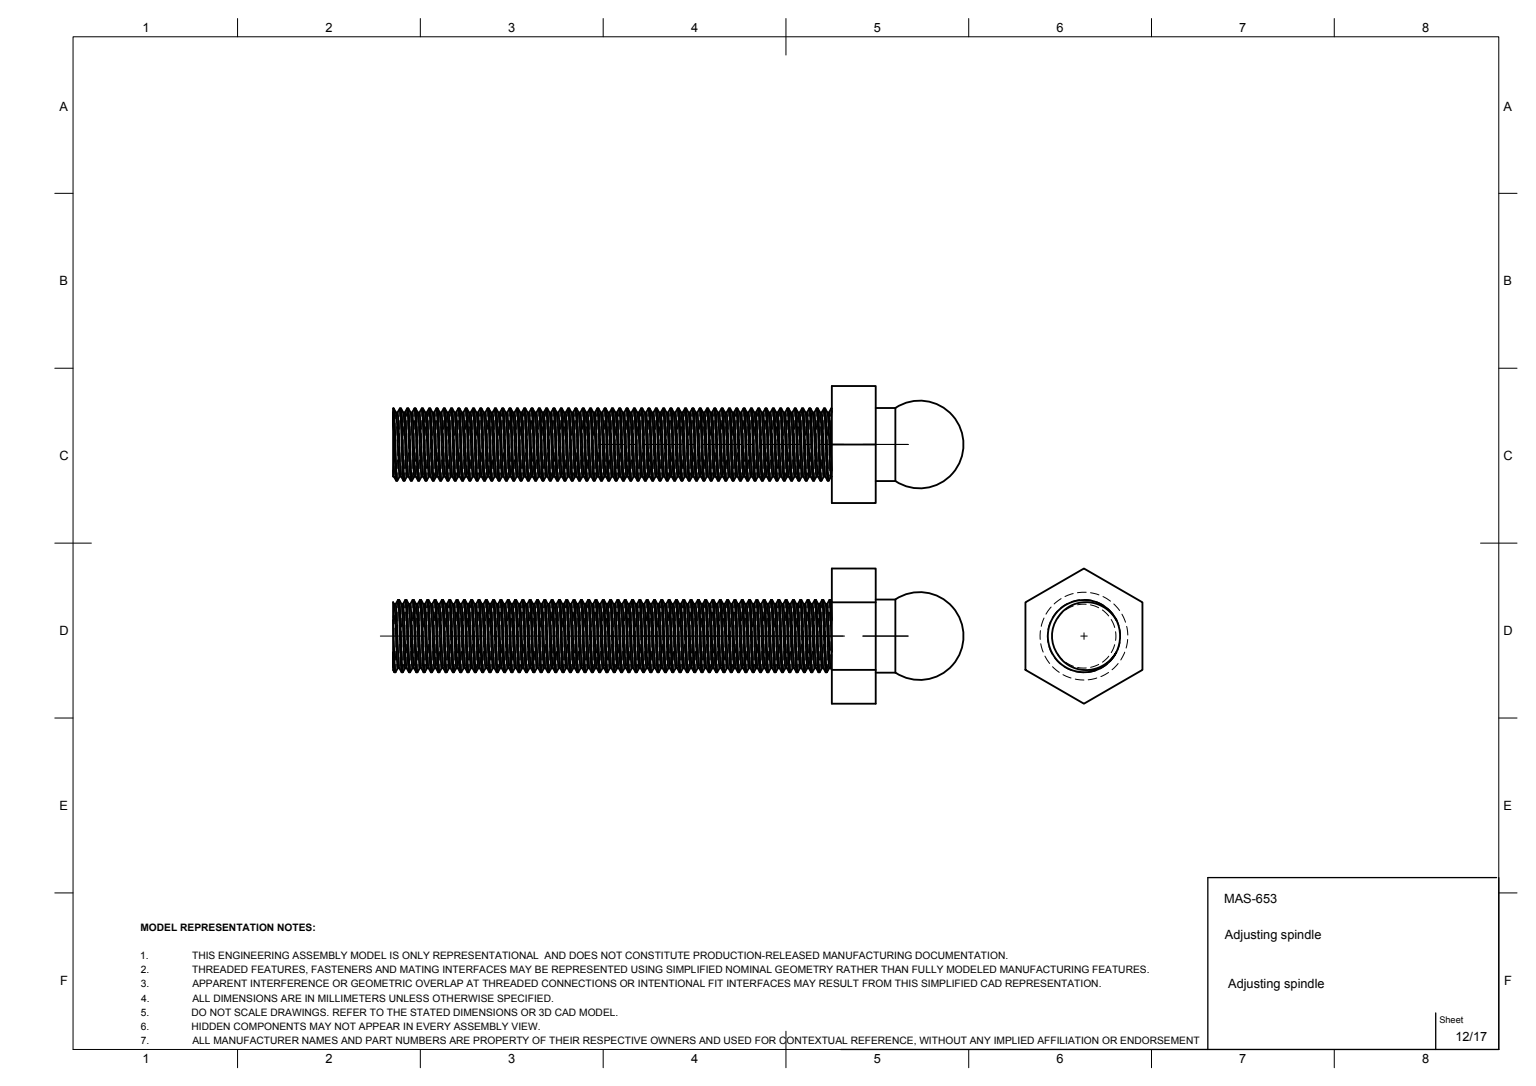
ISO-10303-21;
HEADER;
/* Generated by software containing ST-Developer
 * from STEP Tools, Inc. (www.steptools.com) 
 */

FILE_DESCRIPTION(
/* description */ ('Independent compact industrial fixture table, bolted aluminum worktop
 on connected adjustable support base. Whole-mm nominal dimensions. No
 load rating assigned.'),
/* implementation_level */ '2;1');

FILE_NAME(
/* name */ 'Adjusting spindle.step',
/* time_stamp */ '2026-11-07T17:47:58-08:00',
/* author */ (''),
/* organization */ (''),
/* preprocessor_version */ 'ST-DEVELOPER v20.2',
/* originating_system */ 'Autodesk Translation Framework v15.17.0.0',
/* authorisation */ '');

FILE_SCHEMA (('AUTOMOTIVE_DESIGN { 1 0 10303 214 3 1 1 }'));
ENDSEC;

DATA;
#10=MECHANICAL_DESIGN_GEOMETRIC_PRESENTATION_REPRESENTATION('',(#2261),#97475);
#13=SPHERICAL_SURFACE('',#22948,6.);
#356=B_SPLINE_SURFACE_WITH_KNOTS('',3,3,((#65272,#65273,#65274,#65275,#65276,
#65277,#65278,#65279,#65280,#65281,#65282,#65283,#65284,#65285,#65286,#65287,
#65288,#65289,#65290,#65291,#65292,#65293,#65294,#65295,#65296,#65297,#65298,
#65299,#65300,#65301,#65302,#65303,#65304,#65305,#65306,#65307,#65308,#65309,
#65310,#65311,#65312,#65313,#65314,#65315,#65316,#65317,#65318,#65319,#65320,
#65321,#65322,#65323,#65324,#65325,#65326,#65327,#65328,#65329,#65330,#65331,
#65332,#65333,#65334,#65335,#65336,#65337,#65338,#65339,#65340,#65341,#65342,
#65343,#65344,#65345,#65346,#65347,#65348,#65349,#65350,#65351,#65352,#65353,
#65354,#65355,#65356,#65357,#65358,#65359,#65360,#65361,#65362,#65363,#65364,
#65365,#65366,#65367,#65368,#65369,#65370,#65371,#65372,#65373,#65374,#65375,
#65376,#65377,#65378,#65379,#65380,#65381,#65382,#65383,#65384,#65385,#65386,
#65387,#65388,#65389,#65390,#65391,#65392,#65393,#65394,#65395,#65396,#65397,
#65398,#65399,#65400,#65401,#65402,#65403,#65404,#65405,#65406,#65407,#65408,
#65409,#65410,#65411,#65412,#65413,#65414,#65415,#65416,#65417,#65418,#65419,
#65420,#65421,#65422,#65423,#65424,#65425,#65426,#65427,#65428,#65429,#65430,
#65431,#65432,#65433,#65434,#65435,#65436,#65437,#65438,#65439,#65440,#65441,
#65442,#65443,#65444,#65445,#65446,#65447,#65448,#65449,#65450,#65451,#65452,
#65453,#65454,#65455,#65456,#65457,#65458,#65459,#65460,#65461,#65462,#65463,
#65464,#65465,#65466,#65467,#65468,#65469,#65470,#65471,#65472,#65473,#65474,
#65475,#65476,#65477,#65478,#65479,#65480,#65481,#65482,#65483,#65484,#65485,
#65486,#65487,#65488,#65489,#65490,#65491,#65492,#65493,#65494,#65495,#65496,
#65497,#65498,#65499,#65500,#65501,#65502,#65503,#65504,#65505,#65506,#65507,
#65508,#65509,#65510,#65511,#65512,#65513,#65514,#65515,#65516,#65517,#65518,
#65519,#65520,#65521,#65522,#65523,#65524,#65525,#65526,#65527,#65528,#65529,
#65530,#65531,#65532,#65533,#65534,#65535,#65536,#65537,#65538,#65539,#65540,
#65541,#65542,#65543,#65544,#65545,#65546,#65547,#65548,#65549,#65550,#65551,
#65552,#65553,#65554,#65555,#65556,#65557,#65558,#65559,#65560,#65561,#65562,
#65563,#65564,#65565,#65566,#65567,#65568,#65569,#65570,#65571,#65572,#65573,
#65574,#65575,#65576,#65577,#65578,#65579,#65580,#65581,#65582,#65583,#65584,
#65585,#65586,#65587,#65588,#65589,#65590,#65591,#65592,#65593,#65594,#65595,
#65596,#65597,#65598,#65599,#65600,#65601,#65602,#65603,#65604,#65605,#65606,
#65607,#65608,#65609,#65610,#65611,#65612,#65613,#65614,#65615,#65616,#65617,
#65618,#65619,#65620,#65621,#65622,#65623,#65624,#65625,#65626,#65627,#65628,
#65629,#65630,#65631,#65632,#65633,#65634,#65635,#65636,#65637,#65638,#65639,
#65640,#65641,#65642,#65643,#65644,#65645,#65646,#65647,#65648,#65649,#65650,
#65651,#65652,#65653,#65654,#65655,#65656),(#65657,#65658,#65659,#65660,
#65661,#65662,#65663,#65664,#65665,#65666,#65667,#65668,#65669,#65670,#65671,
#65672,#65673,#65674,#65675,#65676,#65677,#65678,#65679,#65680,#65681,#65682,
#65683,#65684,#65685,#65686,#65687,#65688,#65689,#65690,#65691,#65692,#65693,
#65694,#65695,#65696,#65697,#65698,#65699,#65700,#65701,#65702,#65703,#65704,
#65705,#65706,#65707,#65708,#65709,#65710,#65711,#65712,#65713,#65714,#65715,
#65716,#65717,#65718,#65719,#65720,#65721,#65722,#65723,#65724,#65725,#65726,
#65727,#65728,#65729,#65730,#65731,#65732,#65733,#65734,#65735,#65736,#65737,
#65738,#65739,#65740,#65741,#65742,#65743,#65744,#65745,#65746,#65747,#65748,
#65749,#65750,#65751,#65752,#65753,#65754,#65755,#65756,#65757,#65758,#65759,
#65760,#65761,#65762,#65763,#65764,#65765,#65766,#65767,#65768,#65769,#65770,
#65771,#65772,#65773,#65774,#65775,#65776,#65777,#65778,#65779,#65780,#65781,
#65782,#65783,#65784,#65785,#65786,#65787,#65788,#65789,#65790,#65791,#65792,
#65793,#65794,#65795,#65796,#65797,#65798,#65799,#65800,#65801,#65802,#65803,
#65804,#65805,#65806,#65807,#65808,#65809,#65810,#65811,#65812,#65813,#65814,
#65815,#65816,#65817,#65818,#65819,#65820,#65821,#65822,#65823,#65824,#65825,
#65826,#65827,#65828,#65829,#65830,#65831,#65832,#65833,#65834,#65835,#65836,
#65837,#65838,#65839,#65840,#65841,#65842,#65843,#65844,#65845,#65846,#65847,
#65848,#65849,#65850,#65851,#65852,#65853,#65854,#65855,#65856,#65857,#65858,
#65859,#65860,#65861,#65862,#65863,#65864,#65865,#65866,#65867,#65868,#65869,
#65870,#65871,#65872,#65873,#65874,#65875,#65876,#65877,#65878,#65879,#65880,
#65881,#65882,#65883,#65884,#65885,#65886,#65887,#65888,#65889,#65890,#65891,
#65892,#65893,#65894,#65895,#65896,#65897,#65898,#65899,#65900,#65901,#65902,
#65903,#65904,#65905,#65906,#65907,#65908,#65909,#65910,#65911,#65912,#65913,
#65914,#65915,#65916,#65917,#65918,#65919,#65920,#65921,#65922,#65923,#65924,
#65925,#65926,#65927,#65928,#65929,#65930,#65931,#65932,#65933,#65934,#65935,
#65936,#65937,#65938,#65939,#65940,#65941,#65942,#65943,#65944,#65945,#65946,
#65947,#65948,#65949,#65950,#65951,#65952,#65953,#65954,#65955,#65956,#65957,
#65958,#65959,#65960,#65961,#65962,#65963,#65964,#65965,#65966,#65967,#65968,
#65969,#65970,#65971,#65972,#65973,#65974,#65975,#65976,#65977,#65978,#65979,
#65980,#65981,#65982,#65983,#65984,#65985,#65986,#65987,#65988,#65989,#65990,
#65991,#65992,#65993,#65994,#65995,#65996,#65997,#65998,#65999,#66000,#66001,
#66002,#66003,#66004,#66005,#66006,#66007,#66008,#66009,#66010,#66011,#66012,
#66013,#66014,#66015,#66016,#66017,#66018,#66019,#66020,#66021,#66022,#66023,
#66024,#66025,#66026,#66027,#66028,#66029,#66030,#66031,#66032,#66033,#66034,
#66035,#66036,#66037,#66038,#66039,#66040,#66041),(#66042,#66043,#66044,
#66045,#66046,#66047,#66048,#66049,#66050,#66051,#66052,#66053,#66054,#66055,
#66056,#66057,#66058,#66059,#66060,#66061,#66062,#66063,#66064,#66065,#66066,
#66067,#66068,#66069,#66070,#66071,#66072,#66073,#66074,#66075,#66076,#66077,
#66078,#66079,#66080,#66081,#66082,#66083,#66084,#66085,#66086,#66087,#66088,
#66089,#66090,#66091,#66092,#66093,#66094,#66095,#66096,#66097,#66098,#66099,
#66100,#66101,#66102,#66103,#66104,#66105,#66106,#66107,#66108,#66109,#66110,
#66111,#66112,#66113,#66114,#66115,#66116,#66117,#66118,#66119,#66120,#66121,
#66122,#66123,#66124,#66125,#66126,#66127,#66128,#66129,#66130,#66131,#66132,
#66133,#66134,#66135,#66136,#66137,#66138,#66139,#66140,#66141,#66142,#66143,
#66144,#66145,#66146,#66147,#66148,#66149,#66150,#66151,#66152,#66153,#66154,
#66155,#66156,#66157,#66158,#66159,#66160,#66161,#66162,#66163,#66164,#66165,
#66166,#66167,#66168,#66169,#66170,#66171,#66172,#66173,#66174,#66175,#66176,
#66177,#66178,#66179,#66180,#66181,#66182,#66183,#66184,#66185,#66186,#66187,
#66188,#66189,#66190,#66191,#66192,#66193,#66194,#66195,#66196,#66197,#66198,
#66199,#66200,#66201,#66202,#66203,#66204,#66205,#66206,#66207,#66208,#66209,
#66210,#66211,#66212,#66213,#66214,#66215,#66216,#66217,#66218,#66219,#66220,
#66221,#66222,#66223,#66224,#66225,#66226,#66227,#66228,#66229,#66230,#66231,
#66232,#66233,#66234,#66235,#66236,#66237,#66238,#66239,#66240,#66241,#66242,
#66243,#66244,#66245,#66246,#66247,#66248,#66249,#66250,#66251,#66252,#66253,
#66254,#66255,#66256,#66257,#66258,#66259,#66260,#66261,#66262,#66263,#66264,
#66265,#66266,#66267,#66268,#66269,#66270,#66271,#66272,#66273,#66274,#66275,
#66276,#66277,#66278,#66279,#66280,#66281,#66282,#66283,#66284,#66285,#66286,
#66287,#66288,#66289,#66290,#66291,#66292,#66293,#66294,#66295,#66296,#66297,
#66298,#66299,#66300,#66301,#66302,#66303,#66304,#66305,#66306,#66307,#66308,
#66309,#66310,#66311,#66312,#66313,#66314,#66315,#66316,#66317,#66318,#66319,
#66320,#66321,#66322,#66323,#66324,#66325,#66326,#66327,#66328,#66329,#66330,
#66331,#66332,#66333,#66334,#66335,#66336,#66337,#66338,#66339,#66340,#66341,
#66342,#66343,#66344,#66345,#66346,#66347,#66348,#66349,#66350,#66351,#66352,
#66353,#66354,#66355,#66356,#66357,#66358,#66359,#66360,#66361,#66362,#66363,
#66364,#66365,#66366,#66367,#66368,#66369,#66370,#66371,#66372,#66373,#66374,
#66375,#66376,#66377,#66378,#66379,#66380,#66381,#66382,#66383,#66384,#66385,
#66386,#66387,#66388,#66389,#66390,#66391,#66392,#66393,#66394,#66395,#66396,
#66397,#66398,#66399,#66400,#66401,#66402,#66403,#66404,#66405,#66406,#66407,
#66408,#66409,#66410,#66411,#66412,#66413,#66414,#66415,#66416,#66417,#66418,
#66419,#66420,#66421,#66422,#66423,#66424,#66425,#66426),(#66427,#66428,
#66429,#66430,#66431,#66432,#66433,#66434,#66435,#66436,#66437,#66438,#66439,
#66440,#66441,#66442,#66443,#66444,#66445,#66446,#66447,#66448,#66449,#66450,
#66451,#66452,#66453,#66454,#66455,#66456,#66457,#66458,#66459,#66460,#66461,
#66462,#66463,#66464,#66465,#66466,#66467,#66468,#66469,#66470,#66471,#66472,
#66473,#66474,#66475,#66476,#66477,#66478,#66479,#66480,#66481,#66482,#66483,
#66484,#66485,#66486,#66487,#66488,#66489,#66490,#66491,#66492,#66493,#66494,
#66495,#66496,#66497,#66498,#66499,#66500,#66501,#66502,#66503,#66504,#66505,
#66506,#66507,#66508,#66509,#66510,#66511,#66512,#66513,#66514,#66515,#66516,
#66517,#66518,#66519,#66520,#66521,#66522,#66523,#66524,#66525,#66526,#66527,
#66528,#66529,#66530,#66531,#66532,#66533,#66534,#66535,#66536,#66537,#66538,
#66539,#66540,#66541,#66542,#66543,#66544,#66545,#66546,#66547,#66548,#66549,
#66550,#66551,#66552,#66553,#66554,#66555,#66556,#66557,#66558,#66559,#66560,
#66561,#66562,#66563,#66564,#66565,#66566,#66567,#66568,#66569,#66570,#66571,
#66572,#66573,#66574,#66575,#66576,#66577,#66578,#66579,#66580,#66581,#66582,
#66583,#66584,#66585,#66586,#66587,#66588,#66589,#66590,#66591,#66592,#66593,
#66594,#66595,#66596,#66597,#66598,#66599,#66600,#66601,#66602,#66603,#66604,
#66605,#66606,#66607,#66608,#66609,#66610,#66611,#66612,#66613,#66614,#66615,
#66616,#66617,#66618,#66619,#66620,#66621,#66622,#66623,#66624,#66625,#66626,
#66627,#66628,#66629,#66630,#66631,#66632,#66633,#66634,#66635,#66636,#66637,
#66638,#66639,#66640,#66641,#66642,#66643,#66644,#66645,#66646,#66647,#66648,
#66649,#66650,#66651,#66652,#66653,#66654,#66655,#66656,#66657,#66658,#66659,
#66660,#66661,#66662,#66663,#66664,#66665,#66666,#66667,#66668,#66669,#66670,
#66671,#66672,#66673,#66674,#66675,#66676,#66677,#66678,#66679,#66680,#66681,
#66682,#66683,#66684,#66685,#66686,#66687,#66688,#66689,#66690,#66691,#66692,
#66693,#66694,#66695,#66696,#66697,#66698,#66699,#66700,#66701,#66702,#66703,
#66704,#66705,#66706,#66707,#66708,#66709,#66710,#66711,#66712,#66713,#66714,
#66715,#66716,#66717,#66718,#66719,#66720,#66721,#66722,#66723,#66724,#66725,
#66726,#66727,#66728,#66729,#66730,#66731,#66732,#66733,#66734,#66735,#66736,
#66737,#66738,#66739,#66740,#66741,#66742,#66743,#66744,#66745,#66746,#66747,
#66748,#66749,#66750,#66751,#66752,#66753,#66754,#66755,#66756,#66757,#66758,
#66759,#66760,#66761,#66762,#66763,#66764,#66765,#66766,#66767,#66768,#66769,
#66770,#66771,#66772,#66773,#66774,#66775,#66776,#66777,#66778,#66779,#66780,
#66781,#66782,#66783,#66784,#66785,#66786,#66787,#66788,#66789,#66790,#66791,
#66792,#66793,#66794,#66795,#66796,#66797,#66798,#66799,#66800,#66801,#66802,
#66803,#66804,#66805,#66806,#66807,#66808,#66809,#66810,#66811)),
 .UNSPECIFIED.,.F.,.F.,.F.,(4,4),(4,1,1,1,1,1,1,1,1,1,1,1,1,1,1,1,1,1,1,
1,1,1,1,1,1,1,1,1,1,1,1,1,1,1,1,1,1,1,1,1,1,1,1,1,1,1,1,1,1,1,1,1,1,1,1,
1,1,1,1,1,1,1,1,1,1,1,1,1,1,1,1,1,1,1,1,1,1,1,1,1,1,1,1,1,1,1,1,1,1,1,1,
1,1,1,1,1,1,1,1,1,1,1,1,1,1,1,1,1,1,1,1,1,1,1,1,1,1,1,1,1,1,1,1,1,1,1,1,
1,1,1,1,1,1,1,1,1,1,1,1,1,1,1,1,1,1,1,1,1,1,1,1,1,1,1,1,1,1,1,1,1,1,1,1,
1,1,1,1,1,1,1,1,1,1,1,1,1,1,1,1,1,1,1,1,1,1,1,1,1,1,1,1,1,1,1,1,1,1,1,1,
1,1,1,1,1,1,1,1,1,1,1,1,1,1,1,1,1,1,1,1,1,1,1,1,1,1,1,1,1,1,1,1,1,1,1,1,
1,1,1,1,1,1,1,1,1,1,1,1,1,1,1,1,1,1,1,1,1,1,1,1,1,1,1,1,1,1,1,1,1,1,1,1,
1,1,1,1,1,1,1,1,1,1,1,1,1,1,1,1,1,1,1,1,1,1,1,1,1,1,1,1,1,1,1,1,1,1,1,1,
1,1,1,1,1,1,1,1,1,1,1,1,1,1,1,1,1,1,1,1,1,1,1,1,1,1,1,1,1,1,1,1,1,1,1,1,
1,1,1,1,1,1,1,1,1,1,1,1,1,1,1,1,1,1,1,1,1,1,1,1,1,1,1,1,1,1,1,1,1,1,1,1,
1,1,1,4),(0.,0.0658179306876174),(8.30838445208392,8.80714609643392,9.30590774078392,
10.3034310294839,11.3009543181839,12.2984776068839,13.2960008955839,14.2935241842839,
15.291047472984,16.288570761684,17.286094050384,18.283617339084,19.281140627784,
20.278663916484,21.276187205184,22.273710493884,23.271233782584,24.268757071284,
25.266280359984,26.263803648684,27.261326937384,28.258850226084,29.256373514784,
30.253896803484,31.251420092184,32.2489433808841,33.2464666695841,34.2439899582841,
35.2415132469841,36.2390365356841,37.2365598243841,38.2340831130841,39.2316064017841,
40.2291296904841,41.2266529791841,42.2241762678841,43.2216995565841,44.2192228452841,
45.2167461339841,46.2142694226841,47.2117927113841,48.2093160000841,49.2068392887841,
50.2043625774841,51.2018858661842,52.1994091548842,53.1969324435842,54.1944557322842,
55.1919790209842,56.1895023096842,57.1870255983842,58.1845488870842,59.1820721757842,
60.1795954644842,61.1771187531842,62.1746420418842,63.1721653305842,64.1696886192842,
65.1672119079842,66.1647351966842,67.1622584853842,68.1597817740843,69.1573050627842,
70.1548283514843,71.1523516401843,72.1498749288843,73.1473982175843,74.1449215062843,
75.1424447949843,76.1399680836843,77.1374913723843,78.1350146610843,79.1325379497843,
80.1300612384843,81.1275845271843,82.1251078158843,83.1226311045843,84.1201543932843,
85.1176776819843,86.1152009706843,87.1127242593844,88.1102475480844,89.1077708367844,
90.1052941254844,91.1028174141844,92.1003407028844,93.0978639915844,94.0953872802844,
95.0929105689844,96.0904338576844,97.0879571463844,98.0854804350844,99.0830037237844,
100.080527012484,101.078050301184,102.075573589884,103.073096878584,104.070620167284,
105.068143455984,106.065666744684,107.063190033384,108.060713322084,109.058236610784,
110.055759899484,111.053283188184,112.050806476884,113.048329765584,114.045853054284,
115.043376342985,116.040899631685,117.038422920385,118.035946209085,119.033469497785,
120.030992786485,121.028516075185,122.026039363885,123.023562652585,124.021085941285,
125.018609229985,126.016132518685,127.013655807385,128.011179096085,129.008702384785,
130.006225673485,131.003748962185,132.001272250885,132.998795539585,133.996318828285,
134.993842116985,135.991365405685,136.988888694385,137.986411983085,138.983935271785,
139.981458560485,140.978981849185,141.976505137885,142.974028426585,143.971551715285,
144.969075003985,145.966598292685,146.964121581385,147.961644870085,148.959168158785,
149.956691447485,150.954214736185,151.951738024885,152.949261313585,153.946784602285,
154.944307890985,155.941831179685,156.939354468385,157.936877757085,158.934401045785,
159.931924334485,160.929447623185,161.926970911885,162.924494200585,163.922017489285,
164.919540777985,165.917064066685,166.914587355385,167.912110644085,168.909633932785,
169.907157221485,170.904680510185,171.902203798885,172.899727087585,173.897250376285,
174.894773664985,175.892296953685,176.889820242385,177.887343531085,178.884866819785,
179.882390108485,180.879913397185,181.877436685885,182.874959974585,183.872483263285,
184.870006551985,185.867529840685,186.865053129385,187.862576418085,188.860099706785,
189.857622995485,190.855146284185,191.852669572885,192.850192861585,193.847716150285,
194.845239438985,195.842762727685,196.840286016385,197.837809305085,198.835332593785,
199.832855882485,200.830379171185,201.827902459885,202.825425748585,203.822949037285,
204.820472325985,205.817995614685,206.815518903385,207.813042192085,208.810565480785,
209.808088769485,210.805612058185,211.803135346885,212.800658635585,213.798181924285,
214.795705212985,215.793228501685,216.790751790385,217.788275079085,218.785798367785,
219.783321656485,220.780844945185,221.778368233885,222.775891522585,223.773414811285,
224.770938099985,225.768461388685,226.765984677385,227.763507966085,228.761031254785,
229.758554543485,230.756077832185,231.753601120885,232.751124409585,233.748647698285,
234.746170986985,235.743694275685,236.741217564385,237.738740853085,238.736264141785,
239.733787430485,240.731310719185,241.728834007885,242.726357296585,243.723880585285,
244.721403873985,245.718927162685,246.716450451385,247.713973740085,248.711497028785,
249.709020317485,250.706543606185,251.704066894885,252.701590183585,253.699113472285,
254.696636760985,255.694160049685,256.691683338385,257.689206627085,258.686729915785,
259.684253204485,260.681776493185,261.679299781885,262.676823070585,263.674346359285,
264.671869647985,265.669392936685,266.666916225385,267.664439514085,268.661962802785,
269.659486091485,270.657009380185,271.654532668885,272.652055957585,273.649579246285,
274.647102534985,275.644625823685,276.642149112385,277.639672401085,278.637195689785,
279.634718978485,280.632242267185,281.629765555885,282.627288844585,283.624812133285,
284.622335421985,285.619858710685,286.617381999385,287.614905288085,288.612428576785,
289.609951865485,290.607475154186,291.604998442886,292.602521731586,293.600045020286,
294.597568308986,295.595091597686,296.592614886386,297.590138175086,298.587661463786,
299.585184752486,300.582708041186,301.580231329886,302.577754618586,303.575277907286,
304.572801195986,305.570324484686,306.567847773386,307.565371062086,308.562894350786,
309.560417639486,310.557940928186,311.555464216886,312.552987505586,313.550510794286,
314.548034082986,315.545557371686,316.543080660386,317.540603949086,318.538127237786,
319.535650526486,320.533173815186,321.530697103886,322.528220392586,323.525743681286,
324.523266969986,325.520790258686,326.518313547386,327.515836836086,328.513360124786,
329.510883413486,330.508406702186,331.505929990886,332.503453279586,333.500976568286,
334.498499856986,335.496023145686,336.493546434386,337.491069723086,338.488593011786,
339.486116300486,340.483639589186,341.481162877886,342.478686166586,343.476209455286,
344.473732743986,345.471256032686,346.468779321386,347.466302610086,348.463825898786,
349.461349187486,350.458872476186,351.456395764886,352.453919053586,353.451442342286,
354.448965630986,355.446488919686,356.444012208386,357.441535497086,358.439058785786,
359.436582074486,360.434105363186,361.431628651886,362.429151940586,363.426675229286,
364.424198517986,365.421721806686,366.419245095386,367.416768384086,368.414291672786,
369.411814961486,370.409338250186,371.406861538886,372.404384827586,373.401908116286,
374.399431404986,375.396954693686,376.394477982386,377.392001271086,378.389524559786,
379.387047848486,380.384571137186,381.382094425886,382.379617714586,383.377141003286,
384.374664291986,385.372187580686,386.369710869386,386.868472513736,387.367234158086),
 .UNSPECIFIED.);
#357=B_SPLINE_SURFACE_WITH_KNOTS('',3,3,((#67069,#67070,#67071,#67072,#67073,
#67074,#67075,#67076,#67077,#67078,#67079,#67080,#67081,#67082,#67083,#67084,
#67085,#67086,#67087,#67088,#67089,#67090,#67091,#67092,#67093,#67094,#67095,
#67096,#67097,#67098,#67099,#67100,#67101,#67102,#67103,#67104,#67105,#67106,
#67107,#67108,#67109,#67110,#67111,#67112,#67113,#67114,#67115,#67116,#67117,
#67118,#67119,#67120,#67121,#67122,#67123,#67124,#67125,#67126,#67127,#67128,
#67129,#67130,#67131,#67132,#67133,#67134,#67135,#67136,#67137,#67138,#67139,
#67140,#67141,#67142,#67143,#67144,#67145,#67146,#67147,#67148,#67149,#67150,
#67151,#67152,#67153,#67154,#67155,#67156,#67157,#67158,#67159,#67160,#67161,
#67162,#67163,#67164,#67165,#67166,#67167,#67168,#67169,#67170,#67171,#67172,
#67173,#67174,#67175,#67176,#67177,#67178,#67179,#67180,#67181,#67182,#67183,
#67184,#67185,#67186,#67187,#67188,#67189,#67190,#67191,#67192,#67193,#67194,
#67195,#67196,#67197,#67198,#67199,#67200,#67201,#67202,#67203,#67204,#67205,
#67206,#67207,#67208,#67209,#67210,#67211,#67212,#67213,#67214,#67215,#67216,
#67217,#67218,#67219,#67220,#67221,#67222,#67223,#67224,#67225,#67226,#67227,
#67228,#67229,#67230,#67231,#67232,#67233,#67234,#67235,#67236,#67237,#67238,
#67239,#67240,#67241,#67242,#67243,#67244,#67245,#67246,#67247,#67248,#67249,
#67250,#67251,#67252,#67253,#67254,#67255,#67256,#67257,#67258,#67259,#67260,
#67261,#67262,#67263,#67264,#67265,#67266,#67267,#67268,#67269,#67270,#67271,
#67272,#67273,#67274,#67275,#67276,#67277,#67278,#67279,#67280,#67281,#67282,
#67283,#67284,#67285,#67286,#67287,#67288,#67289,#67290,#67291,#67292,#67293,
#67294,#67295,#67296,#67297,#67298,#67299,#67300,#67301,#67302,#67303,#67304,
#67305,#67306,#67307,#67308,#67309,#67310,#67311,#67312,#67313,#67314,#67315,
#67316,#67317,#67318,#67319,#67320,#67321,#67322,#67323,#67324,#67325,#67326,
#67327,#67328,#67329,#67330,#67331,#67332,#67333,#67334,#67335,#67336,#67337,
#67338,#67339,#67340,#67341,#67342,#67343,#67344,#67345,#67346,#67347,#67348,
#67349,#67350,#67351,#67352,#67353,#67354,#67355,#67356,#67357,#67358,#67359,
#67360,#67361,#67362,#67363,#67364,#67365,#67366,#67367,#67368,#67369,#67370,
#67371,#67372,#67373,#67374,#67375,#67376,#67377,#67378,#67379,#67380,#67381,
#67382,#67383,#67384,#67385,#67386,#67387,#67388,#67389,#67390,#67391,#67392,
#67393,#67394,#67395,#67396,#67397,#67398,#67399,#67400,#67401,#67402,#67403,
#67404,#67405,#67406,#67407,#67408,#67409,#67410,#67411,#67412,#67413,#67414,
#67415,#67416,#67417,#67418,#67419,#67420,#67421,#67422,#67423,#67424,#67425,
#67426,#67427,#67428,#67429,#67430,#67431,#67432,#67433,#67434,#67435,#67436,
#67437,#67438,#67439,#67440,#67441,#67442,#67443,#67444,#67445,#67446,#67447,
#67448,#67449,#67450,#67451,#67452,#67453),(#67454,#67455,#67456,#67457,
#67458,#67459,#67460,#67461,#67462,#67463,#67464,#67465,#67466,#67467,#67468,
#67469,#67470,#67471,#67472,#67473,#67474,#67475,#67476,#67477,#67478,#67479,
#67480,#67481,#67482,#67483,#67484,#67485,#67486,#67487,#67488,#67489,#67490,
#67491,#67492,#67493,#67494,#67495,#67496,#67497,#67498,#67499,#67500,#67501,
#67502,#67503,#67504,#67505,#67506,#67507,#67508,#67509,#67510,#67511,#67512,
#67513,#67514,#67515,#67516,#67517,#67518,#67519,#67520,#67521,#67522,#67523,
#67524,#67525,#67526,#67527,#67528,#67529,#67530,#67531,#67532,#67533,#67534,
#67535,#67536,#67537,#67538,#67539,#67540,#67541,#67542,#67543,#67544,#67545,
#67546,#67547,#67548,#67549,#67550,#67551,#67552,#67553,#67554,#67555,#67556,
#67557,#67558,#67559,#67560,#67561,#67562,#67563,#67564,#67565,#67566,#67567,
#67568,#67569,#67570,#67571,#67572,#67573,#67574,#67575,#67576,#67577,#67578,
#67579,#67580,#67581,#67582,#67583,#67584,#67585,#67586,#67587,#67588,#67589,
#67590,#67591,#67592,#67593,#67594,#67595,#67596,#67597,#67598,#67599,#67600,
#67601,#67602,#67603,#67604,#67605,#67606,#67607,#67608,#67609,#67610,#67611,
#67612,#67613,#67614,#67615,#67616,#67617,#67618,#67619,#67620,#67621,#67622,
#67623,#67624,#67625,#67626,#67627,#67628,#67629,#67630,#67631,#67632,#67633,
#67634,#67635,#67636,#67637,#67638,#67639,#67640,#67641,#67642,#67643,#67644,
#67645,#67646,#67647,#67648,#67649,#67650,#67651,#67652,#67653,#67654,#67655,
#67656,#67657,#67658,#67659,#67660,#67661,#67662,#67663,#67664,#67665,#67666,
#67667,#67668,#67669,#67670,#67671,#67672,#67673,#67674,#67675,#67676,#67677,
#67678,#67679,#67680,#67681,#67682,#67683,#67684,#67685,#67686,#67687,#67688,
#67689,#67690,#67691,#67692,#67693,#67694,#67695,#67696,#67697,#67698,#67699,
#67700,#67701,#67702,#67703,#67704,#67705,#67706,#67707,#67708,#67709,#67710,
#67711,#67712,#67713,#67714,#67715,#67716,#67717,#67718,#67719,#67720,#67721,
#67722,#67723,#67724,#67725,#67726,#67727,#67728,#67729,#67730,#67731,#67732,
#67733,#67734,#67735,#67736,#67737,#67738,#67739,#67740,#67741,#67742,#67743,
#67744,#67745,#67746,#67747,#67748,#67749,#67750,#67751,#67752,#67753,#67754,
#67755,#67756,#67757,#67758,#67759,#67760,#67761,#67762,#67763,#67764,#67765,
#67766,#67767,#67768,#67769,#67770,#67771,#67772,#67773,#67774,#67775,#67776,
#67777,#67778,#67779,#67780,#67781,#67782,#67783,#67784,#67785,#67786,#67787,
#67788,#67789,#67790,#67791,#67792,#67793,#67794,#67795,#67796,#67797,#67798,
#67799,#67800,#67801,#67802,#67803,#67804,#67805,#67806,#67807,#67808,#67809,
#67810,#67811,#67812,#67813,#67814,#67815,#67816,#67817,#67818,#67819,#67820,
#67821,#67822,#67823,#67824,#67825,#67826,#67827,#67828,#67829,#67830,#67831,
#67832,#67833,#67834,#67835,#67836,#67837,#67838),(#67839,#67840,#67841,
#67842,#67843,#67844,#67845,#67846,#67847,#67848,#67849,#67850,#67851,#67852,
#67853,#67854,#67855,#67856,#67857,#67858,#67859,#67860,#67861,#67862,#67863,
#67864,#67865,#67866,#67867,#67868,#67869,#67870,#67871,#67872,#67873,#67874,
#67875,#67876,#67877,#67878,#67879,#67880,#67881,#67882,#67883,#67884,#67885,
#67886,#67887,#67888,#67889,#67890,#67891,#67892,#67893,#67894,#67895,#67896,
#67897,#67898,#67899,#67900,#67901,#67902,#67903,#67904,#67905,#67906,#67907,
#67908,#67909,#67910,#67911,#67912,#67913,#67914,#67915,#67916,#67917,#67918,
#67919,#67920,#67921,#67922,#67923,#67924,#67925,#67926,#67927,#67928,#67929,
#67930,#67931,#67932,#67933,#67934,#67935,#67936,#67937,#67938,#67939,#67940,
#67941,#67942,#67943,#67944,#67945,#67946,#67947,#67948,#67949,#67950,#67951,
#67952,#67953,#67954,#67955,#67956,#67957,#67958,#67959,#67960,#67961,#67962,
#67963,#67964,#67965,#67966,#67967,#67968,#67969,#67970,#67971,#67972,#67973,
#67974,#67975,#67976,#67977,#67978,#67979,#67980,#67981,#67982,#67983,#67984,
#67985,#67986,#67987,#67988,#67989,#67990,#67991,#67992,#67993,#67994,#67995,
#67996,#67997,#67998,#67999,#68000,#68001,#68002,#68003,#68004,#68005,#68006,
#68007,#68008,#68009,#68010,#68011,#68012,#68013,#68014,#68015,#68016,#68017,
#68018,#68019,#68020,#68021,#68022,#68023,#68024,#68025,#68026,#68027,#68028,
#68029,#68030,#68031,#68032,#68033,#68034,#68035,#68036,#68037,#68038,#68039,
#68040,#68041,#68042,#68043,#68044,#68045,#68046,#68047,#68048,#68049,#68050,
#68051,#68052,#68053,#68054,#68055,#68056,#68057,#68058,#68059,#68060,#68061,
#68062,#68063,#68064,#68065,#68066,#68067,#68068,#68069,#68070,#68071,#68072,
#68073,#68074,#68075,#68076,#68077,#68078,#68079,#68080,#68081,#68082,#68083,
#68084,#68085,#68086,#68087,#68088,#68089,#68090,#68091,#68092,#68093,#68094,
#68095,#68096,#68097,#68098,#68099,#68100,#68101,#68102,#68103,#68104,#68105,
#68106,#68107,#68108,#68109,#68110,#68111,#68112,#68113,#68114,#68115,#68116,
#68117,#68118,#68119,#68120,#68121,#68122,#68123,#68124,#68125,#68126,#68127,
#68128,#68129,#68130,#68131,#68132,#68133,#68134,#68135,#68136,#68137,#68138,
#68139,#68140,#68141,#68142,#68143,#68144,#68145,#68146,#68147,#68148,#68149,
#68150,#68151,#68152,#68153,#68154,#68155,#68156,#68157,#68158,#68159,#68160,
#68161,#68162,#68163,#68164,#68165,#68166,#68167,#68168,#68169,#68170,#68171,
#68172,#68173,#68174,#68175,#68176,#68177,#68178,#68179,#68180,#68181,#68182,
#68183,#68184,#68185,#68186,#68187,#68188,#68189,#68190,#68191,#68192,#68193,
#68194,#68195,#68196,#68197,#68198,#68199,#68200,#68201,#68202,#68203,#68204,
#68205,#68206,#68207,#68208,#68209,#68210,#68211,#68212,#68213,#68214,#68215,
#68216,#68217,#68218,#68219,#68220,#68221,#68222,#68223),(#68224,#68225,
#68226,#68227,#68228,#68229,#68230,#68231,#68232,#68233,#68234,#68235,#68236,
#68237,#68238,#68239,#68240,#68241,#68242,#68243,#68244,#68245,#68246,#68247,
#68248,#68249,#68250,#68251,#68252,#68253,#68254,#68255,#68256,#68257,#68258,
#68259,#68260,#68261,#68262,#68263,#68264,#68265,#68266,#68267,#68268,#68269,
#68270,#68271,#68272,#68273,#68274,#68275,#68276,#68277,#68278,#68279,#68280,
#68281,#68282,#68283,#68284,#68285,#68286,#68287,#68288,#68289,#68290,#68291,
#68292,#68293,#68294,#68295,#68296,#68297,#68298,#68299,#68300,#68301,#68302,
#68303,#68304,#68305,#68306,#68307,#68308,#68309,#68310,#68311,#68312,#68313,
#68314,#68315,#68316,#68317,#68318,#68319,#68320,#68321,#68322,#68323,#68324,
#68325,#68326,#68327,#68328,#68329,#68330,#68331,#68332,#68333,#68334,#68335,
#68336,#68337,#68338,#68339,#68340,#68341,#68342,#68343,#68344,#68345,#68346,
#68347,#68348,#68349,#68350,#68351,#68352,#68353,#68354,#68355,#68356,#68357,
#68358,#68359,#68360,#68361,#68362,#68363,#68364,#68365,#68366,#68367,#68368,
#68369,#68370,#68371,#68372,#68373,#68374,#68375,#68376,#68377,#68378,#68379,
#68380,#68381,#68382,#68383,#68384,#68385,#68386,#68387,#68388,#68389,#68390,
#68391,#68392,#68393,#68394,#68395,#68396,#68397,#68398,#68399,#68400,#68401,
#68402,#68403,#68404,#68405,#68406,#68407,#68408,#68409,#68410,#68411,#68412,
#68413,#68414,#68415,#68416,#68417,#68418,#68419,#68420,#68421,#68422,#68423,
#68424,#68425,#68426,#68427,#68428,#68429,#68430,#68431,#68432,#68433,#68434,
#68435,#68436,#68437,#68438,#68439,#68440,#68441,#68442,#68443,#68444,#68445,
#68446,#68447,#68448,#68449,#68450,#68451,#68452,#68453,#68454,#68455,#68456,
#68457,#68458,#68459,#68460,#68461,#68462,#68463,#68464,#68465,#68466,#68467,
#68468,#68469,#68470,#68471,#68472,#68473,#68474,#68475,#68476,#68477,#68478,
#68479,#68480,#68481,#68482,#68483,#68484,#68485,#68486,#68487,#68488,#68489,
#68490,#68491,#68492,#68493,#68494,#68495,#68496,#68497,#68498,#68499,#68500,
#68501,#68502,#68503,#68504,#68505,#68506,#68507,#68508,#68509,#68510,#68511,
#68512,#68513,#68514,#68515,#68516,#68517,#68518,#68519,#68520,#68521,#68522,
#68523,#68524,#68525,#68526,#68527,#68528,#68529,#68530,#68531,#68532,#68533,
#68534,#68535,#68536,#68537,#68538,#68539,#68540,#68541,#68542,#68543,#68544,
#68545,#68546,#68547,#68548,#68549,#68550,#68551,#68552,#68553,#68554,#68555,
#68556,#68557,#68558,#68559,#68560,#68561,#68562,#68563,#68564,#68565,#68566,
#68567,#68568,#68569,#68570,#68571,#68572,#68573,#68574,#68575,#68576,#68577,
#68578,#68579,#68580,#68581,#68582,#68583,#68584,#68585,#68586,#68587,#68588,
#68589,#68590,#68591,#68592,#68593,#68594,#68595,#68596,#68597,#68598,#68599,
#68600,#68601,#68602,#68603,#68604,#68605,#68606,#68607,#68608)),
 .UNSPECIFIED.,.F.,.F.,.F.,(4,4),(4,1,1,1,1,1,1,1,1,1,1,1,1,1,1,1,1,1,1,
1,1,1,1,1,1,1,1,1,1,1,1,1,1,1,1,1,1,1,1,1,1,1,1,1,1,1,1,1,1,1,1,1,1,1,1,
1,1,1,1,1,1,1,1,1,1,1,1,1,1,1,1,1,1,1,1,1,1,1,1,1,1,1,1,1,1,1,1,1,1,1,1,
1,1,1,1,1,1,1,1,1,1,1,1,1,1,1,1,1,1,1,1,1,1,1,1,1,1,1,1,1,1,1,1,1,1,1,1,
1,1,1,1,1,1,1,1,1,1,1,1,1,1,1,1,1,1,1,1,1,1,1,1,1,1,1,1,1,1,1,1,1,1,1,1,
1,1,1,1,1,1,1,1,1,1,1,1,1,1,1,1,1,1,1,1,1,1,1,1,1,1,1,1,1,1,1,1,1,1,1,1,
1,1,1,1,1,1,1,1,1,1,1,1,1,1,1,1,1,1,1,1,1,1,1,1,1,1,1,1,1,1,1,1,1,1,1,1,
1,1,1,1,1,1,1,1,1,1,1,1,1,1,1,1,1,1,1,1,1,1,1,1,1,1,1,1,1,1,1,1,1,1,1,1,
1,1,1,1,1,1,1,1,1,1,1,1,1,1,1,1,1,1,1,1,1,1,1,1,1,1,1,1,1,1,1,1,1,1,1,1,
1,1,1,1,1,1,1,1,1,1,1,1,1,1,1,1,1,1,1,1,1,1,1,1,1,1,1,1,1,1,1,1,1,1,1,1,
1,1,1,1,1,1,1,1,1,1,1,1,1,1,1,1,1,1,1,1,1,1,1,1,1,1,1,1,1,1,1,1,1,1,1,1,
1,1,1,4),(0.,0.0658179306876174),(11.6150328478191,12.1137944921691,12.6125561365191,
13.6100794252191,14.6076027139191,15.6051260026191,16.6026492913191,17.6001725800191,
18.5976958687191,19.5952191574192,20.5927424461192,21.5902657348192,22.5877890235192,
23.5853123122192,24.5828356009192,25.5803588896192,26.5778821783192,27.5754054670192,
28.5729287557192,29.5704520444192,30.5679753331192,31.5654986218192,32.5630219105192,
33.5605451992192,34.5580684879192,35.5555917766192,36.5531150653192,37.5506383540192,
38.5481616427193,39.5456849314193,40.5432082201193,41.5407315088193,42.5382547975193,
43.5357780862193,44.5333013749193,45.5308246636193,46.5283479523193,47.5258712410193,
48.5233945297193,49.5209178184193,50.5184411071193,51.5159643958193,52.5134876845193,
53.5110109732193,54.5085342619193,55.5060575506193,56.5035808393194,57.5011041280194,
58.4986274167194,59.4961507054194,60.4936739941194,61.4911972828194,62.4887205715194,
63.4862438602194,64.4837671489194,65.4812904376194,66.4788137263194,67.4763370150194,
68.4738603037194,69.4713835924194,70.4689068811194,71.4664301698194,72.4639534585194,
73.4614767472195,74.4590000359194,75.4565233246195,76.4540466133195,77.4515699020195,
78.4490931907195,79.4466164794195,80.4441397681195,81.4416630568195,82.4391863455195,
83.4367096342195,84.4342329229195,85.4317562116195,86.4292795003195,87.4268027890195,
88.4243260777195,89.4218493664195,90.4193726551195,91.4168959438195,92.4144192325195,
93.4119425212196,94.4094658099196,95.4069890986196,96.4045123873196,97.4020356760196,
98.3995589647196,99.3970822534196,100.39460554212,101.39212883082,102.38965211952,
103.38717540822,104.38469869692,105.38222198562,106.37974527432,107.37726856302,
108.37479185172,109.37231514042,110.36983842912,111.36736171782,112.36488500652,
113.36240829522,114.35993158392,115.35745487262,116.35497816132,117.35250145002,
118.35002473872,119.34754802742,120.34507131612,121.34259460482,122.34011789352,
123.33764118222,124.33516447092,125.33268775962,126.33021104832,127.32773433702,
128.32525762572,129.32278091442,130.32030420312,131.31782749182,132.31535078052,
133.31287406922,134.31039735792,135.30792064662,136.30544393532,137.30296722402,
138.30049051272,139.29801380142,140.29553709012,141.29306037882,142.29058366752,
143.28810695622,144.28563024492,145.28315353362,146.28067682232,147.27820011102,
148.27572339972,149.27324668842,150.27076997712,151.26829326582,152.26581655452,
153.26333984322,154.26086313192,155.25838642062,156.25590970932,157.25343299802,
158.25095628672,159.24847957542,160.24600286412,161.24352615282,162.24104944152,
163.23857273022,164.23609601892,165.23361930762,166.23114259632,167.22866588502,
168.22618917372,169.22371246242,170.22123575112,171.21875903982,172.21628232852,
173.21380561722,174.21132890592,175.20885219462,176.20637548332,177.20389877202,
178.20142206072,179.19894534942,180.19646863812,181.19399192682,182.19151521552,
183.18903850422,184.18656179292,185.18408508162,186.18160837032,187.17913165902,
188.17665494772,189.17417823642,190.17170152512,191.16922481382,192.16674810252,
193.16427139122,194.16179467992,195.15931796862,196.15684125732,197.15436454602,
198.15188783472,199.14941112342,200.14693441212,201.14445770082,202.14198098952,
203.13950427822,204.13702756692,205.13455085562,206.13207414432,207.12959743302,
208.12712072172,209.12464401042,210.12216729912,211.11969058782,212.11721387652,
213.11473716522,214.11226045392,215.10978374262,216.10730703132,217.10483032002,
218.10235360872,219.09987689742,220.09740018612,221.09492347482,222.09244676352,
223.08997005222,224.08749334092,225.08501662962,226.08253991832,227.08006320702,
228.07758649572,229.07510978442,230.07263307312,231.07015636182,232.06767965052,
233.06520293922,234.06272622792,235.06024951662,236.05777280532,237.05529609402,
238.05281938272,239.05034267142,240.04786596012,241.04538924882,242.04291253752,
243.04043582622,244.03795911492,245.03548240362,246.03300569232,247.03052898102,
248.02805226972,249.02557555842,250.02309884712,251.02062213582,252.01814542452,
253.01566871322,254.01319200192,255.01071529062,256.00823857932,257.00576186802,
258.00328515672,259.00080844542,259.99833173412,260.99585502282,261.99337831152,
262.99090160022,263.98842488892,264.98594817762,265.983471466321,266.980994755021,
267.97851804372,268.97604133242,269.973564621121,270.971087909821,271.968611198521,
272.966134487221,273.963657775921,274.961181064621,275.958704353321,276.956227642021,
277.953750930721,278.951274219421,279.948797508121,280.946320796821,281.943844085521,
282.941367374221,283.938890662921,284.936413951621,285.933937240321,286.931460529021,
287.928983817721,288.926507106421,289.924030395121,290.921553683821,291.919076972521,
292.916600261221,293.914123549921,294.911646838621,295.909170127321,296.906693416021,
297.904216704721,298.901739993421,299.899263282121,300.896786570821,301.894309859521,
302.891833148221,303.889356436921,304.886879725621,305.884403014321,306.881926303021,
307.879449591721,308.876972880421,309.874496169121,310.872019457821,311.869542746521,
312.867066035221,313.864589323921,314.862112612621,315.859635901321,316.857159190021,
317.854682478721,318.852205767421,319.849729056121,320.847252344821,321.844775633521,
322.842298922221,323.839822210921,324.837345499621,325.834868788321,326.832392077021,
327.829915365721,328.827438654421,329.824961943121,330.822485231821,331.820008520521,
332.817531809221,333.815055097921,334.812578386621,335.810101675321,336.807624964021,
337.805148252721,338.802671541421,339.800194830121,340.797718118821,341.795241407521,
342.792764696221,343.790287984921,344.787811273621,345.785334562321,346.782857851021,
347.780381139721,348.777904428421,349.775427717121,350.772951005821,351.770474294521,
352.767997583221,353.765520871921,354.763044160621,355.760567449321,356.758090738021,
357.755614026721,358.753137315421,359.750660604121,360.748183892821,361.745707181521,
362.743230470221,363.740753758921,364.738277047621,365.735800336321,366.733323625021,
367.730846913721,368.728370202421,369.725893491121,370.723416779821,371.720940068521,
372.718463357221,373.715986645921,374.713509934621,375.711033223321,376.708556512021,
377.706079800721,378.703603089421,379.701126378121,380.698649666821,381.696172955521,
382.693696244221,383.691219532921,384.688742821621,385.686266110321,386.683789399021,
387.681312687721,388.678835976421,389.676359265121,390.175120909471,390.673882553821),
 .UNSPECIFIED.);
#1122=B_SPLINE_CURVE_WITH_KNOTS('',3,(#60850,#60851,#60852,#60853,#60854,
#60855,#60856,#60857,#60858,#60859),.UNSPECIFIED.,.F.,.F.,(4,3,3,4),(-4.09293042013064,
-3.99009315480002,-2.99256986610002,-2.06773127522702),.UNSPECIFIED.);
#1123=B_SPLINE_CURVE_WITH_KNOTS('',3,(#60862,#60863,#60864,#60865,#60866,
#60867,#60868,#60869,#60870,#60871),.UNSPECIFIED.,.F.,.F.,(4,3,3,4),(0.,
0.49876164434999,0.997523288699981,1.11639350868703),.UNSPECIFIED.);
#1124=B_SPLINE_CURVE_WITH_KNOTS('',3,(#60876,#60877,#60878,#60879,#60880,
#60881,#60882,#60883,#60884,#60885,#60886,#60887,#60888,#60889,#60890,#60891,
#60892,#60893,#60894,#60895,#60896,#60897),.UNSPECIFIED.,.F.,.F.,(4,3,3,
3,3,3,3,4),(-10.3761157273102,-9.97523288700005,-8.97770959830005,-7.98018630960004,
-6.98266302090004,-5.98513973220003,-4.98761644350003,-4.09293042013064),
 .UNSPECIFIED.);
#1125=B_SPLINE_CURVE_WITH_KNOTS('',3,(#60898,#60899,#60900,#60901,#60902,
#60903,#60904,#60905,#60906,#60907,#60908,#60909,#60910,#60911,#60912,#60913,
#60914,#60915,#60916,#60917,#60918,#60919),.UNSPECIFIED.,.F.,.F.,(4,3,3,
3,3,3,3,4),(1.11639350868703,1.99504657739999,2.9925698661,3.9900931548,
4.98761644350001,5.98513973220002,6.98266302090003,7.39957881586659),
 .UNSPECIFIED.);
#1126=B_SPLINE_CURVE_WITH_KNOTS('',3,(#60924,#60925,#60926,#60927,#60928,
#60929,#60930,#60931,#60932,#60933,#60934,#60935,#60936,#60937,#60938,#60939,
#60940,#60941,#60942,#60943,#60944,#60945),.UNSPECIFIED.,.F.,.F.,(4,3,3,
3,3,3,3,4),(-16.6593010344898,-15.9603726192001,-14.9628493305001,-13.9653260418001,
-12.9678027531001,-11.9702794644001,-10.9727561757001,-10.3761157273102),
 .UNSPECIFIED.);
#1127=B_SPLINE_CURVE_WITH_KNOTS('',3,(#60946,#60947,#60948,#60949,#60950,
#60951,#60952,#60953,#60954,#60955,#60956,#60957,#60958,#60959,#60960,#60961,
#60962,#60963,#60964,#60965,#60966,#60967),.UNSPECIFIED.,.F.,.F.,(4,3,3,
3,3,3,3,4),(7.39957881586659,7.98018630960004,8.97770959830006,9.97523288700007,
10.9727561757001,11.9702794644001,12.9678027531001,13.6827641230462),
 .UNSPECIFIED.);
#1128=B_SPLINE_CURVE_WITH_KNOTS('',3,(#60972,#60973,#60974,#60975,#60976,
#60977,#60978,#60979,#60980,#60981,#60982,#60983,#60984,#60985,#60986,#60987,
#60988,#60989,#60990,#60991,#60992,#60993),.UNSPECIFIED.,.F.,.F.,(4,3,3,
3,3,3,3,4),(-22.9424863416694,-21.9455123514001,-20.9479890627001,-19.9504657740001,
-18.9529424853001,-17.9554191966001,-16.9578959079001,-16.6593010344898),
 .UNSPECIFIED.);
#1129=B_SPLINE_CURVE_WITH_KNOTS('',3,(#60994,#60995,#60996,#60997,#60998,
#60999,#61000,#61001,#61002,#61003,#61004,#61005,#61006,#61007,#61008,#61009,
#61010,#61011,#61012,#61013,#61014,#61015,#61016,#61017,#61018),
 .UNSPECIFIED.,.F.,.F.,(4,3,3,3,3,3,3,3,4),(13.6827641230462,13.9653260418001,
14.9628493305001,15.9603726192001,16.9578959079001,17.9554191966001,18.9529424853001,
19.9504657740001,19.9659494302258),.UNSPECIFIED.);
#1130=B_SPLINE_CURVE_WITH_KNOTS('',3,(#61023,#61024,#61025,#61026,#61027,
#61028,#61029,#61030,#61031,#61032,#61033,#61034,#61035,#61036,#61037,#61038,
#61039,#61040,#61041,#61042,#61043,#61044),.UNSPECIFIED.,.F.,.F.,(4,3,3,
3,3,3,3,4),(-29.225671648849,-28.9281753723002,-27.9306520836002,-26.9331287949001,
-25.9356055062001,-24.9380822175001,-23.9405589288001,-22.9424863416694),
 .UNSPECIFIED.);
#1131=B_SPLINE_CURVE_WITH_KNOTS('',3,(#61045,#61046,#61047,#61048,#61049,
#61050,#61051,#61052,#61053,#61054,#61055,#61056,#61057,#61058,#61059,#61060,
#61061,#61062,#61063,#61064,#61065,#61066),.UNSPECIFIED.,.F.,.F.,(4,3,3,
3,3,3,3,4),(19.9659494302258,20.9479890627001,21.9455123514001,22.9430356401001,
23.9405589288002,24.9380822175002,25.9356055062002,26.2491347374054),
 .UNSPECIFIED.);
#1132=B_SPLINE_CURVE_WITH_KNOTS('',3,(#61071,#61072,#61073,#61074,#61075,
#61076,#61077,#61078,#61079,#61080,#61081,#61082,#61083,#61084,#61085,#61086,
#61087,#61088,#61089,#61090,#61091,#61092),.UNSPECIFIED.,.F.,.F.,(4,3,3,
3,3,3,3,4),(-35.5088569560286,-34.9133151045002,-33.9157918158002,-32.9182685271002,
-31.9207452384002,-30.9232219497002,-29.9256986610002,-29.225671648849),
 .UNSPECIFIED.);
#1133=B_SPLINE_CURVE_WITH_KNOTS('',3,(#61093,#61094,#61095,#61096,#61097,
#61098,#61099,#61100,#61101,#61102,#61103,#61104,#61105,#61106,#61107,#61108,
#61109,#61110,#61111,#61112,#61113,#61114),.UNSPECIFIED.,.F.,.F.,(4,3,3,
3,3,3,3,4),(26.2491347374054,26.9331287949002,27.9306520836002,28.9281753723002,
29.9256986610002,30.9232219497002,31.9207452384002,32.532320044585),
 .UNSPECIFIED.);
#1134=B_SPLINE_CURVE_WITH_KNOTS('',3,(#61119,#61120,#61121,#61122,#61123,
#61124,#61125,#61126,#61127,#61128,#61129,#61130,#61131,#61132,#61133,#61134,
#61135,#61136,#61137,#61138,#61139,#61140),.UNSPECIFIED.,.F.,.F.,(4,3,3,
3,3,3,3,4),(-41.7920422632082,-40.8984548367002,-39.9009315480002,-38.9034082593002,
-37.9058849706002,-36.9083616819002,-35.9108383932002,-35.5088569560286),
 .UNSPECIFIED.);
#1135=B_SPLINE_CURVE_WITH_KNOTS('',3,(#61141,#61142,#61143,#61144,#61145,
#61146,#61147,#61148,#61149,#61150,#61151,#61152,#61153,#61154,#61155,#61156,
#61157,#61158,#61159,#61160,#61161,#61162),.UNSPECIFIED.,.F.,.F.,(4,3,3,
3,3,3,3,4),(32.532320044585,32.9182685271002,33.9157918158002,34.9133151045002,
35.9108383932002,36.9083616819002,37.9058849706002,38.8155053517645),
 .UNSPECIFIED.);
#1136=B_SPLINE_CURVE_WITH_KNOTS('',3,(#61167,#61168,#61169,#61170,#61171,
#61172,#61173,#61174,#61175,#61176,#61177,#61178,#61179,#61180,#61181,#61182,
#61183,#61184,#61185,#61186,#61187,#61188,#61189,#61190,#61191),
 .UNSPECIFIED.,.F.,.F.,(4,3,3,3,3,3,3,3,4),(-48.0752275703878,-47.8811178576003,
-46.8835945689003,-45.8860712802002,-44.8885479915002,-43.8910247028002,
-42.8935014141002,-41.8959781254002,-41.7920422632082),.UNSPECIFIED.);
#1137=B_SPLINE_CURVE_WITH_KNOTS('',3,(#61192,#61193,#61194,#61195,#61196,
#61197,#61198,#61199,#61200,#61201,#61202,#61203,#61204,#61205,#61206,#61207,
#61208,#61209,#61210,#61211,#61212,#61213,#61214,#61215,#61216),
 .UNSPECIFIED.,.F.,.F.,(4,3,3,3,3,3,3,3,4),(38.8155053517645,38.9034082593002,
39.9009315480002,40.8984548367002,41.8959781254002,42.8935014141002,43.8910247028003,
44.8885479915003,45.0986906589441),.UNSPECIFIED.);
#1138=B_SPLINE_CURVE_WITH_KNOTS('',3,(#61221,#61222,#61223,#61224,#61225,
#61226,#61227,#61228,#61229,#61230,#61231,#61232,#61233,#61234,#61235,#61236,
#61237,#61238,#61239,#61240,#61241,#61242),.UNSPECIFIED.,.F.,.F.,(4,3,3,
3,3,3,3,4),(-54.3584128775673,-53.8662575898003,-52.8687343011003,-51.8712110124003,
-50.8736877237003,-49.8761644350003,-48.8786411463003,-48.0752275703878),
 .UNSPECIFIED.);
#1139=B_SPLINE_CURVE_WITH_KNOTS('',3,(#61243,#61244,#61245,#61246,#61247,
#61248,#61249,#61250,#61251,#61252,#61253,#61254,#61255,#61256,#61257,#61258,
#61259,#61260,#61261,#61262,#61263,#61264),.UNSPECIFIED.,.F.,.F.,(4,3,3,
3,3,3,3,4),(45.0986906589441,45.8860712802003,46.8835945689003,47.8811178576003,
48.8786411463002,49.8761644350002,50.8736877237002,51.3818759661237),
 .UNSPECIFIED.);
#1140=B_SPLINE_CURVE_WITH_KNOTS('',3,(#61269,#61270,#61271,#61272,#61273,
#61274,#61275,#61276,#61277,#61278,#61279,#61280,#61281,#61282,#61283,#61284,
#61285,#61286,#61287,#61288,#61289,#61290),.UNSPECIFIED.,.F.,.F.,(4,3,3,
3,3,3,3,4),(-60.6415981847469,-59.8513973220003,-58.8538740333003,-57.8563507446003,
-56.8588274559003,-55.8613041672003,-54.8637808785003,-54.3584128775673),
 .UNSPECIFIED.);
#1141=B_SPLINE_CURVE_WITH_KNOTS('',3,(#61291,#61292,#61293,#61294,#61295,
#61296,#61297,#61298,#61299,#61300,#61301,#61302,#61303,#61304,#61305,#61306,
#61307,#61308,#61309,#61310,#61311,#61312),.UNSPECIFIED.,.F.,.F.,(4,3,3,
3,3,3,3,4),(51.3818759661237,51.8712110124002,52.8687343011003,53.8662575898003,
54.8637808785003,55.8613041672003,56.8588274559003,57.6650612733033),
 .UNSPECIFIED.);
#1142=B_SPLINE_CURVE_WITH_KNOTS('',3,(#61317,#61318,#61319,#61320,#61321,
#61322,#61323,#61324,#61325,#61326,#61327,#61328,#61329,#61330,#61331,#61332,
#61333,#61334,#61335,#61336,#61337,#61338,#61339,#61340,#61341),
 .UNSPECIFIED.,.F.,.F.,(4,3,3,3,3,3,3,3,4),(-66.9247834919265,-66.8340603429004,
-65.8365370542004,-64.8390137655004,-63.8414904768003,-62.8439671881003,
-61.8464438994003,-60.8489206107003,-60.6415981847469),.UNSPECIFIED.);
#1143=B_SPLINE_CURVE_WITH_KNOTS('',3,(#61342,#61343,#61344,#61345,#61346,
#61347,#61348,#61349,#61350,#61351,#61352,#61353,#61354,#61355,#61356,#61357,
#61358,#61359,#61360,#61361,#61362,#61363,#61364,#61365,#61366),
 .UNSPECIFIED.,.F.,.F.,(4,3,3,3,3,3,3,3,4),(57.6650612733033,57.8563507446003,
58.8538740333003,59.8513973220003,60.8489206107003,61.8464438994003,62.8439671881003,
63.8414904768003,63.9482465804829),.UNSPECIFIED.);
#1144=B_SPLINE_CURVE_WITH_KNOTS('',3,(#61371,#61372,#61373,#61374,#61375,
#61376,#61377,#61378,#61379,#61380,#61381,#61382,#61383,#61384,#61385,#61386,
#61387,#61388,#61389,#61390,#61391,#61392),.UNSPECIFIED.,.F.,.F.,(4,3,3,
3,3,3,3,4),(-73.2079687991061,-72.8192000751004,-71.8216767864004,-70.8241534977004,
-69.8266302090004,-68.8291069203004,-67.8315836316004,-66.9247834919265),
 .UNSPECIFIED.);
#1145=B_SPLINE_CURVE_WITH_KNOTS('',3,(#61393,#61394,#61395,#61396,#61397,
#61398,#61399,#61400,#61401,#61402,#61403,#61404,#61405,#61406,#61407,#61408,
#61409,#61410,#61411,#61412,#61413,#61414),.UNSPECIFIED.,.F.,.F.,(4,3,3,
3,3,3,3,4),(63.9482465804829,64.8390137655003,65.8365370542003,66.8340603429004,
67.8315836316004,68.8291069203004,69.8266302090004,70.2314318876625),
 .UNSPECIFIED.);
#1146=B_SPLINE_CURVE_WITH_KNOTS('',3,(#61419,#61420,#61421,#61422,#61423,
#61424,#61425,#61426,#61427,#61428,#61429,#61430,#61431,#61432,#61433,#61434,
#61435,#61436,#61437,#61438,#61439,#61440),.UNSPECIFIED.,.F.,.F.,(4,3,3,
3,3,3,3,4),(-79.4911541062857,-78.8043398073004,-77.8068165186004,-76.8092932299004,
-75.8117699412004,-74.8142466525004,-73.8167233638004,-73.2079687991061),
 .UNSPECIFIED.);
#1147=B_SPLINE_CURVE_WITH_KNOTS('',3,(#61441,#61442,#61443,#61444,#61445,
#61446,#61447,#61448,#61449,#61450,#61451,#61452,#61453,#61454,#61455,#61456,
#61457,#61458,#61459,#61460,#61461,#61462),.UNSPECIFIED.,.F.,.F.,(4,3,3,
3,3,3,3,4),(70.2314318876625,70.8241534977004,71.8216767864004,72.8192000751004,
73.8167233638004,74.8142466525004,75.8117699412004,76.5146171948421),
 .UNSPECIFIED.);
#1148=B_SPLINE_CURVE_WITH_KNOTS('',3,(#61467,#61468,#61469,#61470,#61471,
#61472,#61473,#61474,#61475,#61476,#61477,#61478,#61479,#61480,#61481,#61482,
#61483,#61484,#61485,#61486,#61487,#61488),.UNSPECIFIED.,.F.,.F.,(4,3,3,
3,3,3,3,4),(-85.7743394134653,-84.7894795395005,-83.7919562508005,-82.7944329621005,
-81.7969096734005,-80.7993863847005,-79.8018630960004,-79.4911541062857),
 .UNSPECIFIED.);
#1149=B_SPLINE_CURVE_WITH_KNOTS('',3,(#61489,#61490,#61491,#61492,#61493,
#61494,#61495,#61496,#61497,#61498,#61499,#61500,#61501,#61502,#61503,#61504,
#61505,#61506,#61507,#61508,#61509,#61510,#61511,#61512,#61513),
 .UNSPECIFIED.,.F.,.F.,(4,3,3,3,3,3,3,3,4),(76.5146171948421,76.8092932299004,
77.8068165186004,78.8043398073004,79.8018630960004,80.7993863847004,81.7969096734004,
82.7944329621005,82.7978025020217),.UNSPECIFIED.);
#1150=B_SPLINE_CURVE_WITH_KNOTS('',3,(#61518,#61519,#61520,#61521,#61522,
#61523,#61524,#61525,#61526,#61527,#61528,#61529,#61530,#61531,#61532,#61533,
#61534,#61535,#61536,#61537,#61538,#61539,#61540,#61541,#61542),
 .UNSPECIFIED.,.F.,.F.,(4,3,3,3,3,3,3,3,4),(-92.0575247206449,-91.7721425604005,
-90.7746192717005,-89.7770959830005,-88.7795726943005,-87.7820494056005,
-86.7845261169005,-85.7870028282005,-85.7743394134653),.UNSPECIFIED.);
#1151=B_SPLINE_CURVE_WITH_KNOTS('',3,(#61543,#61544,#61545,#61546,#61547,
#61548,#61549,#61550,#61551,#61552,#61553,#61554,#61555,#61556,#61557,#61558,
#61559,#61560,#61561,#61562,#61563,#61564),.UNSPECIFIED.,.F.,.F.,(4,3,3,
3,3,3,3,4),(82.7978025020217,83.7919562508005,84.7894795395004,85.7870028282005,
86.7845261169005,87.7820494056005,88.7795726943005,89.0809878092013),
 .UNSPECIFIED.);
#1152=B_SPLINE_CURVE_WITH_KNOTS('',3,(#61569,#61570,#61571,#61572,#61573,
#61574,#61575,#61576,#61577,#61578,#61579,#61580,#61581,#61582,#61583,#61584,
#61585,#61586,#61587,#61588,#61589,#61590),.UNSPECIFIED.,.F.,.F.,(4,3,3,
3,3,3,3,4),(-98.3407100278245,-97.7572822926005,-96.7597590039005,-95.7622357152005,
-94.7647124265005,-93.7671891378005,-92.7696658491005,-92.0575247206449),
 .UNSPECIFIED.);
#1153=B_SPLINE_CURVE_WITH_KNOTS('',3,(#61591,#61592,#61593,#61594,#61595,
#61596,#61597,#61598,#61599,#61600,#61601,#61602,#61603,#61604,#61605,#61606,
#61607,#61608,#61609,#61610,#61611,#61612),.UNSPECIFIED.,.F.,.F.,(4,3,3,
3,3,3,3,4),(89.0809878092013,89.7770959830005,90.7746192717005,91.7721425604005,
92.7696658491005,93.7671891378005,94.7647124265005,95.3641731163809),
 .UNSPECIFIED.);
#1154=B_SPLINE_CURVE_WITH_KNOTS('',3,(#61617,#61618,#61619,#61620,#61621,
#61622,#61623,#61624,#61625,#61626,#61627,#61628,#61629,#61630,#61631,#61632,
#61633,#61634,#61635,#61636,#61637,#61638),.UNSPECIFIED.,.F.,.F.,(4,3,3,
3,3,3,3,4),(-104.623895335004,-103.742422024801,-102.744898736101,-101.747375447401,
-100.749852158701,-99.7523288700005,-98.7548055813005,-98.3407100278245),
 .UNSPECIFIED.);
#1155=B_SPLINE_CURVE_WITH_KNOTS('',3,(#61639,#61640,#61641,#61642,#61643,
#61644,#61645,#61646,#61647,#61648,#61649,#61650,#61651,#61652,#61653,#61654,
#61655,#61656,#61657,#61658,#61659,#61660),.UNSPECIFIED.,.F.,.F.,(4,3,3,
3,3,3,3,4),(95.3641731163809,95.7622357152005,96.7597590039006,97.7572822926005,
98.7548055813005,99.7523288700006,100.749852158701,101.647358423561),
 .UNSPECIFIED.);
#1156=B_SPLINE_CURVE_WITH_KNOTS('',3,(#61665,#61666,#61667,#61668,#61669,
#61670,#61671,#61672,#61673,#61674,#61675,#61676,#61677,#61678,#61679,#61680,
#61681,#61682,#61683,#61684,#61685,#61686,#61687,#61688,#61689),
 .UNSPECIFIED.,.F.,.F.,(4,3,3,3,3,3,3,3,4),(-110.907080642184,-110.725085045701,
-109.727561757001,-108.730038468301,-107.732515179601,-106.734991890901,
-105.737468602201,-104.739945313501,-104.623895335004),.UNSPECIFIED.);
#1157=B_SPLINE_CURVE_WITH_KNOTS('',3,(#61690,#61691,#61692,#61693,#61694,
#61695,#61696,#61697,#61698,#61699,#61700,#61701,#61702,#61703,#61704,#61705,
#61706,#61707,#61708,#61709,#61710,#61711,#61712,#61713,#61714),
 .UNSPECIFIED.,.F.,.F.,(4,3,3,3,3,3,3,3,4),(101.647358423561,101.747375447401,
102.744898736101,103.742422024801,104.739945313501,105.737468602201,106.734991890901,
107.732515179601,107.93054373074),.UNSPECIFIED.);
#1158=B_SPLINE_CURVE_WITH_KNOTS('',3,(#61719,#61720,#61721,#61722,#61723,
#61724,#61725,#61726,#61727,#61728,#61729,#61730,#61731,#61732,#61733,#61734,
#61735,#61736,#61737,#61738,#61739,#61740),.UNSPECIFIED.,.F.,.F.,(4,3,3,
3,3,3,3,4),(-117.190265949363,-116.710224777901,-115.712701489201,-114.715178200501,
-113.717654911801,-112.720131623101,-111.722608334401,-110.907080642184),
 .UNSPECIFIED.);
#1159=B_SPLINE_CURVE_WITH_KNOTS('',3,(#61741,#61742,#61743,#61744,#61745,
#61746,#61747,#61748,#61749,#61750,#61751,#61752,#61753,#61754,#61755,#61756,
#61757,#61758,#61759,#61760,#61761,#61762),.UNSPECIFIED.,.F.,.F.,(4,3,3,
3,3,3,3,4),(107.93054373074,108.730038468301,109.727561757001,110.725085045701,
111.722608334401,112.720131623101,113.717654911801,114.21372903792),
 .UNSPECIFIED.);
#1160=B_SPLINE_CURVE_WITH_KNOTS('',3,(#61767,#61768,#61769,#61770,#61771,
#61772,#61773,#61774,#61775,#61776,#61777,#61778,#61779,#61780,#61781,#61782,
#61783,#61784,#61785,#61786,#61787,#61788),.UNSPECIFIED.,.F.,.F.,(4,3,3,
3,3,3,3,4),(-123.473451256543,-122.695364510101,-121.697841221401,-120.700317932701,
-119.702794644001,-118.705271355301,-117.707748066601,-117.190265949363),
 .UNSPECIFIED.);
#1161=B_SPLINE_CURVE_WITH_KNOTS('',3,(#61789,#61790,#61791,#61792,#61793,
#61794,#61795,#61796,#61797,#61798,#61799,#61800,#61801,#61802,#61803,#61804,
#61805,#61806,#61807,#61808,#61809,#61810),.UNSPECIFIED.,.F.,.F.,(4,3,3,
3,3,3,3,4),(114.21372903792,114.715178200501,115.712701489201,116.710224777901,
117.707748066601,118.705271355301,119.702794644001,120.496914345099),
 .UNSPECIFIED.);
#1162=B_SPLINE_CURVE_WITH_KNOTS('',3,(#61815,#61816,#61817,#61818,#61819,
#61820,#61821,#61822,#61823,#61824,#61825,#61826,#61827,#61828,#61829,#61830,
#61831,#61832,#61833,#61834,#61835,#61836,#61837,#61838,#61839),
 .UNSPECIFIED.,.F.,.F.,(4,3,3,3,3,3,3,3,4),(-129.756636563722,-129.678027531001,
-128.680504242301,-127.682980953601,-126.685457664901,-125.687934376201,
-124.690411087501,-123.692887798801,-123.473451256543),.UNSPECIFIED.);
#1163=B_SPLINE_CURVE_WITH_KNOTS('',3,(#61840,#61841,#61842,#61843,#61844,
#61845,#61846,#61847,#61848,#61849,#61850,#61851,#61852,#61853,#61854,#61855,
#61856,#61857,#61858,#61859,#61860,#61861,#61862,#61863,#61864),
 .UNSPECIFIED.,.F.,.F.,(4,3,3,3,3,3,3,3,4),(120.496914345099,120.700317932701,
121.697841221401,122.695364510101,123.692887798801,124.690411087501,125.687934376201,
126.685457664901,126.780099652279),.UNSPECIFIED.);
#1164=B_SPLINE_CURVE_WITH_KNOTS('',3,(#61869,#61870,#61871,#61872,#61873,
#61874,#61875,#61876,#61877,#61878,#61879,#61880,#61881,#61882,#61883,#61884,
#61885,#61886,#61887,#61888,#61889,#61890),.UNSPECIFIED.,.F.,.F.,(4,3,3,
3,3,3,3,4),(-136.039821870902,-135.663167263201,-134.665643974501,-133.668120685801,
-132.670597397101,-131.673074108401,-130.675550819701,-129.756636563722),
 .UNSPECIFIED.);
#1165=B_SPLINE_CURVE_WITH_KNOTS('',3,(#61891,#61892,#61893,#61894,#61895,
#61896,#61897,#61898,#61899,#61900,#61901,#61902,#61903,#61904,#61905,#61906,
#61907,#61908,#61909,#61910,#61911,#61912),.UNSPECIFIED.,.F.,.F.,(4,3,3,
3,3,3,3,4),(126.780099652279,127.682980953601,128.680504242301,129.678027531001,
130.675550819701,131.673074108401,132.670597397101,133.063284959458),
 .UNSPECIFIED.);
#1166=B_SPLINE_CURVE_WITH_KNOTS('',3,(#61917,#61918,#61919,#61920,#61921,
#61922,#61923,#61924,#61925,#61926,#61927,#61928,#61929,#61930,#61931,#61932,
#61933,#61934,#61935,#61936,#61937,#61938),.UNSPECIFIED.,.F.,.F.,(4,3,3,
3,3,3,3,4),(-142.323007178082,-141.648306995401,-140.650783706701,-139.653260418001,
-138.655737129301,-137.658213840601,-136.660690551901,-136.039821870902),
 .UNSPECIFIED.);
#1167=B_SPLINE_CURVE_WITH_KNOTS('',3,(#61939,#61940,#61941,#61942,#61943,
#61944,#61945,#61946,#61947,#61948,#61949,#61950,#61951,#61952,#61953,#61954,
#61955,#61956,#61957,#61958,#61959,#61960),.UNSPECIFIED.,.F.,.F.,(4,3,3,
3,3,3,3,4),(133.063284959458,133.668120685801,134.665643974501,135.663167263201,
136.660690551901,137.658213840601,138.655737129301,139.346470266638),
 .UNSPECIFIED.);
#1168=B_SPLINE_CURVE_WITH_KNOTS('',3,(#61965,#61966,#61967,#61968,#61969,
#61970,#61971,#61972,#61973,#61974,#61975,#61976,#61977,#61978,#61979,#61980,
#61981,#61982,#61983,#61984,#61985,#61986),.UNSPECIFIED.,.F.,.F.,(4,3,3,
3,3,3,3,4),(-148.606192485261,-147.633446727601,-146.635923438901,-145.638400150201,
-144.640876861501,-143.643353572801,-142.645830284101,-142.323007178082),
 .UNSPECIFIED.);
#1169=B_SPLINE_CURVE_WITH_KNOTS('',3,(#61987,#61988,#61989,#61990,#61991,
#61992,#61993,#61994,#61995,#61996,#61997,#61998,#61999,#62000,#62001,#62002,
#62003,#62004,#62005,#62006,#62007,#62008),.UNSPECIFIED.,.F.,.F.,(4,3,3,
3,3,3,3,4),(139.346470266638,139.653260418001,140.650783706701,141.648306995401,
142.645830284101,143.643353572801,144.640876861501,145.629655573818),
 .UNSPECIFIED.);
#1170=B_SPLINE_CURVE_WITH_KNOTS('',3,(#62013,#62014,#62015,#62016,#62017,
#62018,#62019,#62020,#62021,#62022,#62023,#62024,#62025,#62026,#62027,#62028,
#62029,#62030,#62031,#62032,#62033,#62034,#62035,#62036,#62037),
 .UNSPECIFIED.,.F.,.F.,(4,3,3,3,3,3,3,3,4),(-154.889377792441,-154.616109748501,
-153.618586459801,-152.621063171101,-151.623539882401,-150.626016593701,
-149.628493305001,-148.630970016301,-148.606192485261),.UNSPECIFIED.);
#1171=B_SPLINE_CURVE_WITH_KNOTS('',3,(#62038,#62039,#62040,#62041,#62042,
#62043,#62044,#62045,#62046,#62047,#62048,#62049,#62050,#62051,#62052,#62053,
#62054,#62055,#62056,#62057,#62058,#62059,#62060,#62061,#62062),
 .UNSPECIFIED.,.F.,.F.,(4,3,3,3,3,3,3,3,4),(145.629655573818,145.638400150201,
146.635923438901,147.633446727601,148.630970016301,149.628493305001,150.626016593701,
151.623539882401,151.912840880997),.UNSPECIFIED.);
#1172=B_SPLINE_CURVE_WITH_KNOTS('',3,(#62067,#62068,#62069,#62070,#62071,
#62072,#62073,#62074,#62075,#62076,#62077,#62078,#62079,#62080,#62081,#62082,
#62083,#62084,#62085,#62086,#62087,#62088),.UNSPECIFIED.,.F.,.F.,(4,3,3,
3,3,3,3,4),(-161.17256309962,-160.601249480701,-159.603726192001,-158.606202903301,
-157.608679614601,-156.611156325901,-155.613633037201,-154.889377792441),
 .UNSPECIFIED.);
#1173=B_SPLINE_CURVE_WITH_KNOTS('',3,(#62089,#62090,#62091,#62092,#62093,
#62094,#62095,#62096,#62097,#62098,#62099,#62100,#62101,#62102,#62103,#62104,
#62105,#62106,#62107,#62108,#62109,#62110),.UNSPECIFIED.,.F.,.F.,(4,3,3,
3,3,3,3,4),(151.912840880997,152.621063171101,153.618586459801,154.616109748501,
155.613633037201,156.611156325901,157.608679614601,158.196026188177),
 .UNSPECIFIED.);
#1174=B_SPLINE_CURVE_WITH_KNOTS('',3,(#62115,#62116,#62117,#62118,#62119,
#62120,#62121,#62122,#62123,#62124,#62125,#62126,#62127,#62128,#62129,#62130,
#62131,#62132,#62133,#62134,#62135,#62136),.UNSPECIFIED.,.F.,.F.,(4,3,3,
3,3,3,3,4),(-167.4557484068,-166.586389212901,-165.588865924201,-164.591342635501,
-163.593819346801,-162.596296058101,-161.598772769401,-161.17256309962),
 .UNSPECIFIED.);
#1175=B_SPLINE_CURVE_WITH_KNOTS('',3,(#62137,#62138,#62139,#62140,#62141,
#62142,#62143,#62144,#62145,#62146,#62147,#62148,#62149,#62150,#62151,#62152,
#62153,#62154,#62155,#62156,#62157,#62158),.UNSPECIFIED.,.F.,.F.,(4,3,3,
3,3,3,3,4),(158.196026188177,158.606202903301,159.603726192001,160.601249480701,
161.598772769401,162.596296058101,163.593819346801,164.479211495356),
 .UNSPECIFIED.);
#1176=B_SPLINE_CURVE_WITH_KNOTS('',3,(#62163,#62164,#62165,#62166,#62167,
#62168,#62169,#62170,#62171,#62172,#62173,#62174,#62175,#62176,#62177,#62178,
#62179,#62180,#62181,#62182,#62183,#62184,#62185,#62186,#62187),
 .UNSPECIFIED.,.F.,.F.,(4,3,3,3,3,3,3,3,4),(-173.738933713979,-173.569052233801,
-172.571528945101,-171.574005656401,-170.576482367701,-169.578959079001,
-168.581435790301,-167.583912501601,-167.4557484068),.UNSPECIFIED.);
#1177=B_SPLINE_CURVE_WITH_KNOTS('',3,(#62188,#62189,#62190,#62191,#62192,
#62193,#62194,#62195,#62196,#62197,#62198,#62199,#62200,#62201,#62202,#62203,
#62204,#62205,#62206,#62207,#62208,#62209,#62210,#62211,#62212),
 .UNSPECIFIED.,.F.,.F.,(4,3,3,3,3,3,3,3,4),(164.479211495356,164.591342635501,
165.588865924201,166.586389212901,167.583912501601,168.581435790301,169.578959079001,
170.576482367701,170.762396802536),.UNSPECIFIED.);
#1178=B_SPLINE_CURVE_WITH_KNOTS('',3,(#62217,#62218,#62219,#62220,#62221,
#62222,#62223,#62224,#62225,#62226,#62227,#62228,#62229,#62230,#62231,#62232,
#62233,#62234,#62235,#62236,#62237,#62238),.UNSPECIFIED.,.F.,.F.,(4,3,3,
3,3,3,3,4),(-180.022119021159,-179.554191966001,-178.556668677301,-177.559145388601,
-176.561622099901,-175.564098811201,-174.566575522501,-173.738933713979),
 .UNSPECIFIED.);
#1179=B_SPLINE_CURVE_WITH_KNOTS('',3,(#62239,#62240,#62241,#62242,#62243,
#62244,#62245,#62246,#62247,#62248,#62249,#62250,#62251,#62252,#62253,#62254,
#62255,#62256,#62257,#62258,#62259,#62260),.UNSPECIFIED.,.F.,.F.,(4,3,3,
3,3,3,3,4),(170.762396802536,171.574005656401,172.571528945101,173.569052233801,
174.566575522501,175.564098811201,176.561622099901,177.045582109715),
 .UNSPECIFIED.);
#1180=B_SPLINE_CURVE_WITH_KNOTS('',3,(#62265,#62266,#62267,#62268,#62269,
#62270,#62271,#62272,#62273,#62274,#62275,#62276,#62277,#62278,#62279,#62280,
#62281,#62282,#62283,#62284,#62285,#62286),.UNSPECIFIED.,.F.,.F.,(4,3,3,
3,3,3,3,4),(-186.305304328338,-185.539331698201,-184.541808409501,-183.544285120801,
-182.546761832101,-181.549238543401,-180.551715254701,-180.022119021159),
 .UNSPECIFIED.);
#1181=B_SPLINE_CURVE_WITH_KNOTS('',3,(#62287,#62288,#62289,#62290,#62291,
#62292,#62293,#62294,#62295,#62296,#62297,#62298,#62299,#62300,#62301,#62302,
#62303,#62304,#62305,#62306,#62307,#62308),.UNSPECIFIED.,.F.,.F.,(4,3,3,
3,3,3,3,4),(177.045582109715,177.559145388601,178.556668677301,179.554191966001,
180.551715254701,181.549238543401,182.546761832101,183.328767416895),
 .UNSPECIFIED.);
#1182=B_SPLINE_CURVE_WITH_KNOTS('',3,(#62313,#62314,#62315,#62316,#62317,
#62318,#62319,#62320,#62321,#62322,#62323,#62324,#62325,#62326,#62327,#62328,
#62329,#62330,#62331,#62332,#62333,#62334,#62335,#62336,#62337),
 .UNSPECIFIED.,.F.,.F.,(4,3,3,3,3,3,3,3,4),(-192.588489635518,-192.521994719101,
-191.524471430401,-190.526948141701,-189.529424853001,-188.531901564301,
-187.534378275601,-186.536854986901,-186.305304328338),.UNSPECIFIED.);
#1183=B_SPLINE_CURVE_WITH_KNOTS('',3,(#62338,#62339,#62340,#62341,#62342,
#62343,#62344,#62345,#62346,#62347,#62348,#62349,#62350,#62351,#62352,#62353,
#62354,#62355,#62356,#62357,#62358,#62359,#62360,#62361,#62362),
 .UNSPECIFIED.,.F.,.F.,(4,3,3,3,3,3,3,3,4),(183.328767416895,183.544285120801,
184.541808409501,185.539331698201,186.536854986901,187.534378275601,188.531901564301,
189.529424853001,189.611952724075),.UNSPECIFIED.);
#1184=B_SPLINE_CURVE_WITH_KNOTS('',3,(#62367,#62368,#62369,#62370,#62371,
#62372,#62373,#62374,#62375,#62376,#62377,#62378,#62379,#62380,#62381,#62382,
#62383,#62384,#62385,#62386,#62387,#62388),.UNSPECIFIED.,.F.,.F.,(4,3,3,
3,3,3,3,4),(-198.871674942698,-198.507134451301,-197.509611162601,-196.512087873901,
-195.514564585201,-194.517041296501,-193.519518007801,-192.588489635518),
 .UNSPECIFIED.);
#1185=B_SPLINE_CURVE_WITH_KNOTS('',3,(#62389,#62390,#62391,#62392,#62393,
#62394,#62395,#62396,#62397,#62398,#62399,#62400,#62401,#62402,#62403,#62404,
#62405,#62406,#62407,#62408,#62409,#62410),.UNSPECIFIED.,.F.,.F.,(4,3,3,
3,3,3,3,4),(189.611952724075,190.526948141701,191.524471430401,192.521994719101,
193.519518007801,194.517041296501,195.514564585201,195.895138031254),
 .UNSPECIFIED.);
#1186=B_SPLINE_CURVE_WITH_KNOTS('',3,(#62415,#62416,#62417,#62418,#62419,
#62420,#62421,#62422,#62423,#62424,#62425,#62426,#62427,#62428,#62429,#62430,
#62431,#62432,#62433,#62434,#62435,#62436),.UNSPECIFIED.,.F.,.F.,(4,3,3,
3,3,3,3,4),(-205.154860249877,-204.492274183501,-203.494750894801,-202.497227606101,
-201.499704317401,-200.502181028701,-199.504657740001,-198.871674942698),
 .UNSPECIFIED.);
#1187=B_SPLINE_CURVE_WITH_KNOTS('',3,(#62437,#62438,#62439,#62440,#62441,
#62442,#62443,#62444,#62445,#62446,#62447,#62448,#62449,#62450,#62451,#62452,
#62453,#62454,#62455,#62456,#62457,#62458),.UNSPECIFIED.,.F.,.F.,(4,3,3,
3,3,3,3,4),(195.895138031254,196.512087873901,197.509611162601,198.507134451301,
199.504657740001,200.502181028701,201.499704317401,202.178323338434),
 .UNSPECIFIED.);
#1188=B_SPLINE_CURVE_WITH_KNOTS('',3,(#62463,#62464,#62465,#62466,#62467,
#62468,#62469,#62470,#62471,#62472,#62473,#62474,#62475,#62476,#62477,#62478,
#62479,#62480,#62481,#62482,#62483,#62484),.UNSPECIFIED.,.F.,.F.,(4,3,3,
3,3,3,3,4),(-211.438045557057,-210.477413915701,-209.479890627001,-208.482367338301,
-207.484844049601,-206.487320760901,-205.489797472201,-205.154860249877),
 .UNSPECIFIED.);
#1189=B_SPLINE_CURVE_WITH_KNOTS('',3,(#62485,#62486,#62487,#62488,#62489,
#62490,#62491,#62492,#62493,#62494,#62495,#62496,#62497,#62498,#62499,#62500,
#62501,#62502,#62503,#62504,#62505,#62506),.UNSPECIFIED.,.F.,.F.,(4,3,3,
3,3,3,3,4),(202.178323338434,202.497227606101,203.494750894801,204.492274183501,
205.489797472201,206.487320760901,207.484844049601,208.461508645613),
 .UNSPECIFIED.);
#1190=B_SPLINE_CURVE_WITH_KNOTS('',3,(#62511,#62512,#62513,#62514,#62515,
#62516,#62517,#62518,#62519,#62520,#62521,#62522,#62523,#62524,#62525,#62526,
#62527,#62528,#62529,#62530,#62531,#62532,#62533,#62534,#62535),
 .UNSPECIFIED.,.F.,.F.,(4,3,3,3,3,3,3,3,4),(-217.721230864236,-217.460076936601,
-216.462553647901,-215.465030359201,-214.467507070501,-213.469983781801,
-212.472460493101,-211.474937204401,-211.438045557057),.UNSPECIFIED.);
#1191=B_SPLINE_CURVE_WITH_KNOTS('',3,(#62536,#62537,#62538,#62539,#62540,
#62541,#62542,#62543,#62544,#62545,#62546,#62547,#62548,#62549,#62550,#62551,
#62552,#62553,#62554,#62555,#62556,#62557,#62558,#62559,#62560),
 .UNSPECIFIED.,.F.,.F.,(4,3,3,3,3,3,3,3,4),(208.461508645613,208.482367338301,
209.479890627001,210.477413915701,211.474937204401,212.472460493101,213.469983781801,
214.467507070501,214.744693952793),.UNSPECIFIED.);
#1192=B_SPLINE_CURVE_WITH_KNOTS('',3,(#62565,#62566,#62567,#62568,#62569,
#62570,#62571,#62572,#62573,#62574,#62575,#62576,#62577,#62578,#62579,#62580,
#62581,#62582,#62583,#62584,#62585,#62586),.UNSPECIFIED.,.F.,.F.,(4,3,3,
3,3,3,3,4),(-224.004416171416,-223.445216668801,-222.447693380101,-221.450170091401,
-220.452646802701,-219.455123514001,-218.457600225301,-217.721230864236),
 .UNSPECIFIED.);
#1193=B_SPLINE_CURVE_WITH_KNOTS('',3,(#62587,#62588,#62589,#62590,#62591,
#62592,#62593,#62594,#62595,#62596,#62597,#62598,#62599,#62600,#62601,#62602,
#62603,#62604,#62605,#62606,#62607,#62608),.UNSPECIFIED.,.F.,.F.,(4,3,3,
3,3,3,3,4),(214.744693952793,215.465030359201,216.462553647901,217.460076936601,
218.457600225301,219.455123514001,220.452646802701,221.027879259972),
 .UNSPECIFIED.);
#1194=B_SPLINE_CURVE_WITH_KNOTS('',3,(#62613,#62614,#62615,#62616,#62617,
#62618,#62619,#62620,#62621,#62622,#62623,#62624,#62625,#62626,#62627,#62628,
#62629,#62630,#62631,#62632,#62633,#62634),.UNSPECIFIED.,.F.,.F.,(4,3,3,
3,3,3,3,4),(-230.287601478595,-229.430356401001,-228.432833112301,-227.435309823601,
-226.437786534901,-225.440263246201,-224.442739957501,-224.004416171416),
 .UNSPECIFIED.);
#1195=B_SPLINE_CURVE_WITH_KNOTS('',3,(#62635,#62636,#62637,#62638,#62639,
#62640,#62641,#62642,#62643,#62644,#62645,#62646,#62647,#62648,#62649,#62650,
#62651,#62652,#62653,#62654,#62655,#62656),.UNSPECIFIED.,.F.,.F.,(4,3,3,
3,3,3,3,4),(221.027879259972,221.450170091401,222.447693380101,223.445216668801,
224.442739957501,225.440263246201,226.437786534901,227.311064567152),
 .UNSPECIFIED.);
#1196=B_SPLINE_CURVE_WITH_KNOTS('',3,(#62661,#62662,#62663,#62664,#62665,
#62666,#62667,#62668,#62669,#62670,#62671,#62672,#62673,#62674,#62675,#62676,
#62677,#62678,#62679,#62680,#62681,#62682,#62683,#62684,#62685),
 .UNSPECIFIED.,.F.,.F.,(4,3,3,3,3,3,3,3,4),(-236.570786785775,-236.413019421901,
-235.415496133201,-234.417972844501,-233.420449555801,-232.422926267101,
-231.425402978401,-230.427879689701,-230.287601478595),.UNSPECIFIED.);
#1197=B_SPLINE_CURVE_WITH_KNOTS('',3,(#62686,#62687,#62688,#62689,#62690,
#62691,#62692,#62693,#62694,#62695,#62696,#62697,#62698,#62699,#62700,#62701,
#62702,#62703,#62704,#62705,#62706,#62707,#62708,#62709,#62710),
 .UNSPECIFIED.,.F.,.F.,(4,3,3,3,3,3,3,3,4),(227.311064567152,227.435309823601,
228.432833112301,229.430356401001,230.427879689701,231.425402978401,232.422926267101,
233.420449555801,233.594249874331),.UNSPECIFIED.);
#1198=B_SPLINE_CURVE_WITH_KNOTS('',3,(#62715,#62716,#62717,#62718,#62719,
#62720,#62721,#62722,#62723,#62724,#62725,#62726,#62727,#62728,#62729,#62730,
#62731,#62732,#62733,#62734,#62735,#62736),.UNSPECIFIED.,.F.,.F.,(4,3,3,
3,3,3,3,4),(-242.853972092955,-242.398159154101,-241.400635865401,-240.403112576701,
-239.405589288001,-238.408065999301,-237.410542710601,-236.570786785775),
 .UNSPECIFIED.);
#1199=B_SPLINE_CURVE_WITH_KNOTS('',3,(#62737,#62738,#62739,#62740,#62741,
#62742,#62743,#62744,#62745,#62746,#62747,#62748,#62749,#62750,#62751,#62752,
#62753,#62754,#62755,#62756,#62757,#62758),.UNSPECIFIED.,.F.,.F.,(4,3,3,
3,3,3,3,4),(233.594249874331,234.417972844501,235.415496133201,236.413019421901,
237.410542710601,238.408065999301,239.405589288001,239.877435181511),
 .UNSPECIFIED.);
#1200=B_SPLINE_CURVE_WITH_KNOTS('',3,(#62763,#62764,#62765,#62766,#62767,
#62768,#62769,#62770,#62771,#62772,#62773,#62774,#62775,#62776,#62777,#62778,
#62779,#62780,#62781,#62782,#62783,#62784),.UNSPECIFIED.,.F.,.F.,(4,3,3,
3,3,3,3,4),(-249.137157400134,-248.383298886301,-247.385775597601,-246.388252308901,
-245.390729020201,-244.393205731501,-243.395682442801,-242.853972092955),
 .UNSPECIFIED.);
#1201=B_SPLINE_CURVE_WITH_KNOTS('',3,(#62785,#62786,#62787,#62788,#62789,
#62790,#62791,#62792,#62793,#62794,#62795,#62796,#62797,#62798,#62799,#62800,
#62801,#62802,#62803,#62804,#62805,#62806),.UNSPECIFIED.,.F.,.F.,(4,3,3,
3,3,3,3,4),(239.877435181511,240.403112576701,241.400635865401,242.398159154101,
243.395682442801,244.393205731501,245.390729020201,246.160620488691),
 .UNSPECIFIED.);
#1202=B_SPLINE_CURVE_WITH_KNOTS('',3,(#62811,#62812,#62813,#62814,#62815,
#62816,#62817,#62818,#62819,#62820,#62821,#62822,#62823,#62824,#62825,#62826,
#62827,#62828,#62829,#62830,#62831,#62832,#62833,#62834,#62835),
 .UNSPECIFIED.,.F.,.F.,(4,3,3,3,3,3,3,3,4),(-255.420342707314,-255.365961907201,
-254.368438618501,-253.370915329801,-252.373392041101,-251.375868752401,
-250.378345463701,-249.380822175001,-249.137157400134),.UNSPECIFIED.);
#1203=B_SPLINE_CURVE_WITH_KNOTS('',3,(#62836,#62837,#62838,#62839,#62840,
#62841,#62842,#62843,#62844,#62845,#62846,#62847,#62848,#62849,#62850,#62851,
#62852,#62853,#62854,#62855,#62856,#62857,#62858,#62859,#62860),
 .UNSPECIFIED.,.F.,.F.,(4,3,3,3,3,3,3,3,4),(246.160620488691,246.388252308901,
247.385775597601,248.383298886301,249.380822175001,250.378345463701,251.375868752401,
252.373392041101,252.44380579587),.UNSPECIFIED.);
#1204=B_SPLINE_CURVE_WITH_KNOTS('',3,(#62865,#62866,#62867,#62868,#62869,
#62870,#62871,#62872,#62873,#62874,#62875,#62876,#62877,#62878,#62879,#62880,
#62881,#62882,#62883,#62884,#62885,#62886),.UNSPECIFIED.,.F.,.F.,(4,3,3,
3,3,3,3,4),(-261.703528014493,-261.351101639401,-260.353578350701,-259.356055062001,
-258.358531773301,-257.361008484601,-256.363485195901,-255.420342707314),
 .UNSPECIFIED.);
#1205=B_SPLINE_CURVE_WITH_KNOTS('',3,(#62887,#62888,#62889,#62890,#62891,
#62892,#62893,#62894,#62895,#62896,#62897,#62898,#62899,#62900,#62901,#62902,
#62903,#62904,#62905,#62906,#62907,#62908),.UNSPECIFIED.,.F.,.F.,(4,3,3,
3,3,3,3,4),(252.44380579587,253.370915329801,254.368438618501,255.365961907201,
256.363485195901,257.361008484601,258.358531773301,258.72699110305),
 .UNSPECIFIED.);
#1206=B_SPLINE_CURVE_WITH_KNOTS('',3,(#62913,#62914,#62915,#62916,#62917,
#62918,#62919,#62920,#62921,#62922,#62923,#62924,#62925,#62926,#62927,#62928,
#62929,#62930,#62931,#62932,#62933,#62934),.UNSPECIFIED.,.F.,.F.,(4,3,3,
3,3,3,3,4),(-267.986713321673,-267.336241371601,-266.338718082901,-265.341194794201,
-264.343671505501,-263.346148216802,-262.348624928101,-261.703528014493),
 .UNSPECIFIED.);
#1207=B_SPLINE_CURVE_WITH_KNOTS('',3,(#62935,#62936,#62937,#62938,#62939,
#62940,#62941,#62942,#62943,#62944,#62945,#62946,#62947,#62948,#62949,#62950,
#62951,#62952,#62953,#62954,#62955,#62956),.UNSPECIFIED.,.F.,.F.,(4,3,3,
3,3,3,3,4),(258.72699110305,259.356055062001,260.353578350701,261.351101639402,
262.348624928102,263.346148216802,264.343671505502,265.010176410229),
 .UNSPECIFIED.);
#1208=B_SPLINE_CURVE_WITH_KNOTS('',3,(#62961,#62962,#62963,#62964,#62965,
#62966,#62967,#62968,#62969,#62970,#62971,#62972,#62973,#62974,#62975,#62976,
#62977,#62978,#62979,#62980,#62981,#62982),.UNSPECIFIED.,.F.,.F.,(4,3,3,
3,3,3,3,4),(-274.269898628852,-273.321381103802,-272.323857815102,-271.326334526402,
-270.328811237701,-269.331287949001,-268.333764660301,-267.986713321673),
 .UNSPECIFIED.);
#1209=B_SPLINE_CURVE_WITH_KNOTS('',3,(#62983,#62984,#62985,#62986,#62987,
#62988,#62989,#62990,#62991,#62992,#62993,#62994,#62995,#62996,#62997,#62998,
#62999,#63000,#63001,#63002,#63003,#63004),.UNSPECIFIED.,.F.,.F.,(4,3,3,
3,3,3,3,4),(265.010176410229,265.341194794201,266.338718082902,267.336241371602,
268.333764660302,269.331287949002,270.328811237702,271.293361717409),
 .UNSPECIFIED.);
#1210=B_SPLINE_CURVE_WITH_KNOTS('',3,(#63009,#63010,#63011,#63012,#63013,
#63014,#63015,#63016,#63017,#63018,#63019,#63020,#63021,#63022,#63023,#63024,
#63025,#63026,#63027,#63028,#63029,#63030,#63031,#63032,#63033),
 .UNSPECIFIED.,.F.,.F.,(4,3,3,3,3,3,3,3,4),(-280.553083936032,-280.304044124702,
-279.306520836001,-278.308997547301,-277.311474258601,-276.313950969901,
-275.316427681202,-274.318904392502,-274.269898628852),.UNSPECIFIED.);
#1211=B_SPLINE_CURVE_WITH_KNOTS('',3,(#63034,#63035,#63036,#63037,#63038,
#63039,#63040,#63041,#63042,#63043,#63044,#63045,#63046,#63047,#63048,#63049,
#63050,#63051,#63052,#63053,#63054,#63055,#63056,#63057,#63058),
 .UNSPECIFIED.,.F.,.F.,(4,3,3,3,3,3,3,3,4),(271.293361717409,271.326334526402,
272.323857815102,273.321381103802,274.318904392502,275.316427681202,276.313950969902,
277.311474258602,277.576547024588),.UNSPECIFIED.);
#1212=B_SPLINE_CURVE_WITH_KNOTS('',3,(#63063,#63064,#63065,#63066,#63067,
#63068,#63069,#63070,#63071,#63072,#63073,#63074,#63075,#63076,#63077,#63078,
#63079,#63080,#63081,#63082,#63083,#63084),.UNSPECIFIED.,.F.,.F.,(4,3,3,
3,3,3,3,4),(-286.836269243212,-286.289183856902,-285.291660568202,-284.294137279502,
-283.296613990802,-282.299090702102,-281.301567413402,-280.553083936032),
 .UNSPECIFIED.);
#1213=B_SPLINE_CURVE_WITH_KNOTS('',3,(#63085,#63086,#63087,#63088,#63089,
#63090,#63091,#63092,#63093,#63094,#63095,#63096,#63097,#63098,#63099,#63100,
#63101,#63102,#63103,#63104,#63105,#63106),.UNSPECIFIED.,.F.,.F.,(4,3,3,
3,3,3,3,4),(277.576547024588,278.308997547302,279.306520836002,280.304044124702,
281.301567413402,282.299090702102,283.296613990802,283.859732331768),
 .UNSPECIFIED.);
#1214=B_SPLINE_CURVE_WITH_KNOTS('',3,(#63111,#63112,#63113,#63114,#63115,
#63116,#63117,#63118,#63119,#63120,#63121,#63122,#63123,#63124,#63125,#63126,
#63127,#63128,#63129,#63130,#63131,#63132),.UNSPECIFIED.,.F.,.F.,(4,3,3,
3,3,3,3,4),(-293.119454550391,-292.274323589102,-291.276800300402,-290.279277011702,
-289.281753723002,-288.284230434302,-287.286707145602,-286.836269243212),
 .UNSPECIFIED.);
#1215=B_SPLINE_CURVE_WITH_KNOTS('',3,(#63133,#63134,#63135,#63136,#63137,
#63138,#63139,#63140,#63141,#63142,#63143,#63144,#63145,#63146,#63147,#63148,
#63149,#63150,#63151,#63152,#63153,#63154),.UNSPECIFIED.,.F.,.F.,(4,3,3,
3,3,3,3,4),(283.859732331768,284.294137279502,285.291660568202,286.289183856902,
287.286707145602,288.284230434302,289.281753723002,290.142917638947),
 .UNSPECIFIED.);
#1216=B_SPLINE_CURVE_WITH_KNOTS('',3,(#63159,#63160,#63161,#63162,#63163,
#63164,#63165,#63166,#63167,#63168,#63169,#63170,#63171,#63172,#63173,#63174,
#63175,#63176,#63177,#63178,#63179,#63180,#63181,#63182,#63183),
 .UNSPECIFIED.,.F.,.F.,(4,3,3,3,3,3,3,3,4),(-299.402639857571,-299.256986610002,
-298.259463321302,-297.261940032602,-296.264416743902,-295.266893455202,
-294.269370166502,-293.271846877802,-293.119454550391),.UNSPECIFIED.);
#1217=B_SPLINE_CURVE_WITH_KNOTS('',3,(#63184,#63185,#63186,#63187,#63188,
#63189,#63190,#63191,#63192,#63193,#63194,#63195,#63196,#63197,#63198,#63199,
#63200,#63201,#63202,#63203,#63204,#63205,#63206,#63207,#63208),
 .UNSPECIFIED.,.F.,.F.,(4,3,3,3,3,3,3,3,4),(290.142917638947,290.279277011702,
291.276800300402,292.274323589102,293.271846877802,294.269370166502,295.266893455202,
296.264416743902,296.426102946127),.UNSPECIFIED.);
#1218=B_SPLINE_CURVE_WITH_KNOTS('',3,(#63213,#63214,#63215,#63216,#63217,
#63218,#63219,#63220,#63221,#63222,#63223,#63224,#63225,#63226,#63227,#63228,
#63229,#63230,#63231,#63232,#63233,#63234),.UNSPECIFIED.,.F.,.F.,(4,3,3,
3,3,3,3,4),(-305.68582516475,-305.242126342202,-304.244603053502,-303.247079764802,
-302.249556476102,-301.252033187402,-300.254509898702,-299.402639857571),
 .UNSPECIFIED.);
#1219=B_SPLINE_CURVE_WITH_KNOTS('',3,(#63235,#63236,#63237,#63238,#63239,
#63240,#63241,#63242,#63243,#63244,#63245,#63246,#63247,#63248,#63249,#63250,
#63251,#63252,#63253,#63254,#63255,#63256),.UNSPECIFIED.,.F.,.F.,(4,3,3,
3,3,3,3,4),(296.426102946127,297.261940032602,298.259463321302,299.256986610002,
300.254509898702,301.252033187402,302.249556476102,302.709288253307),
 .UNSPECIFIED.);
#1220=B_SPLINE_CURVE_WITH_KNOTS('',3,(#63261,#63262,#63263,#63264,#63265,
#63266,#63267,#63268,#63269,#63270,#63271,#63272,#63273,#63274,#63275,#63276,
#63277,#63278,#63279,#63280,#63281,#63282),.UNSPECIFIED.,.F.,.F.,(4,3,3,
3,3,3,3,4),(-311.96901047193,-311.227266074402,-310.229742785702,-309.232219497002,
-308.234696208302,-307.237172919602,-306.239649630902,-305.68582516475),
 .UNSPECIFIED.);
#1221=B_SPLINE_CURVE_WITH_KNOTS('',3,(#63283,#63284,#63285,#63286,#63287,
#63288,#63289,#63290,#63291,#63292,#63293,#63294,#63295,#63296,#63297,#63298,
#63299,#63300,#63301,#63302,#63303,#63304),.UNSPECIFIED.,.F.,.F.,(4,3,3,
3,3,3,3,4),(302.709288253307,303.247079764802,304.244603053502,305.242126342202,
306.239649630902,307.237172919602,308.234696208302,308.992473560486),
 .UNSPECIFIED.);
#1222=B_SPLINE_CURVE_WITH_KNOTS('',3,(#63309,#63310,#63311,#63312,#63313,
#63314,#63315,#63316,#63317,#63318,#63319,#63320,#63321,#63322,#63323,#63324,
#63325,#63326,#63327,#63328,#63329,#63330,#63331,#63332,#63333),
 .UNSPECIFIED.,.F.,.F.,(4,3,3,3,3,3,3,3,4),(-318.252195779109,-318.209929095302,
-317.212405806602,-316.214882517902,-315.217359229202,-314.219835940502,
-313.222312651802,-312.224789363102,-311.96901047193),.UNSPECIFIED.);
#1223=B_SPLINE_CURVE_WITH_KNOTS('',3,(#63334,#63335,#63336,#63337,#63338,
#63339,#63340,#63341,#63342,#63343,#63344,#63345,#63346,#63347,#63348,#63349,
#63350,#63351,#63352,#63353,#63354,#63355,#63356,#63357,#63358),
 .UNSPECIFIED.,.F.,.F.,(4,3,3,3,3,3,3,3,4),(308.992473560486,309.232219497002,
310.229742785702,311.227266074402,312.224789363102,313.222312651802,314.219835940502,
315.217359229202,315.275658867666),.UNSPECIFIED.);
#1224=B_SPLINE_CURVE_WITH_KNOTS('',3,(#63363,#63364,#63365,#63366,#63367,
#63368,#63369,#63370,#63371,#63372,#63373,#63374,#63375,#63376,#63377,#63378,
#63379,#63380,#63381,#63382,#63383,#63384),.UNSPECIFIED.,.F.,.F.,(4,3,3,
3,3,3,3,4),(-324.535381086289,-324.195068827502,-323.197545538802,-322.200022250102,
-321.202498961402,-320.204975672702,-319.207452384002,-318.252195779109),
 .UNSPECIFIED.);
#1225=B_SPLINE_CURVE_WITH_KNOTS('',3,(#63385,#63386,#63387,#63388,#63389,
#63390,#63391,#63392,#63393,#63394,#63395,#63396,#63397,#63398,#63399,#63400,
#63401,#63402,#63403,#63404,#63405,#63406),.UNSPECIFIED.,.F.,.F.,(4,3,3,
3,3,3,3,4),(315.275658867666,316.214882517902,317.212405806602,318.209929095302,
319.207452384002,320.204975672702,321.202498961402,321.558844174845),
 .UNSPECIFIED.);
#1226=B_SPLINE_CURVE_WITH_KNOTS('',3,(#63411,#63412,#63413,#63414,#63415,
#63416,#63417,#63418,#63419,#63420,#63421,#63422,#63423,#63424,#63425,#63426,
#63427,#63428,#63429,#63430,#63431,#63432),.UNSPECIFIED.,.F.,.F.,(4,3,3,
3,3,3,3,4),(-330.818566393468,-330.180208559702,-329.182685271002,-328.185161982302,
-327.187638693602,-326.190115404902,-325.192592116202,-324.535381086289),
 .UNSPECIFIED.);
#1227=B_SPLINE_CURVE_WITH_KNOTS('',3,(#63433,#63434,#63435,#63436,#63437,
#63438,#63439,#63440,#63441,#63442,#63443,#63444,#63445,#63446,#63447,#63448,
#63449,#63450,#63451,#63452,#63453,#63454),.UNSPECIFIED.,.F.,.F.,(4,3,3,
3,3,3,3,4),(321.558844174845,322.200022250102,323.197545538802,324.195068827502,
325.192592116202,326.190115404902,327.187638693602,327.842029482025),
 .UNSPECIFIED.);
#1228=B_SPLINE_CURVE_WITH_KNOTS('',3,(#63459,#63460,#63461,#63462,#63463,
#63464,#63465,#63466,#63467,#63468,#63469,#63470,#63471,#63472,#63473,#63474,
#63475,#63476,#63477,#63478,#63479,#63480),.UNSPECIFIED.,.F.,.F.,(4,3,3,
3,3,3,3,4),(-337.101751700648,-336.165348291902,-335.167825003202,-334.170301714502,
-333.172778425802,-332.175255137102,-331.177731848402,-330.818566393468),
 .UNSPECIFIED.);
#1229=B_SPLINE_CURVE_WITH_KNOTS('',3,(#63481,#63482,#63483,#63484,#63485,
#63486,#63487,#63488,#63489,#63490,#63491,#63492,#63493,#63494,#63495,#63496,
#63497,#63498,#63499,#63500,#63501,#63502),.UNSPECIFIED.,.F.,.F.,(4,3,3,
3,3,3,3,4),(327.842029482025,328.185161982302,329.182685271002,330.180208559702,
331.177731848402,332.175255137102,333.172778425802,334.125214789205),
 .UNSPECIFIED.);
#1230=B_SPLINE_CURVE_WITH_KNOTS('',3,(#63507,#63508,#63509,#63510,#63511,
#63512,#63513,#63514,#63515,#63516,#63517,#63518,#63519,#63520,#63521,#63522,
#63523,#63524,#63525,#63526,#63527,#63528,#63529,#63530,#63531),
 .UNSPECIFIED.,.F.,.F.,(4,3,3,3,3,3,3,3,4),(-343.384937007828,-343.148011312802,
-342.150488024102,-341.152964735402,-340.155441446702,-339.157918158002,
-338.160394869302,-337.162871580602,-337.101751700648),.UNSPECIFIED.);
#1231=B_SPLINE_CURVE_WITH_KNOTS('',3,(#63532,#63533,#63534,#63535,#63536,
#63537,#63538,#63539,#63540,#63541,#63542,#63543,#63544,#63545,#63546,#63547,
#63548,#63549,#63550,#63551,#63552,#63553,#63554,#63555,#63556),
 .UNSPECIFIED.,.F.,.F.,(4,3,3,3,3,3,3,3,4),(334.125214789205,334.170301714502,
335.167825003202,336.165348291902,337.162871580602,338.160394869302,339.157918158002,
340.155441446702,340.408400096384),.UNSPECIFIED.);
#1232=B_SPLINE_CURVE_WITH_KNOTS('',3,(#63561,#63562,#63563,#63564,#63565,
#63566,#63567,#63568,#63569,#63570,#63571,#63572,#63573,#63574,#63575,#63576,
#63577,#63578,#63579,#63580,#63581,#63582),.UNSPECIFIED.,.F.,.F.,(4,3,3,
3,3,3,3,4),(-349.668122315007,-349.133151045002,-348.135627756302,-347.138104467602,
-346.140581178902,-345.143057890202,-344.145534601502,-343.384937007828),
 .UNSPECIFIED.);
#1233=B_SPLINE_CURVE_WITH_KNOTS('',3,(#63583,#63584,#63585,#63586,#63587,
#63588,#63589,#63590,#63591,#63592,#63593,#63594,#63595,#63596,#63597,#63598,
#63599,#63600,#63601,#63602,#63603,#63604),.UNSPECIFIED.,.F.,.F.,(4,3,3,
3,3,3,3,4),(340.408400096384,341.152964735402,342.150488024102,343.148011312802,
344.145534601502,345.143057890202,346.140581178902,346.691585403564),
 .UNSPECIFIED.);
#1234=B_SPLINE_CURVE_WITH_KNOTS('',3,(#63609,#63610,#63611,#63612,#63613,
#63614,#63615,#63616,#63617,#63618,#63619,#63620,#63621,#63622,#63623,#63624,
#63625,#63626,#63627,#63628,#63629,#63630),.UNSPECIFIED.,.F.,.F.,(4,3,3,
3,3,3,3,4),(-355.951307622187,-355.118290777202,-354.120767488502,-353.123244199802,
-352.125720911102,-351.128197622402,-350.130674333702,-349.668122315007),
 .UNSPECIFIED.);
#1235=B_SPLINE_CURVE_WITH_KNOTS('',3,(#63631,#63632,#63633,#63634,#63635,
#63636,#63637,#63638,#63639,#63640,#63641,#63642,#63643,#63644,#63645,#63646,
#63647,#63648,#63649,#63650,#63651,#63652),.UNSPECIFIED.,.F.,.F.,(4,3,3,
3,3,3,3,4),(346.691585403564,347.138104467602,348.135627756302,349.133151045002,
350.130674333702,351.128197622402,352.125720911102,352.974770710743),
 .UNSPECIFIED.);
#1236=B_SPLINE_CURVE_WITH_KNOTS('',3,(#63657,#63658,#63659,#63660,#63661,
#63662,#63663,#63664,#63665,#63666,#63667,#63668,#63669,#63670,#63671,#63672,
#63673,#63674,#63675,#63676,#63677,#63678,#63679,#63680,#63681),
 .UNSPECIFIED.,.F.,.F.,(4,3,3,3,3,3,3,3,4),(-362.234492929366,-362.100953798102,
-361.103430509402,-360.105907220702,-359.108383932002,-358.110860643302,
-357.113337354602,-356.115814065902,-355.951307622187),.UNSPECIFIED.);
#1237=B_SPLINE_CURVE_WITH_KNOTS('',3,(#63682,#63683,#63684,#63685,#63686,
#63687,#63688,#63689,#63690,#63691,#63692,#63693,#63694,#63695,#63696,#63697,
#63698,#63699,#63700,#63701,#63702,#63703,#63704,#63705,#63706),
 .UNSPECIFIED.,.F.,.F.,(4,3,3,3,3,3,3,3,4),(352.974770710743,353.123244199802,
354.120767488502,355.118290777202,356.115814065902,357.113337354602,358.110860643302,
359.108383932002,359.257956017923),.UNSPECIFIED.);
#1238=B_SPLINE_CURVE_WITH_KNOTS('',3,(#63711,#63712,#63713,#63714,#63715,
#63716,#63717,#63718,#63719,#63720,#63721,#63722,#63723,#63724,#63725,#63726,
#63727,#63728,#63729,#63730,#63731,#63732),.UNSPECIFIED.,.F.,.F.,(4,3,3,
3,3,3,3,4),(-368.517678236546,-368.086093530302,-367.088570241602,-366.091046952902,
-365.093523664202,-364.096000375502,-363.098477086802,-362.234492929366),
 .UNSPECIFIED.);
#1239=B_SPLINE_CURVE_WITH_KNOTS('',3,(#63733,#63734,#63735,#63736,#63737,
#63738,#63739,#63740,#63741,#63742,#63743,#63744,#63745,#63746,#63747,#63748,
#63749,#63750,#63751,#63752,#63753,#63754),.UNSPECIFIED.,.F.,.F.,(4,3,3,
3,3,3,3,4),(359.257956017923,360.105907220702,361.103430509402,362.100953798102,
363.098477086802,364.096000375502,365.093523664202,365.541141325102),
 .UNSPECIFIED.);
#1240=B_SPLINE_CURVE_WITH_KNOTS('',3,(#63759,#63760,#63761,#63762,#63763,
#63764,#63765,#63766,#63767,#63768,#63769,#63770,#63771,#63772,#63773,#63774,
#63775,#63776,#63777,#63778,#63779,#63780),.UNSPECIFIED.,.F.,.F.,(4,3,3,
3,3,3,3,4),(-374.800863543725,-374.071233262502,-373.073709973802,-372.076186685102,
-371.078663396402,-370.081140107702,-369.083616819002,-368.517678236546),
 .UNSPECIFIED.);
#1241=B_SPLINE_CURVE_WITH_KNOTS('',3,(#63781,#63782,#63783,#63784,#63785,
#63786,#63787,#63788,#63789,#63790,#63791,#63792,#63793,#63794,#63795,#63796,
#63797,#63798,#63799,#63800,#63801,#63802),.UNSPECIFIED.,.F.,.F.,(4,3,3,
3,3,3,3,4),(365.541141325102,366.091046952902,367.088570241602,368.086093530302,
369.083616819002,370.081140107702,371.078663396402,371.824326632282),
 .UNSPECIFIED.);
#1242=B_SPLINE_CURVE_WITH_KNOTS('',3,(#63808,#63809,#63810,#63811,#63812,
#63813),.UNSPECIFIED.,.F.,.F.,(4,1,1,4),(386.415896391544,386.683789399021,
387.681312687721,388.606151278594),.UNSPECIFIED.);
#1243=B_SPLINE_CURVE_WITH_KNOTS('',3,(#63816,#63817,#63818,#63819,#63820),
 .UNSPECIFIED.,.F.,.F.,(4,1,4),(386.415896391544,386.868472513736,387.367234158086),
 .UNSPECIFIED.);
#1244=B_SPLINE_CURVE_WITH_KNOTS('',3,(#63825,#63826,#63827,#63828,#63829,
#63830,#63831,#63832,#63833,#63834),.UNSPECIFIED.,.F.,.F.,(4,1,1,1,1,1,
1,4),(380.132711084365,380.698649666821,381.696172955521,382.693696244221,
383.691219532921,384.688742821621,385.686266110321,386.415896391544),
 .UNSPECIFIED.);
#1245=B_SPLINE_CURVE_WITH_KNOTS('',3,(#63835,#63836,#63837,#63838,#63839,
#63840,#63841,#63842,#63843,#63844,#63845),.UNSPECIFIED.,.F.,.F.,(4,1,1,
1,1,1,1,1,4),(380.132711084365,380.384571137186,381.382094425886,382.379617714586,
383.377141003286,384.374664291986,385.372187580686,386.369710869386,386.415896391544),
 .UNSPECIFIED.);
#1246=B_SPLINE_CURVE_WITH_KNOTS('',3,(#63850,#63851,#63852,#63853,#63854,
#63855,#63856,#63857,#63858,#63859),.UNSPECIFIED.,.F.,.F.,(4,1,1,1,1,1,
1,4),(373.849525777185,374.713509934621,375.711033223321,376.708556512021,
377.706079800721,378.703603089421,379.701126378121,380.132711084365),
 .UNSPECIFIED.);
#1247=B_SPLINE_CURVE_WITH_KNOTS('',3,(#63860,#63861,#63862,#63863,#63864,
#63865,#63866,#63867,#63868,#63869),.UNSPECIFIED.,.F.,.F.,(4,1,1,1,1,1,
1,4),(373.849525777185,374.399431404986,375.396954693686,376.394477982386,
377.392001271086,378.389524559786,379.387047848486,380.132711084365),
 .UNSPECIFIED.);
#1248=B_SPLINE_CURVE_WITH_KNOTS('',3,(#63874,#63875,#63876,#63877,#63878,
#63879,#63880,#63881,#63882,#63883,#63884),.UNSPECIFIED.,.F.,.F.,(4,1,1,
1,1,1,1,1,4),(367.566340470006,367.730846913721,368.728370202421,369.725893491121,
370.723416779821,371.720940068521,372.718463357221,373.715986645921,373.849525777185),
 .UNSPECIFIED.);
#1249=B_SPLINE_CURVE_WITH_KNOTS('',3,(#63885,#63886,#63887,#63888,#63889,
#63890,#63891,#63892,#63893,#63894),.UNSPECIFIED.,.F.,.F.,(4,1,1,1,1,1,
1,4),(367.566340470006,368.414291672786,369.411814961486,370.409338250186,
371.406861538886,372.404384827586,373.401908116286,373.849525777185),
 .UNSPECIFIED.);
#1250=B_SPLINE_CURVE_WITH_KNOTS('',3,(#63899,#63900,#63901,#63902,#63903,
#63904,#63905,#63906,#63907,#63908),.UNSPECIFIED.,.F.,.F.,(4,1,1,1,1,1,
1,4),(361.283155162826,361.745707181521,362.743230470221,363.740753758921,
364.738277047621,365.735800336321,366.733323625021,367.566340470006),
 .UNSPECIFIED.);
#1251=B_SPLINE_CURVE_WITH_KNOTS('',3,(#63909,#63910,#63911,#63912,#63913,
#63914,#63915,#63916,#63917,#63918,#63919),.UNSPECIFIED.,.F.,.F.,(4,1,1,
1,1,1,1,1,4),(361.283155162826,361.431628651886,362.429151940586,363.426675229286,
364.424198517986,365.421721806686,366.419245095386,367.416768384086,367.566340470006),
 .UNSPECIFIED.);
#1252=B_SPLINE_CURVE_WITH_KNOTS('',3,(#63924,#63925,#63926,#63927,#63928,
#63929,#63930,#63931,#63932,#63933),.UNSPECIFIED.,.F.,.F.,(4,1,1,1,1,1,
1,4),(354.999969855647,355.760567449321,356.758090738021,357.755614026721,
358.753137315421,359.750660604121,360.748183892821,361.283155162826),
 .UNSPECIFIED.);
#1253=B_SPLINE_CURVE_WITH_KNOTS('',3,(#63934,#63935,#63936,#63937,#63938,
#63939,#63940,#63941,#63942,#63943),.UNSPECIFIED.,.F.,.F.,(4,1,1,1,1,1,
1,4),(354.999969855647,355.446488919686,356.444012208386,357.441535497086,
358.439058785786,359.436582074486,360.434105363186,361.283155162826),
 .UNSPECIFIED.);
#1254=B_SPLINE_CURVE_WITH_KNOTS('',3,(#63948,#63949,#63950,#63951,#63952,
#63953,#63954,#63955,#63956,#63957,#63958),.UNSPECIFIED.,.F.,.F.,(4,1,1,
1,1,1,1,1,4),(348.716784548467,348.777904428421,349.775427717121,350.772951005821,
351.770474294521,352.767997583221,353.765520871921,354.763044160621,354.999969855647),
 .UNSPECIFIED.);
#1255=B_SPLINE_CURVE_WITH_KNOTS('',3,(#63959,#63960,#63961,#63962,#63963,
#63964,#63965,#63966,#63967,#63968),.UNSPECIFIED.,.F.,.F.,(4,1,1,1,1,1,
1,4),(348.716784548467,349.461349187486,350.458872476186,351.456395764886,
352.453919053586,353.451442342286,354.448965630986,354.999969855647),
 .UNSPECIFIED.);
#1256=B_SPLINE_CURVE_WITH_KNOTS('',3,(#63973,#63974,#63975,#63976,#63977,
#63978,#63979,#63980,#63981,#63982),.UNSPECIFIED.,.F.,.F.,(4,1,1,1,1,1,
1,4),(342.433599241287,342.792764696221,343.790287984921,344.787811273621,
345.785334562321,346.782857851021,347.780381139721,348.716784548467),
 .UNSPECIFIED.);
#1257=B_SPLINE_CURVE_WITH_KNOTS('',3,(#63983,#63984,#63985,#63986,#63987,
#63988,#63989,#63990,#63991,#63992,#63993),.UNSPECIFIED.,.F.,.F.,(4,1,1,
1,1,1,1,1,4),(342.433599241287,342.478686166586,343.476209455286,344.473732743986,
345.471256032686,346.468779321386,347.466302610086,348.463825898786,348.716784548467),
 .UNSPECIFIED.);
#1258=B_SPLINE_CURVE_WITH_KNOTS('',3,(#63998,#63999,#64000,#64001,#64002,
#64003,#64004,#64005,#64006,#64007),.UNSPECIFIED.,.F.,.F.,(4,1,1,1,1,1,
1,4),(336.150413934108,336.807624964021,337.805148252721,338.802671541421,
339.800194830121,340.797718118821,341.795241407521,342.433599241287),
 .UNSPECIFIED.);
#1259=B_SPLINE_CURVE_WITH_KNOTS('',3,(#64008,#64009,#64010,#64011,#64012,
#64013,#64014,#64015,#64016,#64017),.UNSPECIFIED.,.F.,.F.,(4,1,1,1,1,1,
1,4),(336.150413934108,336.493546434386,337.491069723086,338.488593011786,
339.486116300486,340.483639589186,341.481162877886,342.433599241287),
 .UNSPECIFIED.);
#1260=B_SPLINE_CURVE_WITH_KNOTS('',3,(#64022,#64023,#64024,#64025,#64026,
#64027,#64028,#64029,#64030,#64031),.UNSPECIFIED.,.F.,.F.,(4,1,1,1,1,1,
1,4),(329.867228626928,330.822485231821,331.820008520521,332.817531809221,
333.815055097921,334.812578386621,335.810101675321,336.150413934108),
 .UNSPECIFIED.);
#1261=B_SPLINE_CURVE_WITH_KNOTS('',3,(#64032,#64033,#64034,#64035,#64036,
#64037,#64038,#64039,#64040,#64041),.UNSPECIFIED.,.F.,.F.,(4,1,1,1,1,1,
1,4),(329.867228626928,330.508406702186,331.505929990886,332.503453279586,
333.500976568286,334.498499856986,335.496023145686,336.150413934108),
 .UNSPECIFIED.);
#1262=B_SPLINE_CURVE_WITH_KNOTS('',3,(#64046,#64047,#64048,#64049,#64050,
#64051,#64052,#64053,#64054,#64055,#64056),.UNSPECIFIED.,.F.,.F.,(4,1,1,
1,1,1,1,1,4),(323.584043319749,323.839822210921,324.837345499621,325.834868788321,
326.832392077021,327.829915365721,328.827438654421,329.824961943121,329.867228626928),
 .UNSPECIFIED.);
#1263=B_SPLINE_CURVE_WITH_KNOTS('',3,(#64057,#64058,#64059,#64060,#64061,
#64062,#64063,#64064,#64065,#64066),.UNSPECIFIED.,.F.,.F.,(4,1,1,1,1,1,
1,4),(323.584043319749,324.523266969986,325.520790258686,326.518313547386,
327.515836836086,328.513360124786,329.510883413486,329.867228626928),
 .UNSPECIFIED.);
#1264=B_SPLINE_CURVE_WITH_KNOTS('',3,(#64071,#64072,#64073,#64074,#64075,
#64076,#64077,#64078,#64079,#64080),.UNSPECIFIED.,.F.,.F.,(4,1,1,1,1,1,
1,4),(317.300858012569,317.854682478721,318.852205767421,319.849729056121,
320.847252344821,321.844775633521,322.842298922221,323.584043319749),
 .UNSPECIFIED.);
#1265=B_SPLINE_CURVE_WITH_KNOTS('',3,(#64081,#64082,#64083,#64084,#64085,
#64086,#64087,#64088,#64089,#64090,#64091),.UNSPECIFIED.,.F.,.F.,(4,1,1,
1,1,1,1,1,4),(317.300858012569,317.540603949086,318.538127237786,319.535650526486,
320.533173815186,321.530697103886,322.528220392586,323.525743681286,323.584043319749),
 .UNSPECIFIED.);
#1266=B_SPLINE_CURVE_WITH_KNOTS('',3,(#64096,#64097,#64098,#64099,#64100,
#64101,#64102,#64103,#64104,#64105),.UNSPECIFIED.,.F.,.F.,(4,1,1,1,1,1,
1,4),(311.01767270539,311.869542746521,312.867066035221,313.864589323921,
314.862112612621,315.859635901321,316.857159190021,317.300858012569),
 .UNSPECIFIED.);
#1267=B_SPLINE_CURVE_WITH_KNOTS('',3,(#64106,#64107,#64108,#64109,#64110,
#64111,#64112,#64113,#64114,#64115),.UNSPECIFIED.,.F.,.F.,(4,1,1,1,1,1,
1,4),(311.01767270539,311.555464216886,312.552987505586,313.550510794286,
314.548034082986,315.545557371686,316.543080660386,317.300858012569),
 .UNSPECIFIED.);
#1268=B_SPLINE_CURVE_WITH_KNOTS('',3,(#64120,#64121,#64122,#64123,#64124,
#64125,#64126,#64127,#64128,#64129,#64130),.UNSPECIFIED.,.F.,.F.,(4,1,1,
1,1,1,1,1,4),(304.73448739821,304.886879725621,305.884403014321,306.881926303021,
307.879449591721,308.876972880421,309.874496169121,310.872019457821,311.01767270539),
 .UNSPECIFIED.);
#1269=B_SPLINE_CURVE_WITH_KNOTS('',3,(#64131,#64132,#64133,#64134,#64135,
#64136,#64137,#64138,#64139,#64140),.UNSPECIFIED.,.F.,.F.,(4,1,1,1,1,1,
1,4),(304.73448739821,305.570324484686,306.567847773386,307.565371062086,
308.562894350786,309.560417639486,310.557940928186,311.01767270539),
 .UNSPECIFIED.);
#1270=B_SPLINE_CURVE_WITH_KNOTS('',3,(#64145,#64146,#64147,#64148,#64149,
#64150,#64151,#64152,#64153,#64154),.UNSPECIFIED.,.F.,.F.,(4,1,1,1,1,1,
1,4),(298.451302091031,298.901739993421,299.899263282121,300.896786570821,
301.894309859521,302.891833148221,303.889356436921,304.73448739821),
 .UNSPECIFIED.);
#1271=B_SPLINE_CURVE_WITH_KNOTS('',3,(#64155,#64156,#64157,#64158,#64159,
#64160,#64161,#64162,#64163,#64164,#64165),.UNSPECIFIED.,.F.,.F.,(4,1,1,
1,1,1,1,1,4),(298.451302091031,298.587661463786,299.585184752486,300.582708041186,
301.580231329886,302.577754618586,303.575277907286,304.572801195986,304.73448739821),
 .UNSPECIFIED.);
#1272=B_SPLINE_CURVE_WITH_KNOTS('',3,(#64170,#64171,#64172,#64173,#64174,
#64175,#64176,#64177,#64178,#64179),.UNSPECIFIED.,.F.,.F.,(4,1,1,1,1,1,
1,4),(292.168116783851,292.916600261221,293.914123549921,294.911646838621,
295.909170127321,296.906693416021,297.904216704721,298.451302091031),
 .UNSPECIFIED.);
#1273=B_SPLINE_CURVE_WITH_KNOTS('',3,(#64180,#64181,#64182,#64183,#64184,
#64185,#64186,#64187,#64188,#64189),.UNSPECIFIED.,.F.,.F.,(4,1,1,1,1,1,
1,4),(292.168116783851,292.602521731586,293.600045020286,294.597568308986,
295.595091597686,296.592614886386,297.590138175086,298.451302091031),
 .UNSPECIFIED.);
#1274=B_SPLINE_CURVE_WITH_KNOTS('',3,(#64194,#64195,#64196,#64197,#64198,
#64199,#64200,#64201,#64202,#64203,#64204),.UNSPECIFIED.,.F.,.F.,(4,1,1,
1,1,1,1,1,4),(285.884931476671,285.933937240321,286.931460529021,287.928983817721,
288.926507106421,289.924030395121,290.921553683821,291.919076972521,292.168116783851),
 .UNSPECIFIED.);
#1275=B_SPLINE_CURVE_WITH_KNOTS('',3,(#64205,#64206,#64207,#64208,#64209,
#64210,#64211,#64212,#64213,#64214),.UNSPECIFIED.,.F.,.F.,(4,1,1,1,1,1,
1,4),(285.884931476671,286.617381999385,287.614905288085,288.612428576785,
289.609951865485,290.607475154186,291.604998442886,292.168116783851),
 .UNSPECIFIED.);
#1276=B_SPLINE_CURVE_WITH_KNOTS('',3,(#64219,#64220,#64221,#64222,#64223,
#64224,#64225,#64226,#64227,#64228),.UNSPECIFIED.,.F.,.F.,(4,1,1,1,1,1,
1,4),(279.601746169492,279.948797508121,280.946320796821,281.943844085521,
282.941367374221,283.938890662921,284.936413951621,285.884931476671),
 .UNSPECIFIED.);
#1277=B_SPLINE_CURVE_WITH_KNOTS('',3,(#64229,#64230,#64231,#64232,#64233,
#64234,#64235,#64236,#64237,#64238,#64239),.UNSPECIFIED.,.F.,.F.,(4,1,1,
1,1,1,1,1,4),(279.601746169492,279.634718978485,280.632242267185,281.629765555885,
282.627288844585,283.624812133285,284.622335421985,285.619858710685,285.884931476671),
 .UNSPECIFIED.);
#1278=B_SPLINE_CURVE_WITH_KNOTS('',3,(#64244,#64245,#64246,#64247,#64248,
#64249,#64250,#64251,#64252,#64253),.UNSPECIFIED.,.F.,.F.,(4,1,1,1,1,1,
1,4),(273.318560862312,273.963657775921,274.961181064621,275.958704353321,
276.956227642021,277.953750930721,278.951274219421,279.601746169492),
 .UNSPECIFIED.);
#1279=B_SPLINE_CURVE_WITH_KNOTS('',3,(#64254,#64255,#64256,#64257,#64258,
#64259,#64260,#64261,#64262,#64263),.UNSPECIFIED.,.F.,.F.,(4,1,1,1,1,1,
1,4),(273.318560862312,273.649579246285,274.647102534985,275.644625823685,
276.642149112385,277.639672401085,278.637195689785,279.601746169492),
 .UNSPECIFIED.);
#1280=B_SPLINE_CURVE_WITH_KNOTS('',3,(#64268,#64269,#64270,#64271,#64272,
#64273,#64274,#64275,#64276,#64277),.UNSPECIFIED.,.F.,.F.,(4,1,1,1,1,1,
1,4),(267.035375555133,267.97851804372,268.97604133242,269.973564621121,
270.971087909821,271.968611198521,272.966134487221,273.318560862312),
 .UNSPECIFIED.);
#1281=B_SPLINE_CURVE_WITH_KNOTS('',3,(#64278,#64279,#64280,#64281,#64282,
#64283,#64284,#64285,#64286,#64287),.UNSPECIFIED.,.F.,.F.,(4,1,1,1,1,1,
1,4),(267.035375555133,267.664439514085,268.661962802785,269.659486091485,
270.657009380185,271.654532668885,272.652055957585,273.318560862312),
 .UNSPECIFIED.);
#1282=B_SPLINE_CURVE_WITH_KNOTS('',3,(#64292,#64293,#64294,#64295,#64296,
#64297,#64298,#64299,#64300,#64301,#64302),.UNSPECIFIED.,.F.,.F.,(4,1,1,
1,1,1,1,1,4),(260.752190247953,260.99585502282,261.99337831152,262.99090160022,
263.98842488892,264.98594817762,265.983471466321,266.980994755021,267.035375555133),
 .UNSPECIFIED.);
#1283=B_SPLINE_CURVE_WITH_KNOTS('',3,(#64303,#64304,#64305,#64306,#64307,
#64308,#64309,#64310,#64311,#64312),.UNSPECIFIED.,.F.,.F.,(4,1,1,1,1,1,
1,4),(260.752190247953,261.679299781885,262.676823070585,263.674346359285,
264.671869647985,265.669392936685,266.666916225385,267.035375555133),
 .UNSPECIFIED.);
#1284=B_SPLINE_CURVE_WITH_KNOTS('',3,(#64317,#64318,#64319,#64320,#64321,
#64322,#64323,#64324,#64325,#64326),.UNSPECIFIED.,.F.,.F.,(4,1,1,1,1,1,
1,4),(254.469004940774,255.01071529062,256.00823857932,257.00576186802,
258.00328515672,259.00080844542,259.99833173412,260.752190247953),
 .UNSPECIFIED.);
#1285=B_SPLINE_CURVE_WITH_KNOTS('',3,(#64327,#64328,#64329,#64330,#64331,
#64332,#64333,#64334,#64335,#64336,#64337),.UNSPECIFIED.,.F.,.F.,(4,1,1,
1,1,1,1,1,4),(254.469004940774,254.696636760985,255.694160049685,256.691683338385,
257.689206627085,258.686729915785,259.684253204485,260.681776493185,260.752190247953),
 .UNSPECIFIED.);
#1286=B_SPLINE_CURVE_WITH_KNOTS('',3,(#64342,#64343,#64344,#64345,#64346,
#64347,#64348,#64349,#64350,#64351),.UNSPECIFIED.,.F.,.F.,(4,1,1,1,1,1,
1,4),(248.185819633594,249.02557555842,250.02309884712,251.02062213582,
252.01814542452,253.01566871322,254.01319200192,254.469004940774),
 .UNSPECIFIED.);
#1287=B_SPLINE_CURVE_WITH_KNOTS('',3,(#64352,#64353,#64354,#64355,#64356,
#64357,#64358,#64359,#64360,#64361),.UNSPECIFIED.,.F.,.F.,(4,1,1,1,1,1,
1,4),(248.185819633594,248.711497028785,249.709020317485,250.706543606185,
251.704066894885,252.701590183585,253.699113472285,254.469004940774),
 .UNSPECIFIED.);
#1288=B_SPLINE_CURVE_WITH_KNOTS('',3,(#64366,#64367,#64368,#64369,#64370,
#64371,#64372,#64373,#64374,#64375,#64376),.UNSPECIFIED.,.F.,.F.,(4,1,1,
1,1,1,1,1,4),(241.902634326414,242.04291253752,243.04043582622,244.03795911492,
245.03548240362,246.03300569232,247.03052898102,248.02805226972,248.185819633594),
 .UNSPECIFIED.);
#1289=B_SPLINE_CURVE_WITH_KNOTS('',3,(#64377,#64378,#64379,#64380,#64381,
#64382,#64383,#64384,#64385,#64386),.UNSPECIFIED.,.F.,.F.,(4,1,1,1,1,1,
1,4),(241.902634326414,242.726357296585,243.723880585285,244.721403873985,
245.718927162685,246.716450451385,247.713973740085,248.185819633594),
 .UNSPECIFIED.);
#1290=B_SPLINE_CURVE_WITH_KNOTS('',3,(#64391,#64392,#64393,#64394,#64395,
#64396,#64397,#64398,#64399,#64400),.UNSPECIFIED.,.F.,.F.,(4,1,1,1,1,1,
1,4),(235.619449019235,236.05777280532,237.05529609402,238.05281938272,
239.05034267142,240.04786596012,241.04538924882,241.902634326414),
 .UNSPECIFIED.);
#1291=B_SPLINE_CURVE_WITH_KNOTS('',3,(#64401,#64402,#64403,#64404,#64405,
#64406,#64407,#64408,#64409,#64410,#64411),.UNSPECIFIED.,.F.,.F.,(4,1,1,
1,1,1,1,1,4),(235.619449019235,235.743694275685,236.741217564385,237.738740853085,
238.736264141785,239.733787430485,240.731310719185,241.728834007885,241.902634326414),
 .UNSPECIFIED.);
#1292=B_SPLINE_CURVE_WITH_KNOTS('',3,(#64416,#64417,#64418,#64419,#64420,
#64421,#64422,#64423,#64424,#64425),.UNSPECIFIED.,.F.,.F.,(4,1,1,1,1,1,
1,4),(229.336263712055,230.07263307312,231.07015636182,232.06767965052,
233.06520293922,234.06272622792,235.06024951662,235.619449019235),
 .UNSPECIFIED.);
#1293=B_SPLINE_CURVE_WITH_KNOTS('',3,(#64426,#64427,#64428,#64429,#64430,
#64431,#64432,#64433,#64434,#64435),.UNSPECIFIED.,.F.,.F.,(4,1,1,1,1,1,
1,4),(229.336263712055,229.758554543485,230.756077832185,231.753601120885,
232.751124409585,233.748647698285,234.746170986985,235.619449019235),
 .UNSPECIFIED.);
#1294=B_SPLINE_CURVE_WITH_KNOTS('',3,(#64440,#64441,#64442,#64443,#64444,
#64445,#64446,#64447,#64448,#64449,#64450),.UNSPECIFIED.,.F.,.F.,(4,1,1,
1,1,1,1,1,4),(223.053078404876,223.08997005222,224.08749334092,225.08501662962,
226.08253991832,227.08006320702,228.07758649572,229.07510978442,229.336263712055),
 .UNSPECIFIED.);
#1295=B_SPLINE_CURVE_WITH_KNOTS('',3,(#64451,#64452,#64453,#64454,#64455,
#64456,#64457,#64458,#64459,#64460),.UNSPECIFIED.,.F.,.F.,(4,1,1,1,1,1,
1,4),(223.053078404876,223.773414811285,224.770938099985,225.768461388685,
226.765984677385,227.763507966085,228.761031254785,229.336263712055),
 .UNSPECIFIED.);
#1296=B_SPLINE_CURVE_WITH_KNOTS('',3,(#64465,#64466,#64467,#64468,#64469,
#64470,#64471,#64472,#64473,#64474),.UNSPECIFIED.,.F.,.F.,(4,1,1,1,1,1,
1,4),(216.769893097696,217.10483032002,218.10235360872,219.09987689742,
220.09740018612,221.09492347482,222.09244676352,223.053078404876),
 .UNSPECIFIED.);
#1297=B_SPLINE_CURVE_WITH_KNOTS('',3,(#64475,#64476,#64477,#64478,#64479,
#64480,#64481,#64482,#64483,#64484,#64485),.UNSPECIFIED.,.F.,.F.,(4,1,1,
1,1,1,1,1,4),(216.769893097696,216.790751790385,217.788275079085,218.785798367785,
219.783321656485,220.780844945185,221.778368233885,222.775891522585,223.053078404876),
 .UNSPECIFIED.);
#1298=B_SPLINE_CURVE_WITH_KNOTS('',3,(#64490,#64491,#64492,#64493,#64494,
#64495,#64496,#64497,#64498,#64499),.UNSPECIFIED.,.F.,.F.,(4,1,1,1,1,1,
1,4),(210.486707790517,211.11969058782,212.11721387652,213.11473716522,
214.11226045392,215.10978374262,216.10730703132,216.769893097696),
 .UNSPECIFIED.);
#1299=B_SPLINE_CURVE_WITH_KNOTS('',3,(#64500,#64501,#64502,#64503,#64504,
#64505,#64506,#64507,#64508,#64509),.UNSPECIFIED.,.F.,.F.,(4,1,1,1,1,1,
1,4),(210.486707790517,210.805612058185,211.803135346885,212.800658635585,
213.798181924285,214.795705212985,215.793228501685,216.769893097696),
 .UNSPECIFIED.);
#1300=B_SPLINE_CURVE_WITH_KNOTS('',3,(#64514,#64515,#64516,#64517,#64518,
#64519,#64520,#64521,#64522,#64523),.UNSPECIFIED.,.F.,.F.,(4,1,1,1,1,1,
1,4),(204.203522483337,205.13455085562,206.13207414432,207.12959743302,
208.12712072172,209.12464401042,210.12216729912,210.486707790517),
 .UNSPECIFIED.);
#1301=B_SPLINE_CURVE_WITH_KNOTS('',3,(#64524,#64525,#64526,#64527,#64528,
#64529,#64530,#64531,#64532,#64533),.UNSPECIFIED.,.F.,.F.,(4,1,1,1,1,1,
1,4),(204.203522483337,204.820472325985,205.817995614685,206.815518903385,
207.813042192085,208.810565480785,209.808088769485,210.486707790517),
 .UNSPECIFIED.);
#1302=B_SPLINE_CURVE_WITH_KNOTS('',3,(#64538,#64539,#64540,#64541,#64542,
#64543,#64544,#64545,#64546,#64547,#64548),.UNSPECIFIED.,.F.,.F.,(4,1,1,
1,1,1,1,1,4),(197.920337176158,198.15188783472,199.14941112342,200.14693441212,
201.14445770082,202.14198098952,203.13950427822,204.13702756692,204.203522483337),
 .UNSPECIFIED.);
#1303=B_SPLINE_CURVE_WITH_KNOTS('',3,(#64549,#64550,#64551,#64552,#64553,
#64554,#64555,#64556,#64557,#64558),.UNSPECIFIED.,.F.,.F.,(4,1,1,1,1,1,
1,4),(197.920337176158,198.835332593785,199.832855882485,200.830379171185,
201.827902459885,202.825425748585,203.822949037285,204.203522483337),
 .UNSPECIFIED.);
#1304=B_SPLINE_CURVE_WITH_KNOTS('',3,(#64563,#64564,#64565,#64566,#64567,
#64568,#64569,#64570,#64571,#64572),.UNSPECIFIED.,.F.,.F.,(4,1,1,1,1,1,
1,4),(191.637151868978,192.16674810252,193.16427139122,194.16179467992,
195.15931796862,196.15684125732,197.15436454602,197.920337176158),
 .UNSPECIFIED.);
#1305=B_SPLINE_CURVE_WITH_KNOTS('',3,(#64573,#64574,#64575,#64576,#64577,
#64578,#64579,#64580,#64581,#64582,#64583),.UNSPECIFIED.,.F.,.F.,(4,1,1,
1,1,1,1,1,4),(191.637151868978,191.852669572885,192.850192861585,193.847716150285,
194.845239438985,195.842762727685,196.840286016385,197.837809305085,197.920337176158),
 .UNSPECIFIED.);
#1306=B_SPLINE_CURVE_WITH_KNOTS('',3,(#64588,#64589,#64590,#64591,#64592,
#64593,#64594,#64595,#64596,#64597),.UNSPECIFIED.,.F.,.F.,(4,1,1,1,1,1,
1,4),(185.353966561798,186.18160837032,187.17913165902,188.17665494772,
189.17417823642,190.17170152512,191.16922481382,191.637151868978),
 .UNSPECIFIED.);
#1307=B_SPLINE_CURVE_WITH_KNOTS('',3,(#64598,#64599,#64600,#64601,#64602,
#64603,#64604,#64605,#64606,#64607),.UNSPECIFIED.,.F.,.F.,(4,1,1,1,1,1,
1,4),(185.353966561798,185.867529840685,186.865053129385,187.862576418085,
188.860099706785,189.857622995485,190.855146284185,191.637151868978),
 .UNSPECIFIED.);
#1308=B_SPLINE_CURVE_WITH_KNOTS('',3,(#64612,#64613,#64614,#64615,#64616,
#64617,#64618,#64619,#64620,#64621,#64622),.UNSPECIFIED.,.F.,.F.,(4,1,1,
1,1,1,1,1,4),(179.070781254619,179.19894534942,180.19646863812,181.19399192682,
182.19151521552,183.18903850422,184.18656179292,185.18408508162,185.353966561798),
 .UNSPECIFIED.);
#1309=B_SPLINE_CURVE_WITH_KNOTS('',3,(#64623,#64624,#64625,#64626,#64627,
#64628,#64629,#64630,#64631,#64632),.UNSPECIFIED.,.F.,.F.,(4,1,1,1,1,1,
1,4),(179.070781254619,179.882390108485,180.879913397185,181.877436685885,
182.874959974585,183.872483263285,184.870006551985,185.353966561798),
 .UNSPECIFIED.);
#1310=B_SPLINE_CURVE_WITH_KNOTS('',3,(#64637,#64638,#64639,#64640,#64641,
#64642,#64643,#64644,#64645,#64646),.UNSPECIFIED.,.F.,.F.,(4,1,1,1,1,1,
1,4),(172.787595947439,173.21380561722,174.21132890592,175.20885219462,
176.20637548332,177.20389877202,178.20142206072,179.070781254619),
 .UNSPECIFIED.);
#1311=B_SPLINE_CURVE_WITH_KNOTS('',3,(#64647,#64648,#64649,#64650,#64651,
#64652,#64653,#64654,#64655,#64656,#64657),.UNSPECIFIED.,.F.,.F.,(4,1,1,
1,1,1,1,1,4),(172.787595947439,172.899727087585,173.897250376285,174.894773664985,
175.892296953685,176.889820242385,177.887343531085,178.884866819785,179.070781254619),
 .UNSPECIFIED.);
#1312=B_SPLINE_CURVE_WITH_KNOTS('',3,(#64662,#64663,#64664,#64665,#64666,
#64667,#64668,#64669,#64670,#64671),.UNSPECIFIED.,.F.,.F.,(4,1,1,1,1,1,
1,4),(166.50441064026,167.22866588502,168.22618917372,169.22371246242,170.22123575112,
171.21875903982,172.21628232852,172.787595947439),.UNSPECIFIED.);
#1313=B_SPLINE_CURVE_WITH_KNOTS('',3,(#64672,#64673,#64674,#64675,#64676,
#64677,#64678,#64679,#64680,#64681),.UNSPECIFIED.,.F.,.F.,(4,1,1,1,1,1,
1,4),(166.50441064026,166.914587355385,167.912110644085,168.909633932785,
169.907157221485,170.904680510185,171.902203798885,172.787595947439),
 .UNSPECIFIED.);
#1314=B_SPLINE_CURVE_WITH_KNOTS('',3,(#64686,#64687,#64688,#64689,#64690,
#64691,#64692,#64693,#64694,#64695,#64696),.UNSPECIFIED.,.F.,.F.,(4,1,1,
1,1,1,1,1,4),(160.22122533308,160.24600286412,161.24352615282,162.24104944152,
163.23857273022,164.23609601892,165.23361930762,166.23114259632,166.50441064026),
 .UNSPECIFIED.);
#1315=B_SPLINE_CURVE_WITH_KNOTS('',3,(#64697,#64698,#64699,#64700,#64701,
#64702,#64703,#64704,#64705,#64706),.UNSPECIFIED.,.F.,.F.,(4,1,1,1,1,1,
1,4),(160.22122533308,160.929447623185,161.926970911885,162.924494200585,
163.922017489285,164.919540777985,165.917064066685,166.50441064026),
 .UNSPECIFIED.);
#1316=B_SPLINE_CURVE_WITH_KNOTS('',3,(#64711,#64712,#64713,#64714,#64715,
#64716,#64717,#64718,#64719,#64720),.UNSPECIFIED.,.F.,.F.,(4,1,1,1,1,1,
1,4),(153.938040025901,154.26086313192,155.25838642062,156.25590970932,
157.25343299802,158.25095628672,159.24847957542,160.22122533308),
 .UNSPECIFIED.);
#1317=B_SPLINE_CURVE_WITH_KNOTS('',3,(#64721,#64722,#64723,#64724,#64725,
#64726,#64727,#64728,#64729,#64730,#64731),.UNSPECIFIED.,.F.,.F.,(4,1,1,
1,1,1,1,1,4),(153.938040025901,153.946784602285,154.944307890985,155.941831179685,
156.939354468385,157.936877757085,158.934401045785,159.931924334485,160.22122533308),
 .UNSPECIFIED.);
#1318=B_SPLINE_CURVE_WITH_KNOTS('',3,(#64736,#64737,#64738,#64739,#64740,
#64741,#64742,#64743,#64744,#64745),.UNSPECIFIED.,.F.,.F.,(4,1,1,1,1,1,
1,4),(147.654854718721,148.27572339972,149.27324668842,150.27076997712,
151.26829326582,152.26581655452,153.26333984322,153.938040025901),
 .UNSPECIFIED.);
#1319=B_SPLINE_CURVE_WITH_KNOTS('',3,(#64746,#64747,#64748,#64749,#64750,
#64751,#64752,#64753,#64754,#64755),.UNSPECIFIED.,.F.,.F.,(4,1,1,1,1,1,
1,4),(147.654854718721,147.961644870085,148.959168158785,149.956691447485,
150.954214736185,151.951738024885,152.949261313585,153.938040025901),
 .UNSPECIFIED.);
#1320=B_SPLINE_CURVE_WITH_KNOTS('',3,(#64760,#64761,#64762,#64763,#64764,
#64765,#64766,#64767,#64768,#64769),.UNSPECIFIED.,.F.,.F.,(4,1,1,1,1,1,
1,4),(141.371669411541,142.29058366752,143.28810695622,144.28563024492,
145.28315353362,146.28067682232,147.27820011102,147.654854718721),
 .UNSPECIFIED.);
#1321=B_SPLINE_CURVE_WITH_KNOTS('',3,(#64770,#64771,#64772,#64773,#64774,
#64775,#64776,#64777,#64778,#64779),.UNSPECIFIED.,.F.,.F.,(4,1,1,1,1,1,
1,4),(141.371669411541,141.976505137885,142.974028426585,143.971551715285,
144.969075003985,145.966598292685,146.964121581385,147.654854718721),
 .UNSPECIFIED.);
#1322=B_SPLINE_CURVE_WITH_KNOTS('',3,(#64784,#64785,#64786,#64787,#64788,
#64789,#64790,#64791,#64792,#64793,#64794),.UNSPECIFIED.,.F.,.F.,(4,1,1,
1,1,1,1,1,4),(135.088484104362,135.30792064662,136.30544393532,137.30296722402,
138.30049051272,139.29801380142,140.29553709012,141.29306037882,141.371669411541),
 .UNSPECIFIED.);
#1323=B_SPLINE_CURVE_WITH_KNOTS('',3,(#64795,#64796,#64797,#64798,#64799,
#64800,#64801,#64802,#64803,#64804),.UNSPECIFIED.,.F.,.F.,(4,1,1,1,1,1,
1,4),(135.088484104362,135.991365405685,136.988888694385,137.986411983085,
138.983935271785,139.981458560485,140.978981849185,141.371669411541),
 .UNSPECIFIED.);
#1324=B_SPLINE_CURVE_WITH_KNOTS('',3,(#64809,#64810,#64811,#64812,#64813,
#64814,#64815,#64816,#64817,#64818),.UNSPECIFIED.,.F.,.F.,(4,1,1,1,1,1,
1,4),(128.805298797182,129.32278091442,130.32030420312,131.31782749182,
132.31535078052,133.31287406922,134.31039735792,135.088484104362),
 .UNSPECIFIED.);
#1325=B_SPLINE_CURVE_WITH_KNOTS('',3,(#64819,#64820,#64821,#64822,#64823,
#64824,#64825,#64826,#64827,#64828,#64829),.UNSPECIFIED.,.F.,.F.,(4,1,1,
1,1,1,1,1,4),(128.805298797182,129.008702384785,130.006225673485,131.003748962185,
132.001272250885,132.998795539585,133.996318828285,134.993842116985,135.088484104362),
 .UNSPECIFIED.);
#1326=B_SPLINE_CURVE_WITH_KNOTS('',3,(#64834,#64835,#64836,#64837,#64838,
#64839,#64840,#64841,#64842,#64843),.UNSPECIFIED.,.F.,.F.,(4,1,1,1,1,1,
1,4),(122.522113490003,123.33764118222,124.33516447092,125.33268775962,
126.33021104832,127.32773433702,128.32525762572,128.805298797182),
 .UNSPECIFIED.);
#1327=B_SPLINE_CURVE_WITH_KNOTS('',3,(#64844,#64845,#64846,#64847,#64848,
#64849,#64850,#64851,#64852,#64853),.UNSPECIFIED.,.F.,.F.,(4,1,1,1,1,1,
1,4),(122.522113490003,123.023562652585,124.021085941285,125.018609229985,
126.016132518685,127.013655807385,128.011179096085,128.805298797182),
 .UNSPECIFIED.);
#1328=B_SPLINE_CURVE_WITH_KNOTS('',3,(#64858,#64859,#64860,#64861,#64862,
#64863,#64864,#64865,#64866,#64867,#64868),.UNSPECIFIED.,.F.,.F.,(4,1,1,
1,1,1,1,1,4),(116.238928182823,116.35497816132,117.35250145002,118.35002473872,
119.34754802742,120.34507131612,121.34259460482,122.34011789352,122.522113490003),
 .UNSPECIFIED.);
#1329=B_SPLINE_CURVE_WITH_KNOTS('',3,(#64869,#64870,#64871,#64872,#64873,
#64874,#64875,#64876,#64877,#64878),.UNSPECIFIED.,.F.,.F.,(4,1,1,1,1,1,
1,4),(116.238928182823,117.038422920385,118.035946209085,119.033469497785,
120.030992786485,121.028516075185,122.026039363885,122.522113490003),
 .UNSPECIFIED.);
#1330=B_SPLINE_CURVE_WITH_KNOTS('',3,(#64883,#64884,#64885,#64886,#64887,
#64888,#64889,#64890,#64891,#64892),.UNSPECIFIED.,.F.,.F.,(4,1,1,1,1,1,
1,4),(109.955742875644,110.36983842912,111.36736171782,112.36488500652,
113.36240829522,114.35993158392,115.35745487262,116.238928182823),
 .UNSPECIFIED.);
#1331=B_SPLINE_CURVE_WITH_KNOTS('',3,(#64893,#64894,#64895,#64896,#64897,
#64898,#64899,#64900,#64901,#64902,#64903),.UNSPECIFIED.,.F.,.F.,(4,1,1,
1,1,1,1,1,4),(109.955742875644,110.055759899484,111.053283188184,112.050806476884,
113.048329765584,114.045853054284,115.043376342985,116.040899631685,116.238928182823),
 .UNSPECIFIED.);
#1332=B_SPLINE_CURVE_WITH_KNOTS('',3,(#64908,#64909,#64910,#64911,#64912,
#64913,#64914,#64915,#64916,#64917),.UNSPECIFIED.,.F.,.F.,(4,1,1,1,1,1,
1,4),(103.672557568464,104.38469869692,105.38222198562,106.37974527432,
107.37726856302,108.37479185172,109.37231514042,109.955742875644),
 .UNSPECIFIED.);
#1333=B_SPLINE_CURVE_WITH_KNOTS('',3,(#64918,#64919,#64920,#64921,#64922,
#64923,#64924,#64925,#64926,#64927),.UNSPECIFIED.,.F.,.F.,(4,1,1,1,1,1,
1,4),(103.672557568464,104.070620167284,105.068143455984,106.065666744684,
107.063190033384,108.060713322084,109.058236610784,109.955742875644),
 .UNSPECIFIED.);
#1334=B_SPLINE_CURVE_WITH_KNOTS('',3,(#64932,#64933,#64934,#64935,#64936,
#64937,#64938,#64939,#64940,#64941,#64942),.UNSPECIFIED.,.F.,.F.,(4,1,1,
1,1,1,1,1,4),(97.3893722612843,97.4020356760196,98.3995589647196,99.3970822534196,
100.39460554212,101.39212883082,102.38965211952,103.38717540822,103.672557568464),
 .UNSPECIFIED.);
#1335=B_SPLINE_CURVE_WITH_KNOTS('',3,(#64943,#64944,#64945,#64946,#64947,
#64948,#64949,#64950,#64951,#64952),.UNSPECIFIED.,.F.,.F.,(4,1,1,1,1,1,
1,4),(97.3893722612844,98.0854804350844,99.0830037237844,100.080527012484,
101.078050301184,102.075573589884,103.073096878584,103.672557568464),
 .UNSPECIFIED.);
#1336=B_SPLINE_CURVE_WITH_KNOTS('',3,(#64957,#64958,#64959,#64960,#64961,
#64962,#64963,#64964,#64965,#64966),.UNSPECIFIED.,.F.,.F.,(4,1,1,1,1,1,
1,4),(91.1061869541047,91.4168959438195,92.4144192325195,93.4119425212196,
94.4094658099196,95.4069890986196,96.4045123873196,97.3893722612843),
 .UNSPECIFIED.);
#1337=B_SPLINE_CURVE_WITH_KNOTS('',3,(#64967,#64968,#64969,#64970,#64971,
#64972,#64973,#64974,#64975,#64976),.UNSPECIFIED.,.F.,.F.,(4,1,1,1,1,1,
1,4),(91.1061869541048,92.1003407028844,93.0978639915844,94.0953872802844,
95.0929105689844,96.0904338576844,97.0879571463844,97.3893722612844),
 .UNSPECIFIED.);
#1338=B_SPLINE_CURVE_WITH_KNOTS('',3,(#64981,#64982,#64983,#64984,#64985,
#64986,#64987,#64988,#64989,#64990),.UNSPECIFIED.,.F.,.F.,(4,1,1,1,1,1,
1,4),(84.8230016469251,85.4317562116195,86.4292795003195,87.4268027890195,
88.4243260777195,89.4218493664195,90.4193726551195,91.1061869541047),
 .UNSPECIFIED.);
#1339=B_SPLINE_CURVE_WITH_KNOTS('',3,(#64991,#64992,#64993,#64994,#64995,
#64996,#64997,#64998,#64999,#65000,#65001),.UNSPECIFIED.,.F.,.F.,(4,1,1,
1,1,1,1,1,4),(84.8230016469252,85.1176776819843,86.1152009706843,87.1127242593844,
88.1102475480844,89.1077708367844,90.1052941254844,91.1028174141844,91.1061869541048),
 .UNSPECIFIED.);
#1340=B_SPLINE_CURVE_WITH_KNOTS('',3,(#65006,#65007,#65008,#65009,#65010,
#65011,#65012,#65013,#65014,#65015),.UNSPECIFIED.,.F.,.F.,(4,1,1,1,1,1,
1,4),(78.5398163397455,79.4466164794195,80.4441397681195,81.4416630568195,
82.4391863455195,83.4367096342195,84.4342329229195,84.8230016469251),
 .UNSPECIFIED.);
#1341=B_SPLINE_CURVE_WITH_KNOTS('',3,(#65016,#65017,#65018,#65019,#65020,
#65021,#65022,#65023,#65024,#65025),.UNSPECIFIED.,.F.,.F.,(4,1,1,1,1,1,
1,4),(78.5398163397456,79.1325379497843,80.1300612384843,81.1275845271843,
82.1251078158843,83.1226311045843,84.1201543932843,84.8230016469252),
 .UNSPECIFIED.);
#1342=B_SPLINE_CURVE_WITH_KNOTS('',3,(#65030,#65031,#65032,#65033,#65034,
#65035,#65036,#65037,#65038,#65039,#65040),.UNSPECIFIED.,.F.,.F.,(4,1,1,
1,1,1,1,1,4),(72.2566310325659,72.4639534585194,73.4614767472195,74.4590000359194,
75.4565233246195,76.4540466133195,77.4515699020195,78.4490931907195,78.5398163397455),
 .UNSPECIFIED.);
#1343=B_SPLINE_CURVE_WITH_KNOTS('',3,(#65041,#65042,#65043,#65044,#65045,
#65046,#65047,#65048,#65049,#65050),.UNSPECIFIED.,.F.,.F.,(4,1,1,1,1,1,
1,4),(72.256631032566,73.1473982175843,74.1449215062843,75.1424447949843,
76.1399680836843,77.1374913723843,78.1350146610843,78.5398163397456),
 .UNSPECIFIED.);
#1344=B_SPLINE_CURVE_WITH_KNOTS('',3,(#65055,#65056,#65057,#65058,#65059,
#65060,#65061,#65062,#65063,#65064),.UNSPECIFIED.,.F.,.F.,(4,1,1,1,1,1,
1,4),(65.9734457253863,66.4788137263194,67.4763370150194,68.4738603037194,
69.4713835924194,70.4689068811194,71.4664301698194,72.2566310325659),
 .UNSPECIFIED.);
#1345=B_SPLINE_CURVE_WITH_KNOTS('',3,(#65065,#65066,#65067,#65068,#65069,
#65070,#65071,#65072,#65073,#65074,#65075),.UNSPECIFIED.,.F.,.F.,(4,1,1,
1,1,1,1,1,4),(65.9734457253864,66.1647351966842,67.1622584853842,68.1597817740843,
69.1573050627842,70.1548283514843,71.1523516401843,72.1498749288843,72.256631032566),
 .UNSPECIFIED.);
#1346=B_SPLINE_CURVE_WITH_KNOTS('',3,(#65080,#65081,#65082,#65083,#65084,
#65085,#65086,#65087,#65088,#65089),.UNSPECIFIED.,.F.,.F.,(4,1,1,1,1,1,
1,4),(59.6902604182067,60.4936739941194,61.4911972828194,62.4887205715194,
63.4862438602194,64.4837671489194,65.4812904376194,65.9734457253863),
 .UNSPECIFIED.);
#1347=B_SPLINE_CURVE_WITH_KNOTS('',3,(#65090,#65091,#65092,#65093,#65094,
#65095,#65096,#65097,#65098,#65099),.UNSPECIFIED.,.F.,.F.,(4,1,1,1,1,1,
1,4),(59.6902604182069,60.1795954644842,61.1771187531842,62.1746420418842,
63.1721653305842,64.1696886192842,65.1672119079842,65.9734457253864),
 .UNSPECIFIED.);
#1348=B_SPLINE_CURVE_WITH_KNOTS('',3,(#65104,#65105,#65106,#65107,#65108,
#65109,#65110,#65111,#65112,#65113,#65114),.UNSPECIFIED.,.F.,.F.,(4,1,1,
1,1,1,1,1,4),(53.4070751110272,53.5110109732193,54.5085342619193,55.5060575506193,
56.5035808393194,57.5011041280194,58.4986274167194,59.4961507054194,59.6902604182067),
 .UNSPECIFIED.);
#1349=B_SPLINE_CURVE_WITH_KNOTS('',3,(#65115,#65116,#65117,#65118,#65119,
#65120,#65121,#65122,#65123,#65124),.UNSPECIFIED.,.F.,.F.,(4,1,1,1,1,1,
1,4),(53.4070751110273,54.1944557322842,55.1919790209842,56.1895023096842,
57.1870255983842,58.1845488870842,59.1820721757842,59.6902604182069),
 .UNSPECIFIED.);
#1350=B_SPLINE_CURVE_WITH_KNOTS('',3,(#65129,#65130,#65131,#65132,#65133,
#65134,#65135,#65136,#65137,#65138),.UNSPECIFIED.,.F.,.F.,(4,1,1,1,1,1,
1,4),(47.1238898038476,47.5258712410193,48.5233945297193,49.5209178184193,
50.5184411071193,51.5159643958193,52.5134876845193,53.4070751110272),
 .UNSPECIFIED.);
#1351=B_SPLINE_CURVE_WITH_KNOTS('',3,(#65139,#65140,#65141,#65142,#65143,
#65144,#65145,#65146,#65147,#65148,#65149),.UNSPECIFIED.,.F.,.F.,(4,1,1,
1,1,1,1,1,4),(47.1238898038477,47.2117927113841,48.2093160000841,49.2068392887841,
50.2043625774841,51.2018858661842,52.1994091548842,53.1969324435842,53.4070751110273),
 .UNSPECIFIED.);
#1352=B_SPLINE_CURVE_WITH_KNOTS('',3,(#65154,#65155,#65156,#65157,#65158,
#65159,#65160,#65161,#65162,#65163),.UNSPECIFIED.,.F.,.F.,(4,1,1,1,1,1,
1,4),(40.840704496668,41.5407315088193,42.5382547975193,43.5357780862193,
44.5333013749193,45.5308246636193,46.5283479523193,47.1238898038476),
 .UNSPECIFIED.);
#1353=B_SPLINE_CURVE_WITH_KNOTS('',3,(#65164,#65165,#65166,#65167,#65168,
#65169,#65170,#65171,#65172,#65173),.UNSPECIFIED.,.F.,.F.,(4,1,1,1,1,1,
1,4),(40.8407044966681,41.2266529791841,42.2241762678841,43.2216995565841,
44.2192228452841,45.2167461339841,46.2142694226841,47.1238898038477),
 .UNSPECIFIED.);
#1354=B_SPLINE_CURVE_WITH_KNOTS('',3,(#65178,#65179,#65180,#65181,#65182,
#65183,#65184,#65185,#65186,#65187,#65188),.UNSPECIFIED.,.F.,.F.,(4,1,1,
1,1,1,1,1,4),(34.5575191894884,34.5580684879192,35.5555917766192,36.5531150653192,
37.5506383540192,38.5481616427193,39.5456849314193,40.5432082201193,40.840704496668),
 .UNSPECIFIED.);
#1355=B_SPLINE_CURVE_WITH_KNOTS('',3,(#65189,#65190,#65191,#65192,#65193,
#65194,#65195,#65196,#65197,#65198),.UNSPECIFIED.,.F.,.F.,(4,1,1,1,1,1,
1,4),(34.5575191894885,35.2415132469841,36.2390365356841,37.2365598243841,
38.2340831130841,39.2316064017841,40.2291296904841,40.8407044966681),
 .UNSPECIFIED.);
#1356=B_SPLINE_CURVE_WITH_KNOTS('',3,(#65203,#65204,#65205,#65206,#65207,
#65208,#65209,#65210,#65211,#65212),.UNSPECIFIED.,.F.,.F.,(4,1,1,1,1,1,
1,4),(28.2743338823088,28.5729287557192,29.5704520444192,30.5679753331192,
31.5654986218192,32.5630219105192,33.5605451992192,34.5575191894884),
 .UNSPECIFIED.);
#1357=B_SPLINE_CURVE_WITH_KNOTS('',3,(#65213,#65214,#65215,#65216,#65217,
#65218,#65219,#65220,#65221,#65222),.UNSPECIFIED.,.F.,.F.,(4,1,1,1,1,1,
1,4),(28.2743338823089,29.256373514784,30.253896803484,31.251420092184,
32.2489433808841,33.2464666695841,34.2439899582841,34.5575191894885),
 .UNSPECIFIED.);
#1358=B_SPLINE_CURVE_WITH_KNOTS('',3,(#65227,#65228,#65229,#65230,#65231,
#65232,#65233,#65234,#65235,#65236),.UNSPECIFIED.,.F.,.F.,(4,1,1,1,1,1,
1,4),(21.9911485751292,22.5877890235192,23.5853123122192,24.5828356009192,
25.5803588896192,26.5778821783192,27.5754054670192,28.2743338823088),
 .UNSPECIFIED.);
#1359=B_SPLINE_CURVE_WITH_KNOTS('',3,(#65237,#65238,#65239,#65240,#65241,
#65242,#65243,#65244,#65245,#65246,#65247),.UNSPECIFIED.,.F.,.F.,(4,1,1,
1,1,1,1,1,4),(21.9911485751293,22.273710493884,23.271233782584,24.268757071284,
25.266280359984,26.263803648684,27.261326937384,28.258850226084,28.2743338823089),
 .UNSPECIFIED.);
#1360=B_SPLINE_CURVE_WITH_KNOTS('',3,(#65252,#65253,#65254,#65255,#65256,
#65257,#65258,#65259,#65260,#65261),.UNSPECIFIED.,.F.,.F.,(4,1,1,1,1,1,
1,4),(15.7079632679496,16.6026492913191,17.6001725800191,18.5976958687191,
19.5952191574192,20.5927424461192,21.5902657348192,21.9911485751292),
 .UNSPECIFIED.);
#1361=B_SPLINE_CURVE_WITH_KNOTS('',3,(#65262,#65263,#65264,#65265,#65266,
#65267,#65268,#65269,#65270,#65271),.UNSPECIFIED.,.F.,.F.,(4,1,1,1,1,1,
1,4),(15.7079632679497,16.288570761684,17.286094050384,18.283617339084,
19.281140627784,20.278663916484,21.276187205184,21.9911485751293),
 .UNSPECIFIED.);
#1362=B_SPLINE_CURVE_WITH_KNOTS('',3,(#66813,#66814,#66815,#66816,#66817,
#66818,#66819,#66820,#66821,#66822,#66823,#66824,#66825,#66826,#66827,#66828,
#66829,#66830,#66831,#66832,#66833,#66834,#66835,#66836,#66837,#66838,#66839,
#66840,#66841,#66842,#66843,#66844,#66845,#66846,#66847,#66848,#66849,#66850,
#66851,#66852,#66853,#66854,#66855,#66856,#66857,#66858,#66859,#66860,#66861,
#66862,#66863,#66864,#66865,#66866,#66867,#66868,#66869,#66870,#66871,#66872,
#66873,#66874,#66875,#66876,#66877,#66878,#66879,#66880,#66881,#66882,#66883,
#66884,#66885,#66886,#66887,#66888,#66889,#66890,#66891,#66892,#66893,#66894,
#66895,#66896,#66897,#66898,#66899,#66900,#66901,#66902,#66903,#66904,#66905,
#66906,#66907,#66908,#66909,#66910,#66911,#66912,#66913,#66914,#66915,#66916,
#66917,#66918,#66919,#66920,#66921),.UNSPECIFIED.,.F.,.F.,(4,3,3,3,3,3,
3,3,3,3,3,3,3,3,3,3,3,3,3,3,3,3,3,3,3,3,3,3,3,3,3,3,3,3,3,3,4),(0.,0.0359628151845056,
0.0790640675124802,0.122944974172411,0.167078080679047,0.180430545026742,
0.19037773183983,0.196180338284082,0.239492682886256,0.282925566791464,
0.325969530232972,0.368238370501489,0.375078460706215,0.381042467863404,
0.42346125387141,0.465393907031249,0.506323913773678,0.51599109870151,0.544714566753401,
0.554178082246963,0.559723896450525,0.565364051500323,0.606359797650403,
0.648015429264718,0.689524423166306,0.717651633141474,0.732581126571207,
0.739096451862393,0.745778843116641,0.786822056096576,0.827804944486442,
0.845389038445888,0.853674880949773,0.860823772315063,0.901249933519242,
0.94103892518765,0.96847769616201),.UNSPECIFIED.);
#1363=B_SPLINE_CURVE_WITH_KNOTS('',3,(#66922,#66923,#66924,#66925,#66926,
#66927,#66928,#66929,#66930,#66931,#66932,#66933,#66934,#66935,#66936,#66937,
#66938,#66939,#66940),.UNSPECIFIED.,.F.,.F.,(4,3,3,3,3,3,4),(371.824326632282,
372.076186685102,373.073709973802,374.071233262502,375.068756551202,376.066279839902,
376.991118430775),.UNSPECIFIED.);
#1364=B_SPLINE_CURVE_WITH_KNOTS('',3,(#66942,#66943,#66944,#66945,#66946,
#66947,#66948,#66949,#66950,#66951,#66952,#66953,#66954,#66955,#66956,#66957,
#66958,#66959,#66960,#66961,#66962,#66963,#66964,#66965,#66966,#66967,#66968,
#66969,#66970,#66971,#66972,#66973,#66974,#66975,#66976,#66977,#66978,#66979,
#66980,#66981,#66982,#66983,#66984,#66985,#66986,#66987,#66988,#66989,#66990,
#66991,#66992,#66993,#66994,#66995,#66996,#66997,#66998,#66999,#67000,#67001,
#67002,#67003,#67004,#67005,#67006,#67007,#67008,#67009,#67010,#67011,#67012,
#67013,#67014,#67015,#67016,#67017,#67018,#67019,#67020,#67021,#67022,#67023,
#67024,#67025,#67026,#67027,#67028,#67029,#67030,#67031,#67032,#67033,#67034,
#67035,#67036,#67037,#67038,#67039,#67040,#67041,#67042,#67043,#67044,#67045,
#67046,#67047),.UNSPECIFIED.,.F.,.F.,(4,3,3,3,3,3,3,3,3,3,3,3,3,3,3,3,3,
3,3,3,3,3,3,3,3,3,3,3,3,3,3,3,3,3,3,4),(-0.968477696161913,-0.936462781732006,
-0.897034237282827,-0.871088158002514,-0.855755616551603,-0.849836345176422,
-0.809673382933614,-0.76870133116664,-0.750776058518589,-0.741856737530979,
-0.7341371378361,-0.692655598295136,-0.650704137993651,-0.608502345694694,
-0.576851001470477,-0.56347054188062,-0.556078670388381,-0.513475355214464,
-0.481896968797825,-0.440388916382611,-0.398291621794682,-0.386095361159993,
-0.379050278062876,-0.373539380612515,-0.331389873213074,-0.287819274607371,
-0.244248676001668,-0.213717591501459,-0.200360242032618,-0.19269654176718,
-0.1869673316623,-0.143586522253231,-0.0997397595963603,-0.0560111116848197,
-0.0129407155146067,0.),.UNSPECIFIED.);
#1365=B_SPLINE_CURVE_WITH_KNOTS('',3,(#67048,#67049,#67050,#67051,#67052,
#67053,#67054,#67055,#67056),.UNSPECIFIED.,.F.,.F.,(4,1,1,1,1,1,4),(10.3761157273111,
11.3009543181839,12.2984776068839,13.2960008955839,14.2935241842839,15.291047472984,
15.7079632679497),.UNSPECIFIED.);
#1366=B_SPLINE_CURVE_WITH_KNOTS('',3,(#67060,#67061,#67062,#67063,#67064,
#67065,#67066,#67067,#67068),.UNSPECIFIED.,.F.,.F.,(4,1,1,1,1,1,4),(11.6150328478191,
12.1137944921691,12.6125561365191,13.6100794252191,14.6076027139191,15.6051260026191,
15.7079632679496),.UNSPECIFIED.);
#1367=B_SPLINE_CURVE_WITH_KNOTS('',3,(#68610,#68611,#68612,#68613,#68614,
#68615,#68616,#68617,#68618,#68619,#68620,#68621,#68622,#68623,#68624,#68625,
#68626,#68627,#68628,#68629,#68630,#68631,#68632,#68633,#68634,#68635,#68636,
#68637,#68638,#68639,#68640,#68641,#68642,#68643,#68644,#68645,#68646,#68647,
#68648,#68649,#68650,#68651,#68652,#68653,#68654,#68655,#68656,#68657,#68658,
#68659,#68660,#68661,#68662,#68663,#68664,#68665,#68666,#68667,#68668,#68669,
#68670,#68671,#68672,#68673,#68674,#68675,#68676,#68677,#68678,#68679,#68680,
#68681,#68682,#68683,#68684,#68685,#68686,#68687,#68688,#68689,#68690,#68691,
#68692,#68693,#68694,#68695,#68696,#68697,#68698,#68699,#68700,#68701,#68702,
#68703,#68704,#68705,#68706,#68707,#68708,#68709,#68710,#68711,#68712,#68713,
#68714,#68715,#68716,#68717,#68718),.UNSPECIFIED.,.F.,.F.,(4,3,3,3,3,3,
3,3,3,3,3,3,3,3,3,3,3,3,3,3,3,3,3,3,3,3,3,3,3,3,3,3,3,3,3,3,4),(0.,0.0319610084124964,
0.0709970802367925,0.110918019903594,0.151489267836741,0.166268550959158,
0.172136820332691,0.17773227169752,0.218621519728627,0.260105203172031,
0.301749535598996,0.343042584632714,0.348577800050639,0.354310610465885,
0.396643769367683,0.438881645932778,0.480394489143215,0.485838103022159,
0.515447494563868,0.527322668925359,0.533096841618444,0.574119197999633,
0.616402831080215,0.659075854182062,0.69089454476895,0.706803890062393,
0.714443723340302,0.720575125052056,0.722713235355837,0.765747942600601,
0.80908641486819,0.828699390062085,0.838036583520388,0.844245630783005,
0.888067982944121,0.931632292905962,0.965990216419354),.UNSPECIFIED.);
#1368=B_SPLINE_CURVE_WITH_KNOTS('',3,(#68719,#68720,#68721,#68722,#68723,
#68724,#68725,#68726,#68727,#68728,#68729,#68730,#68731,#68732,#68733,#68734,
#68735,#68736,#68737,#68738,#68739,#68740,#68741,#68742,#68743,#68744,#68745,
#68746,#68747,#68748,#68749,#68750,#68751,#68752,#68753,#68754,#68755,#68756,
#68757,#68758,#68759,#68760,#68761,#68762,#68763,#68764,#68765,#68766,#68767,
#68768,#68769,#68770,#68771,#68772,#68773,#68774,#68775,#68776,#68777,#68778,
#68779,#68780,#68781,#68782,#68783,#68784,#68785,#68786,#68787,#68788,#68789,
#68790,#68791,#68792,#68793,#68794,#68795,#68796,#68797,#68798,#68799,#68800,
#68801,#68802,#68803,#68804,#68805,#68806,#68807,#68808,#68809,#68810,#68811,
#68812,#68813,#68814,#68815,#68816,#68817,#68818,#68819,#68820,#68821),
 .UNSPECIFIED.,.F.,.F.,(4,3,3,3,3,3,3,3,3,3,3,3,3,3,3,3,3,3,3,3,3,3,3,3,
3,3,3,3,3,3,3,3,3,3,4),(-0.965990216419533,-0.930132396483882,-0.886600314752691,
-0.859427241407658,-0.844575649172136,-0.83450269382505,-0.791217440053876,
-0.748794152701163,-0.730233964484351,-0.71490535117285,-0.708744621568391,
-0.665691199232105,-0.622727628938354,-0.580003507011809,-0.5479604155669,
-0.535021607402038,-0.529041072836267,-0.487381790675506,-0.451831141232172,
-0.409951411560376,-0.367982065107459,-0.353448430125576,-0.345247061313217,
-0.304116472475951,-0.262917042414806,-0.222498465588061,-0.194686157389553,
-0.181409937644946,-0.17316340151046,-0.167260443835079,-0.125445332876309,
-0.0850027204681986,-0.0449509623998064,-0.00571310113625183,0.),
 .UNSPECIFIED.);
#1369=B_SPLINE_CURVE_WITH_KNOTS('',3,(#68822,#68823,#68824,#68825,#68826,
#68827,#68828,#68829,#68830,#68831,#68832,#68833,#68834,#68835,#68836,#68837,
#68838,#68839,#68840),.UNSPECIFIED.,.F.,.F.,(4,3,3,3,3,3,4),(-379.058849706002,
-378.560088061652,-378.061326417302,-377.063803128602,-376.066279839902,
-375.068756551202,-374.800863543725),.UNSPECIFIED.);
#2223=SHAPE_REPRESENTATION_RELATIONSHIP('SRR','None',#97617,#2242);
#2242=ADVANCED_BREP_SHAPE_REPRESENTATION('',(#2280),#97467);
#2261=STYLED_ITEM('',(#97723),#2280);
#2280=MANIFOLD_SOLID_BREP('Body1',#21822);
#2353=FACE_BOUND('',#4430,.T.);
#2354=FACE_BOUND('',#4432,.T.);
#2488=PLANE('',#22936);
#2489=PLANE('',#22937);
#2490=PLANE('',#22939);
#2491=PLANE('',#22940);
#2492=PLANE('',#22941);
#2493=PLANE('',#22942);
#2494=PLANE('',#22943);
#2495=PLANE('',#22944);
#2496=PLANE('',#22947);
#3086=FACE_OUTER_BOUND('',#4305,.T.);
#3087=FACE_OUTER_BOUND('',#4306,.T.);
#3088=FACE_OUTER_BOUND('',#4307,.T.);
#3089=FACE_OUTER_BOUND('',#4308,.T.);
#3090=FACE_OUTER_BOUND('',#4309,.T.);
#3091=FACE_OUTER_BOUND('',#4310,.T.);
#3092=FACE_OUTER_BOUND('',#4311,.T.);
#3093=FACE_OUTER_BOUND('',#4312,.T.);
#3094=FACE_OUTER_BOUND('',#4313,.T.);
#3095=FACE_OUTER_BOUND('',#4314,.T.);
#3096=FACE_OUTER_BOUND('',#4315,.T.);
#3097=FACE_OUTER_BOUND('',#4316,.T.);
#3098=FACE_OUTER_BOUND('',#4317,.T.);
#3099=FACE_OUTER_BOUND('',#4318,.T.);
#3100=FACE_OUTER_BOUND('',#4319,.T.);
#3101=FACE_OUTER_BOUND('',#4320,.T.);
#3102=FACE_OUTER_BOUND('',#4321,.T.);
#3103=FACE_OUTER_BOUND('',#4322,.T.);
#3104=FACE_OUTER_BOUND('',#4323,.T.);
#3105=FACE_OUTER_BOUND('',#4324,.T.);
#3106=FACE_OUTER_BOUND('',#4325,.T.);
#3107=FACE_OUTER_BOUND('',#4326,.T.);
#3108=FACE_OUTER_BOUND('',#4327,.T.);
#3109=FACE_OUTER_BOUND('',#4328,.T.);
#3110=FACE_OUTER_BOUND('',#4329,.T.);
#3111=FACE_OUTER_BOUND('',#4330,.T.);
#3112=FACE_OUTER_BOUND('',#4331,.T.);
#3113=FACE_OUTER_BOUND('',#4332,.T.);
#3114=FACE_OUTER_BOUND('',#4333,.T.);
#3115=FACE_OUTER_BOUND('',#4334,.T.);
#3116=FACE_OUTER_BOUND('',#4335,.T.);
#3117=FACE_OUTER_BOUND('',#4336,.T.);
#3118=FACE_OUTER_BOUND('',#4337,.T.);
#3119=FACE_OUTER_BOUND('',#4338,.T.);
#3120=FACE_OUTER_BOUND('',#4339,.T.);
#3121=FACE_OUTER_BOUND('',#4340,.T.);
#3122=FACE_OUTER_BOUND('',#4341,.T.);
#3123=FACE_OUTER_BOUND('',#4342,.T.);
#3124=FACE_OUTER_BOUND('',#4343,.T.);
#3125=FACE_OUTER_BOUND('',#4344,.T.);
#3126=FACE_OUTER_BOUND('',#4345,.T.);
#3127=FACE_OUTER_BOUND('',#4346,.T.);
#3128=FACE_OUTER_BOUND('',#4347,.T.);
#3129=FACE_OUTER_BOUND('',#4348,.T.);
#3130=FACE_OUTER_BOUND('',#4349,.T.);
#3131=FACE_OUTER_BOUND('',#4350,.T.);
#3132=FACE_OUTER_BOUND('',#4351,.T.);
#3133=FACE_OUTER_BOUND('',#4352,.T.);
#3134=FACE_OUTER_BOUND('',#4353,.T.);
#3135=FACE_OUTER_BOUND('',#4354,.T.);
#3136=FACE_OUTER_BOUND('',#4355,.T.);
#3137=FACE_OUTER_BOUND('',#4356,.T.);
#3138=FACE_OUTER_BOUND('',#4357,.T.);
#3139=FACE_OUTER_BOUND('',#4358,.T.);
#3140=FACE_OUTER_BOUND('',#4359,.T.);
#3141=FACE_OUTER_BOUND('',#4360,.T.);
#3142=FACE_OUTER_BOUND('',#4361,.T.);
#3143=FACE_OUTER_BOUND('',#4362,.T.);
#3144=FACE_OUTER_BOUND('',#4363,.T.);
#3145=FACE_OUTER_BOUND('',#4364,.T.);
#3146=FACE_OUTER_BOUND('',#4365,.T.);
#3147=FACE_OUTER_BOUND('',#4366,.T.);
#3148=FACE_OUTER_BOUND('',#4367,.T.);
#3149=FACE_OUTER_BOUND('',#4368,.T.);
#3150=FACE_OUTER_BOUND('',#4369,.T.);
#3151=FACE_OUTER_BOUND('',#4370,.T.);
#3152=FACE_OUTER_BOUND('',#4371,.T.);
#3153=FACE_OUTER_BOUND('',#4372,.T.);
#3154=FACE_OUTER_BOUND('',#4373,.T.);
#3155=FACE_OUTER_BOUND('',#4374,.T.);
#3156=FACE_OUTER_BOUND('',#4375,.T.);
#3157=FACE_OUTER_BOUND('',#4376,.T.);
#3158=FACE_OUTER_BOUND('',#4377,.T.);
#3159=FACE_OUTER_BOUND('',#4378,.T.);
#3160=FACE_OUTER_BOUND('',#4379,.T.);
#3161=FACE_OUTER_BOUND('',#4380,.T.);
#3162=FACE_OUTER_BOUND('',#4381,.T.);
#3163=FACE_OUTER_BOUND('',#4382,.T.);
#3164=FACE_OUTER_BOUND('',#4383,.T.);
#3165=FACE_OUTER_BOUND('',#4384,.T.);
#3166=FACE_OUTER_BOUND('',#4385,.T.);
#3167=FACE_OUTER_BOUND('',#4386,.T.);
#3168=FACE_OUTER_BOUND('',#4387,.T.);
#3169=FACE_OUTER_BOUND('',#4388,.T.);
#3170=FACE_OUTER_BOUND('',#4389,.T.);
#3171=FACE_OUTER_BOUND('',#4390,.T.);
#3172=FACE_OUTER_BOUND('',#4391,.T.);
#3173=FACE_OUTER_BOUND('',#4392,.T.);
#3174=FACE_OUTER_BOUND('',#4393,.T.);
#3175=FACE_OUTER_BOUND('',#4394,.T.);
#3176=FACE_OUTER_BOUND('',#4395,.T.);
#3177=FACE_OUTER_BOUND('',#4396,.T.);
#3178=FACE_OUTER_BOUND('',#4397,.T.);
#3179=FACE_OUTER_BOUND('',#4398,.T.);
#3180=FACE_OUTER_BOUND('',#4399,.T.);
#3181=FACE_OUTER_BOUND('',#4400,.T.);
#3182=FACE_OUTER_BOUND('',#4401,.T.);
#3183=FACE_OUTER_BOUND('',#4402,.T.);
#3184=FACE_OUTER_BOUND('',#4403,.T.);
#3185=FACE_OUTER_BOUND('',#4404,.T.);
#3186=FACE_OUTER_BOUND('',#4405,.T.);
#3187=FACE_OUTER_BOUND('',#4406,.T.);
#3188=FACE_OUTER_BOUND('',#4407,.T.);
#3189=FACE_OUTER_BOUND('',#4408,.T.);
#3190=FACE_OUTER_BOUND('',#4409,.T.);
#3191=FACE_OUTER_BOUND('',#4410,.T.);
#3192=FACE_OUTER_BOUND('',#4411,.T.);
#3193=FACE_OUTER_BOUND('',#4412,.T.);
#3194=FACE_OUTER_BOUND('',#4413,.T.);
#3195=FACE_OUTER_BOUND('',#4414,.T.);
#3196=FACE_OUTER_BOUND('',#4415,.T.);
#3197=FACE_OUTER_BOUND('',#4416,.T.);
#3198=FACE_OUTER_BOUND('',#4417,.T.);
#3199=FACE_OUTER_BOUND('',#4418,.T.);
#3200=FACE_OUTER_BOUND('',#4419,.T.);
#3201=FACE_OUTER_BOUND('',#4420,.T.);
#3202=FACE_OUTER_BOUND('',#4421,.T.);
#3203=FACE_OUTER_BOUND('',#4422,.T.);
#3204=FACE_OUTER_BOUND('',#4423,.T.);
#3205=FACE_OUTER_BOUND('',#4424,.T.);
#3206=FACE_OUTER_BOUND('',#4425,.T.);
#3207=FACE_OUTER_BOUND('',#4426,.T.);
#3208=FACE_OUTER_BOUND('',#4427,.T.);
#3209=FACE_OUTER_BOUND('',#4428,.T.);
#3210=FACE_OUTER_BOUND('',#4429,.T.);
#3211=FACE_OUTER_BOUND('',#4431,.T.);
#3212=FACE_OUTER_BOUND('',#4433,.T.);
#3213=FACE_OUTER_BOUND('',#4434,.T.);
#3214=FACE_OUTER_BOUND('',#4435,.T.);
#3215=FACE_OUTER_BOUND('',#4436,.T.);
#3216=FACE_OUTER_BOUND('',#4437,.T.);
#3217=FACE_OUTER_BOUND('',#4438,.T.);
#3218=FACE_OUTER_BOUND('',#4439,.T.);
#3219=FACE_OUTER_BOUND('',#4440,.T.);
#3220=FACE_OUTER_BOUND('',#4441,.T.);
#4305=EDGE_LOOP('',(#16210,#16211,#16212,#16213));
#4306=EDGE_LOOP('',(#16214,#16215,#16216,#16217));
#4307=EDGE_LOOP('',(#16218,#16219,#16220,#16221));
#4308=EDGE_LOOP('',(#16222,#16223,#16224,#16225));
#4309=EDGE_LOOP('',(#16226,#16227,#16228,#16229));
#4310=EDGE_LOOP('',(#16230,#16231,#16232,#16233));
#4311=EDGE_LOOP('',(#16234,#16235,#16236,#16237));
#4312=EDGE_LOOP('',(#16238,#16239,#16240,#16241));
#4313=EDGE_LOOP('',(#16242,#16243,#16244,#16245));
#4314=EDGE_LOOP('',(#16246,#16247,#16248,#16249));
#4315=EDGE_LOOP('',(#16250,#16251,#16252,#16253));
#4316=EDGE_LOOP('',(#16254,#16255,#16256,#16257));
#4317=EDGE_LOOP('',(#16258,#16259,#16260,#16261));
#4318=EDGE_LOOP('',(#16262,#16263,#16264,#16265));
#4319=EDGE_LOOP('',(#16266,#16267,#16268,#16269));
#4320=EDGE_LOOP('',(#16270,#16271,#16272,#16273));
#4321=EDGE_LOOP('',(#16274,#16275,#16276,#16277));
#4322=EDGE_LOOP('',(#16278,#16279,#16280,#16281));
#4323=EDGE_LOOP('',(#16282,#16283,#16284,#16285));
#4324=EDGE_LOOP('',(#16286,#16287,#16288,#16289));
#4325=EDGE_LOOP('',(#16290,#16291,#16292,#16293));
#4326=EDGE_LOOP('',(#16294,#16295,#16296,#16297));
#4327=EDGE_LOOP('',(#16298,#16299,#16300,#16301));
#4328=EDGE_LOOP('',(#16302,#16303,#16304,#16305));
#4329=EDGE_LOOP('',(#16306,#16307,#16308,#16309));
#4330=EDGE_LOOP('',(#16310,#16311,#16312,#16313));
#4331=EDGE_LOOP('',(#16314,#16315,#16316,#16317));
#4332=EDGE_LOOP('',(#16318,#16319,#16320,#16321));
#4333=EDGE_LOOP('',(#16322,#16323,#16324,#16325));
#4334=EDGE_LOOP('',(#16326,#16327,#16328,#16329));
#4335=EDGE_LOOP('',(#16330,#16331,#16332,#16333));
#4336=EDGE_LOOP('',(#16334,#16335,#16336,#16337));
#4337=EDGE_LOOP('',(#16338,#16339,#16340,#16341));
#4338=EDGE_LOOP('',(#16342,#16343,#16344,#16345));
#4339=EDGE_LOOP('',(#16346,#16347,#16348,#16349));
#4340=EDGE_LOOP('',(#16350,#16351,#16352,#16353));
#4341=EDGE_LOOP('',(#16354,#16355,#16356,#16357));
#4342=EDGE_LOOP('',(#16358,#16359,#16360,#16361));
#4343=EDGE_LOOP('',(#16362,#16363,#16364,#16365));
#4344=EDGE_LOOP('',(#16366,#16367,#16368,#16369));
#4345=EDGE_LOOP('',(#16370,#16371,#16372,#16373));
#4346=EDGE_LOOP('',(#16374,#16375,#16376,#16377));
#4347=EDGE_LOOP('',(#16378,#16379,#16380,#16381));
#4348=EDGE_LOOP('',(#16382,#16383,#16384,#16385));
#4349=EDGE_LOOP('',(#16386,#16387,#16388,#16389));
#4350=EDGE_LOOP('',(#16390,#16391,#16392,#16393));
#4351=EDGE_LOOP('',(#16394,#16395,#16396,#16397));
#4352=EDGE_LOOP('',(#16398,#16399,#16400,#16401));
#4353=EDGE_LOOP('',(#16402,#16403,#16404,#16405));
#4354=EDGE_LOOP('',(#16406,#16407,#16408,#16409));
#4355=EDGE_LOOP('',(#16410,#16411,#16412,#16413));
#4356=EDGE_LOOP('',(#16414,#16415,#16416,#16417));
#4357=EDGE_LOOP('',(#16418,#16419,#16420,#16421));
#4358=EDGE_LOOP('',(#16422,#16423,#16424,#16425));
#4359=EDGE_LOOP('',(#16426,#16427,#16428,#16429));
#4360=EDGE_LOOP('',(#16430,#16431,#16432,#16433));
#4361=EDGE_LOOP('',(#16434,#16435,#16436,#16437));
#4362=EDGE_LOOP('',(#16438,#16439,#16440,#16441));
#4363=EDGE_LOOP('',(#16442,#16443,#16444,#16445));
#4364=EDGE_LOOP('',(#16446,#16447,#16448,#16449));
#4365=EDGE_LOOP('',(#16450,#16451,#16452,#16453));
#4366=EDGE_LOOP('',(#16454,#16455,#16456,#16457));
#4367=EDGE_LOOP('',(#16458,#16459,#16460,#16461));
#4368=EDGE_LOOP('',(#16462,#16463,#16464,#16465));
#4369=EDGE_LOOP('',(#16466,#16467,#16468,#16469));
#4370=EDGE_LOOP('',(#16470,#16471,#16472,#16473));
#4371=EDGE_LOOP('',(#16474,#16475,#16476,#16477));
#4372=EDGE_LOOP('',(#16478,#16479,#16480,#16481));
#4373=EDGE_LOOP('',(#16482,#16483,#16484,#16485));
#4374=EDGE_LOOP('',(#16486,#16487,#16488,#16489));
#4375=EDGE_LOOP('',(#16490,#16491,#16492,#16493));
#4376=EDGE_LOOP('',(#16494,#16495,#16496,#16497));
#4377=EDGE_LOOP('',(#16498,#16499,#16500,#16501));
#4378=EDGE_LOOP('',(#16502,#16503,#16504,#16505));
#4379=EDGE_LOOP('',(#16506,#16507,#16508,#16509));
#4380=EDGE_LOOP('',(#16510,#16511,#16512,#16513));
#4381=EDGE_LOOP('',(#16514,#16515,#16516,#16517));
#4382=EDGE_LOOP('',(#16518,#16519,#16520,#16521));
#4383=EDGE_LOOP('',(#16522,#16523,#16524,#16525));
#4384=EDGE_LOOP('',(#16526,#16527,#16528,#16529));
#4385=EDGE_LOOP('',(#16530,#16531,#16532,#16533));
#4386=EDGE_LOOP('',(#16534,#16535,#16536,#16537));
#4387=EDGE_LOOP('',(#16538,#16539,#16540,#16541));
#4388=EDGE_LOOP('',(#16542,#16543,#16544,#16545));
#4389=EDGE_LOOP('',(#16546,#16547,#16548,#16549));
#4390=EDGE_LOOP('',(#16550,#16551,#16552,#16553));
#4391=EDGE_LOOP('',(#16554,#16555,#16556,#16557));
#4392=EDGE_LOOP('',(#16558,#16559,#16560,#16561));
#4393=EDGE_LOOP('',(#16562,#16563,#16564,#16565));
#4394=EDGE_LOOP('',(#16566,#16567,#16568,#16569));
#4395=EDGE_LOOP('',(#16570,#16571,#16572,#16573));
#4396=EDGE_LOOP('',(#16574,#16575,#16576,#16577));
#4397=EDGE_LOOP('',(#16578,#16579,#16580,#16581));
#4398=EDGE_LOOP('',(#16582,#16583,#16584,#16585));
#4399=EDGE_LOOP('',(#16586,#16587,#16588,#16589));
#4400=EDGE_LOOP('',(#16590,#16591,#16592,#16593));
#4401=EDGE_LOOP('',(#16594,#16595,#16596,#16597));
#4402=EDGE_LOOP('',(#16598,#16599,#16600,#16601));
#4403=EDGE_LOOP('',(#16602,#16603,#16604,#16605));
#4404=EDGE_LOOP('',(#16606,#16607,#16608,#16609));
#4405=EDGE_LOOP('',(#16610,#16611,#16612,#16613));
#4406=EDGE_LOOP('',(#16614,#16615,#16616,#16617));
#4407=EDGE_LOOP('',(#16618,#16619,#16620,#16621));
#4408=EDGE_LOOP('',(#16622,#16623,#16624,#16625));
#4409=EDGE_LOOP('',(#16626,#16627,#16628,#16629));
#4410=EDGE_LOOP('',(#16630,#16631,#16632,#16633));
#4411=EDGE_LOOP('',(#16634,#16635,#16636,#16637));
#4412=EDGE_LOOP('',(#16638,#16639,#16640,#16641));
#4413=EDGE_LOOP('',(#16642,#16643,#16644,#16645));
#4414=EDGE_LOOP('',(#16646,#16647,#16648,#16649));
#4415=EDGE_LOOP('',(#16650,#16651,#16652,#16653));
#4416=EDGE_LOOP('',(#16654,#16655,#16656,#16657));
#4417=EDGE_LOOP('',(#16658,#16659,#16660,#16661));
#4418=EDGE_LOOP('',(#16662,#16663,#16664,#16665));
#4419=EDGE_LOOP('',(#16666,#16667,#16668,#16669));
#4420=EDGE_LOOP('',(#16670,#16671,#16672,#16673));
#4421=EDGE_LOOP('',(#16674,#16675,#16676,#16677));
#4422=EDGE_LOOP('',(#16678,#16679,#16680,#16681));
#4423=EDGE_LOOP('',(#16682,#16683,#16684,#16685));
#4424=EDGE_LOOP('',(#16686,#16687,#16688,#16689));
#4425=EDGE_LOOP('',(#16690,#16691,#16692,#16693,#16694,#16695,#16696,#16697,
#16698,#16699,#16700,#16701,#16702,#16703,#16704,#16705,#16706,#16707,#16708,
#16709,#16710,#16711,#16712,#16713,#16714,#16715,#16716,#16717,#16718,#16719,
#16720,#16721,#16722,#16723,#16724,#16725,#16726,#16727,#16728,#16729,#16730,
#16731,#16732,#16733,#16734,#16735,#16736,#16737,#16738,#16739,#16740,#16741,
#16742,#16743,#16744,#16745,#16746,#16747,#16748,#16749,#16750,#16751,#16752,
#16753,#16754,#16755,#16756,#16757,#16758,#16759,#16760,#16761,#16762,#16763,
#16764,#16765,#16766,#16767,#16768,#16769,#16770,#16771,#16772,#16773,#16774,
#16775,#16776,#16777,#16778,#16779,#16780,#16781,#16782,#16783,#16784,#16785,
#16786,#16787,#16788,#16789,#16790,#16791,#16792,#16793,#16794,#16795,#16796,
#16797,#16798,#16799,#16800,#16801,#16802,#16803,#16804,#16805,#16806,#16807,
#16808,#16809,#16810,#16811,#16812,#16813));
#4426=EDGE_LOOP('',(#16814,#16815,#16816,#16817));
#4427=EDGE_LOOP('',(#16818,#16819,#16820,#16821,#16822,#16823,#16824,#16825,
#16826,#16827,#16828,#16829,#16830,#16831,#16832,#16833,#16834,#16835,#16836,
#16837,#16838,#16839,#16840,#16841,#16842,#16843,#16844,#16845,#16846,#16847,
#16848,#16849,#16850,#16851,#16852,#16853,#16854,#16855,#16856,#16857,#16858,
#16859,#16860,#16861,#16862,#16863,#16864,#16865,#16866,#16867,#16868,#16869,
#16870,#16871,#16872,#16873,#16874,#16875,#16876,#16877,#16878,#16879,#16880,
#16881,#16882,#16883,#16884,#16885,#16886,#16887,#16888,#16889,#16890,#16891,
#16892,#16893,#16894,#16895,#16896,#16897,#16898,#16899,#16900,#16901,#16902,
#16903,#16904,#16905,#16906,#16907,#16908,#16909,#16910,#16911,#16912,#16913,
#16914,#16915,#16916,#16917,#16918,#16919,#16920,#16921,#16922,#16923,#16924,
#16925,#16926,#16927,#16928,#16929,#16930,#16931,#16932,#16933,#16934,#16935,
#16936,#16937,#16938,#16939,#16940,#16941));
#4428=EDGE_LOOP('',(#16942,#16943,#16944,#16945));
#4429=EDGE_LOOP('',(#16946,#16947,#16948,#16949,#16950,#16951));
#4430=EDGE_LOOP('',(#16952,#16953,#16954,#16955));
#4431=EDGE_LOOP('',(#16956,#16957,#16958,#16959,#16960,#16961));
#4432=EDGE_LOOP('',(#16962));
#4433=EDGE_LOOP('',(#16963,#16964,#16965,#16966));
#4434=EDGE_LOOP('',(#16967,#16968,#16969,#16970));
#4435=EDGE_LOOP('',(#16971,#16972,#16973,#16974));
#4436=EDGE_LOOP('',(#16975,#16976,#16977,#16978));
#4437=EDGE_LOOP('',(#16979,#16980,#16981,#16982));
#4438=EDGE_LOOP('',(#16983,#16984,#16985,#16986));
#4439=EDGE_LOOP('',(#16987,#16988,#16989,#16990));
#4440=EDGE_LOOP('',(#16991,#16992,#16993,#16994));
#4441=EDGE_LOOP('',(#16995,#16996,#16997));
#5551=LINE('',#60848,#6765);
#5552=LINE('',#60875,#6766);
#5553=LINE('',#60923,#6767);
#5554=LINE('',#60971,#6768);
#5555=LINE('',#61022,#6769);
#5556=LINE('',#61070,#6770);
#5557=LINE('',#61118,#6771);
#5558=LINE('',#61166,#6772);
#5559=LINE('',#61220,#6773);
#5560=LINE('',#61268,#6774);
#5561=LINE('',#61316,#6775);
#5562=LINE('',#61370,#6776);
#5563=LINE('',#61418,#6777);
#5564=LINE('',#61466,#6778);
#5565=LINE('',#61517,#6779);
#5566=LINE('',#61568,#6780);
#5567=LINE('',#61616,#6781);
#5568=LINE('',#61664,#6782);
#5569=LINE('',#61718,#6783);
#5570=LINE('',#61766,#6784);
#5571=LINE('',#61814,#6785);
#5572=LINE('',#61868,#6786);
#5573=LINE('',#61916,#6787);
#5574=LINE('',#61964,#6788);
#5575=LINE('',#62012,#6789);
#5576=LINE('',#62066,#6790);
#5577=LINE('',#62114,#6791);
#5578=LINE('',#62162,#6792);
#5579=LINE('',#62216,#6793);
#5580=LINE('',#62264,#6794);
#5581=LINE('',#62312,#6795);
#5582=LINE('',#62366,#6796);
#5583=LINE('',#62414,#6797);
#5584=LINE('',#62462,#6798);
#5585=LINE('',#62510,#6799);
#5586=LINE('',#62564,#6800);
#5587=LINE('',#62612,#6801);
#5588=LINE('',#62660,#6802);
#5589=LINE('',#62714,#6803);
#5590=LINE('',#62762,#6804);
#5591=LINE('',#62810,#6805);
#5592=LINE('',#62864,#6806);
#5593=LINE('',#62912,#6807);
#5594=LINE('',#62960,#6808);
#5595=LINE('',#63008,#6809);
#5596=LINE('',#63062,#6810);
#5597=LINE('',#63110,#6811);
#5598=LINE('',#63158,#6812);
#5599=LINE('',#63212,#6813);
#5600=LINE('',#63260,#6814);
#5601=LINE('',#63308,#6815);
#5602=LINE('',#63362,#6816);
#5603=LINE('',#63410,#6817);
#5604=LINE('',#63458,#6818);
#5605=LINE('',#63506,#6819);
#5606=LINE('',#63560,#6820);
#5607=LINE('',#63608,#6821);
#5608=LINE('',#63656,#6822);
#5609=LINE('',#63710,#6823);
#5610=LINE('',#63758,#6824);
#5611=LINE('',#63806,#6825);
#5612=LINE('',#63824,#6826);
#5613=LINE('',#63849,#6827);
#5614=LINE('',#63873,#6828);
#5615=LINE('',#63898,#6829);
#5616=LINE('',#63923,#6830);
#5617=LINE('',#63947,#6831);
#5618=LINE('',#63972,#6832);
#5619=LINE('',#63997,#6833);
#5620=LINE('',#64021,#6834);
#5621=LINE('',#64045,#6835);
#5622=LINE('',#64070,#6836);
#5623=LINE('',#64095,#6837);
#5624=LINE('',#64119,#6838);
#5625=LINE('',#64144,#6839);
#5626=LINE('',#64169,#6840);
#5627=LINE('',#64193,#6841);
#5628=LINE('',#64218,#6842);
#5629=LINE('',#64243,#6843);
#5630=LINE('',#64267,#6844);
#5631=LINE('',#64291,#6845);
#5632=LINE('',#64316,#6846);
#5633=LINE('',#64341,#6847);
#5634=LINE('',#64365,#6848);
#5635=LINE('',#64390,#6849);
#5636=LINE('',#64415,#6850);
#5637=LINE('',#64439,#6851);
#5638=LINE('',#64464,#6852);
#5639=LINE('',#64489,#6853);
#5640=LINE('',#64513,#6854);
#5641=LINE('',#64537,#6855);
#5642=LINE('',#64562,#6856);
#5643=LINE('',#64587,#6857);
#5644=LINE('',#64611,#6858);
#5645=LINE('',#64636,#6859);
#5646=LINE('',#64661,#6860);
#5647=LINE('',#64685,#6861);
#5648=LINE('',#64710,#6862);
#5649=LINE('',#64735,#6863);
#5650=LINE('',#64759,#6864);
#5651=LINE('',#64783,#6865);
#5652=LINE('',#64808,#6866);
#5653=LINE('',#64833,#6867);
#5654=LINE('',#64857,#6868);
#5655=LINE('',#64882,#6869);
#5656=LINE('',#64907,#6870);
#5657=LINE('',#64931,#6871);
#5658=LINE('',#64956,#6872);
#5659=LINE('',#64980,#6873);
#5660=LINE('',#65005,#6874);
#5661=LINE('',#65029,#6875);
#5662=LINE('',#65054,#6876);
#5663=LINE('',#65079,#6877);
#5664=LINE('',#65103,#6878);
#5665=LINE('',#65128,#6879);
#5666=LINE('',#65153,#6880);
#5667=LINE('',#65177,#6881);
#5668=LINE('',#65202,#6882);
#5669=LINE('',#65226,#6883);
#5670=LINE('',#65251,#6884);
#5671=LINE('',#68846,#6885);
#5672=LINE('',#68848,#6886);
#5673=LINE('',#68850,#6887);
#5674=LINE('',#68852,#6888);
#5675=LINE('',#68854,#6889);
#5676=LINE('',#68855,#6890);
#5677=LINE('',#68859,#6891);
#5678=LINE('',#68861,#6892);
#5679=LINE('',#68863,#6893);
#5680=LINE('',#68865,#6894);
#5681=LINE('',#68867,#6895);
#5682=LINE('',#68868,#6896);
#5683=LINE('',#68872,#6897);
#5684=LINE('',#68873,#6898);
#5685=LINE('',#68875,#6899);
#5686=LINE('',#68877,#6900);
#5687=LINE('',#68879,#6901);
#5688=LINE('',#68881,#6902);
#5689=LINE('',#68885,#6903);
#6765=VECTOR('',#25659,5.);
#6766=VECTOR('',#25664,5.);
#6767=VECTOR('',#25667,5.);
#6768=VECTOR('',#25670,5.);
#6769=VECTOR('',#25673,5.);
#6770=VECTOR('',#25676,5.);
#6771=VECTOR('',#25679,5.);
#6772=VECTOR('',#25682,5.);
#6773=VECTOR('',#25685,5.);
#6774=VECTOR('',#25688,5.);
#6775=VECTOR('',#25691,5.);
#6776=VECTOR('',#25694,5.);
#6777=VECTOR('',#25697,5.);
#6778=VECTOR('',#25700,5.);
#6779=VECTOR('',#25703,5.);
#6780=VECTOR('',#25706,5.);
#6781=VECTOR('',#25709,5.);
#6782=VECTOR('',#25712,5.);
#6783=VECTOR('',#25715,5.);
#6784=VECTOR('',#25718,5.);
#6785=VECTOR('',#25721,5.);
#6786=VECTOR('',#25724,5.);
#6787=VECTOR('',#25727,5.);
#6788=VECTOR('',#25730,5.);
#6789=VECTOR('',#25733,5.);
#6790=VECTOR('',#25736,5.);
#6791=VECTOR('',#25739,5.);
#6792=VECTOR('',#25742,5.);
#6793=VECTOR('',#25745,5.);
#6794=VECTOR('',#25748,5.);
#6795=VECTOR('',#25751,5.);
#6796=VECTOR('',#25754,5.);
#6797=VECTOR('',#25757,5.);
#6798=VECTOR('',#25760,5.);
#6799=VECTOR('',#25763,5.);
#6800=VECTOR('',#25766,5.);
#6801=VECTOR('',#25769,5.);
#6802=VECTOR('',#25772,5.);
#6803=VECTOR('',#25775,5.);
#6804=VECTOR('',#25778,5.);
#6805=VECTOR('',#25781,5.);
#6806=VECTOR('',#25784,5.);
#6807=VECTOR('',#25787,5.);
#6808=VECTOR('',#25790,5.);
#6809=VECTOR('',#25793,5.);
#6810=VECTOR('',#25796,5.);
#6811=VECTOR('',#25799,5.);
#6812=VECTOR('',#25802,5.);
#6813=VECTOR('',#25805,5.);
#6814=VECTOR('',#25808,5.);
#6815=VECTOR('',#25811,5.);
#6816=VECTOR('',#25814,5.);
#6817=VECTOR('',#25817,5.);
#6818=VECTOR('',#25820,5.);
#6819=VECTOR('',#25823,5.);
#6820=VECTOR('',#25826,5.);
#6821=VECTOR('',#25829,5.);
#6822=VECTOR('',#25832,5.);
#6823=VECTOR('',#25835,5.);
#6824=VECTOR('',#25838,5.);
#6825=VECTOR('',#25841,4.372);
#6826=VECTOR('',#25846,4.372);
#6827=VECTOR('',#25849,4.372);
#6828=VECTOR('',#25852,4.372);
#6829=VECTOR('',#25855,4.372);
#6830=VECTOR('',#25858,4.372);
#6831=VECTOR('',#25861,4.372);
#6832=VECTOR('',#25864,4.372);
#6833=VECTOR('',#25867,4.372);
#6834=VECTOR('',#25870,4.372);
#6835=VECTOR('',#25873,4.372);
#6836=VECTOR('',#25876,4.372);
#6837=VECTOR('',#25879,4.372);
#6838=VECTOR('',#25882,4.372);
#6839=VECTOR('',#25885,4.372);
#6840=VECTOR('',#25888,4.372);
#6841=VECTOR('',#25891,4.372);
#6842=VECTOR('',#25894,4.372);
#6843=VECTOR('',#25897,4.372);
#6844=VECTOR('',#25900,4.372);
#6845=VECTOR('',#25903,4.372);
#6846=VECTOR('',#25906,4.372);
#6847=VECTOR('',#25909,4.372);
#6848=VECTOR('',#25912,4.372);
#6849=VECTOR('',#25915,4.372);
#6850=VECTOR('',#25918,4.372);
#6851=VECTOR('',#25921,4.372);
#6852=VECTOR('',#25924,4.372);
#6853=VECTOR('',#25927,4.372);
#6854=VECTOR('',#25930,4.372);
#6855=VECTOR('',#25933,4.372);
#6856=VECTOR('',#25936,4.372);
#6857=VECTOR('',#25939,4.372);
#6858=VECTOR('',#25942,4.372);
#6859=VECTOR('',#25945,4.372);
#6860=VECTOR('',#25948,4.372);
#6861=VECTOR('',#25951,4.372);
#6862=VECTOR('',#25954,4.372);
#6863=VECTOR('',#25957,4.372);
#6864=VECTOR('',#25960,4.372);
#6865=VECTOR('',#25963,4.372);
#6866=VECTOR('',#25966,4.372);
#6867=VECTOR('',#25969,4.372);
#6868=VECTOR('',#25972,4.372);
#6869=VECTOR('',#25975,4.372);
#6870=VECTOR('',#25978,4.372);
#6871=VECTOR('',#25981,4.372);
#6872=VECTOR('',#25984,4.372);
#6873=VECTOR('',#25987,4.372);
#6874=VECTOR('',#25990,4.372);
#6875=VECTOR('',#25993,4.372);
#6876=VECTOR('',#25996,4.372);
#6877=VECTOR('',#25999,4.372);
#6878=VECTOR('',#26002,4.372);
#6879=VECTOR('',#26005,4.372);
#6880=VECTOR('',#26008,4.372);
#6881=VECTOR('',#26011,4.372);
#6882=VECTOR('',#26014,4.372);
#6883=VECTOR('',#26017,4.372);
#6884=VECTOR('',#26020,4.372);
#6885=VECTOR('',#26031,10.);
#6886=VECTOR('',#26032,10.);
#6887=VECTOR('',#26033,10.);
#6888=VECTOR('',#26034,10.);
#6889=VECTOR('',#26035,10.);
#6890=VECTOR('',#26036,10.);
#6891=VECTOR('',#26039,10.);
#6892=VECTOR('',#26040,10.);
#6893=VECTOR('',#26041,10.);
#6894=VECTOR('',#26042,10.);
#6895=VECTOR('',#26043,10.);
#6896=VECTOR('',#26044,10.);
#6897=VECTOR('',#26049,10.);
#6898=VECTOR('',#26050,10.);
#6899=VECTOR('',#26053,10.);
#6900=VECTOR('',#26056,10.);
#6901=VECTOR('',#26059,10.);
#6902=VECTOR('',#26062,10.);
#6903=VECTOR('',#26067,5.);
#7552=CIRCLE('',#22811,4.942);
#7553=CIRCLE('',#22872,4.372);
#7554=CIRCLE('',#22933,4.372);
#7555=CIRCLE('',#22935,4.942);
#7556=CIRCLE('',#22938,5.);
#7557=CIRCLE('',#22946,5.);
#7558=CIRCLE('',#22949,6.);
#8646=VERTEX_POINT('',#60846);
#8647=VERTEX_POINT('',#60847);
#8648=VERTEX_POINT('',#60849);
#8649=VERTEX_POINT('',#60860);
#8650=VERTEX_POINT('',#60873);
#8651=VERTEX_POINT('',#60874);
#8652=VERTEX_POINT('',#60921);
#8653=VERTEX_POINT('',#60922);
#8654=VERTEX_POINT('',#60969);
#8655=VERTEX_POINT('',#60970);
#8656=VERTEX_POINT('',#61020);
#8657=VERTEX_POINT('',#61021);
#8658=VERTEX_POINT('',#61068);
#8659=VERTEX_POINT('',#61069);
#8660=VERTEX_POINT('',#61116);
#8661=VERTEX_POINT('',#61117);
#8662=VERTEX_POINT('',#61164);
#8663=VERTEX_POINT('',#61165);
#8664=VERTEX_POINT('',#61218);
#8665=VERTEX_POINT('',#61219);
#8666=VERTEX_POINT('',#61266);
#8667=VERTEX_POINT('',#61267);
#8668=VERTEX_POINT('',#61314);
#8669=VERTEX_POINT('',#61315);
#8670=VERTEX_POINT('',#61368);
#8671=VERTEX_POINT('',#61369);
#8672=VERTEX_POINT('',#61416);
#8673=VERTEX_POINT('',#61417);
#8674=VERTEX_POINT('',#61464);
#8675=VERTEX_POINT('',#61465);
#8676=VERTEX_POINT('',#61515);
#8677=VERTEX_POINT('',#61516);
#8678=VERTEX_POINT('',#61566);
#8679=VERTEX_POINT('',#61567);
#8680=VERTEX_POINT('',#61614);
#8681=VERTEX_POINT('',#61615);
#8682=VERTEX_POINT('',#61662);
#8683=VERTEX_POINT('',#61663);
#8684=VERTEX_POINT('',#61716);
#8685=VERTEX_POINT('',#61717);
#8686=VERTEX_POINT('',#61764);
#8687=VERTEX_POINT('',#61765);
#8688=VERTEX_POINT('',#61812);
#8689=VERTEX_POINT('',#61813);
#8690=VERTEX_POINT('',#61866);
#8691=VERTEX_POINT('',#61867);
#8692=VERTEX_POINT('',#61914);
#8693=VERTEX_POINT('',#61915);
#8694=VERTEX_POINT('',#61962);
#8695=VERTEX_POINT('',#61963);
#8696=VERTEX_POINT('',#62010);
#8697=VERTEX_POINT('',#62011);
#8698=VERTEX_POINT('',#62064);
#8699=VERTEX_POINT('',#62065);
#8700=VERTEX_POINT('',#62112);
#8701=VERTEX_POINT('',#62113);
#8702=VERTEX_POINT('',#62160);
#8703=VERTEX_POINT('',#62161);
#8704=VERTEX_POINT('',#62214);
#8705=VERTEX_POINT('',#62215);
#8706=VERTEX_POINT('',#62262);
#8707=VERTEX_POINT('',#62263);
#8708=VERTEX_POINT('',#62310);
#8709=VERTEX_POINT('',#62311);
#8710=VERTEX_POINT('',#62364);
#8711=VERTEX_POINT('',#62365);
#8712=VERTEX_POINT('',#62412);
#8713=VERTEX_POINT('',#62413);
#8714=VERTEX_POINT('',#62460);
#8715=VERTEX_POINT('',#62461);
#8716=VERTEX_POINT('',#62508);
#8717=VERTEX_POINT('',#62509);
#8718=VERTEX_POINT('',#62562);
#8719=VERTEX_POINT('',#62563);
#8720=VERTEX_POINT('',#62610);
#8721=VERTEX_POINT('',#62611);
#8722=VERTEX_POINT('',#62658);
#8723=VERTEX_POINT('',#62659);
#8724=VERTEX_POINT('',#62712);
#8725=VERTEX_POINT('',#62713);
#8726=VERTEX_POINT('',#62760);
#8727=VERTEX_POINT('',#62761);
#8728=VERTEX_POINT('',#62808);
#8729=VERTEX_POINT('',#62809);
#8730=VERTEX_POINT('',#62862);
#8731=VERTEX_POINT('',#62863);
#8732=VERTEX_POINT('',#62910);
#8733=VERTEX_POINT('',#62911);
#8734=VERTEX_POINT('',#62958);
#8735=VERTEX_POINT('',#62959);
#8736=VERTEX_POINT('',#63006);
#8737=VERTEX_POINT('',#63007);
#8738=VERTEX_POINT('',#63060);
#8739=VERTEX_POINT('',#63061);
#8740=VERTEX_POINT('',#63108);
#8741=VERTEX_POINT('',#63109);
#8742=VERTEX_POINT('',#63156);
#8743=VERTEX_POINT('',#63157);
#8744=VERTEX_POINT('',#63210);
#8745=VERTEX_POINT('',#63211);
#8746=VERTEX_POINT('',#63258);
#8747=VERTEX_POINT('',#63259);
#8748=VERTEX_POINT('',#63306);
#8749=VERTEX_POINT('',#63307);
#8750=VERTEX_POINT('',#63360);
#8751=VERTEX_POINT('',#63361);
#8752=VERTEX_POINT('',#63408);
#8753=VERTEX_POINT('',#63409);
#8754=VERTEX_POINT('',#63456);
#8755=VERTEX_POINT('',#63457);
#8756=VERTEX_POINT('',#63504);
#8757=VERTEX_POINT('',#63505);
#8758=VERTEX_POINT('',#63558);
#8759=VERTEX_POINT('',#63559);
#8760=VERTEX_POINT('',#63606);
#8761=VERTEX_POINT('',#63607);
#8762=VERTEX_POINT('',#63654);
#8763=VERTEX_POINT('',#63655);
#8764=VERTEX_POINT('',#63708);
#8765=VERTEX_POINT('',#63709);
#8766=VERTEX_POINT('',#63756);
#8767=VERTEX_POINT('',#63757);
#8768=VERTEX_POINT('',#63804);
#8769=VERTEX_POINT('',#63805);
#8770=VERTEX_POINT('',#63807);
#8771=VERTEX_POINT('',#63814);
#8772=VERTEX_POINT('',#63822);
#8773=VERTEX_POINT('',#63823);
#8774=VERTEX_POINT('',#63847);
#8775=VERTEX_POINT('',#63848);
#8776=VERTEX_POINT('',#63871);
#8777=VERTEX_POINT('',#63872);
#8778=VERTEX_POINT('',#63896);
#8779=VERTEX_POINT('',#63897);
#8780=VERTEX_POINT('',#63921);
#8781=VERTEX_POINT('',#63922);
#8782=VERTEX_POINT('',#63945);
#8783=VERTEX_POINT('',#63946);
#8784=VERTEX_POINT('',#63970);
#8785=VERTEX_POINT('',#63971);
#8786=VERTEX_POINT('',#63995);
#8787=VERTEX_POINT('',#63996);
#8788=VERTEX_POINT('',#64019);
#8789=VERTEX_POINT('',#64020);
#8790=VERTEX_POINT('',#64043);
#8791=VERTEX_POINT('',#64044);
#8792=VERTEX_POINT('',#64068);
#8793=VERTEX_POINT('',#64069);
#8794=VERTEX_POINT('',#64093);
#8795=VERTEX_POINT('',#64094);
#8796=VERTEX_POINT('',#64117);
#8797=VERTEX_POINT('',#64118);
#8798=VERTEX_POINT('',#64142);
#8799=VERTEX_POINT('',#64143);
#8800=VERTEX_POINT('',#64167);
#8801=VERTEX_POINT('',#64168);
#8802=VERTEX_POINT('',#64191);
#8803=VERTEX_POINT('',#64192);
#8804=VERTEX_POINT('',#64216);
#8805=VERTEX_POINT('',#64217);
#8806=VERTEX_POINT('',#64241);
#8807=VERTEX_POINT('',#64242);
#8808=VERTEX_POINT('',#64265);
#8809=VERTEX_POINT('',#64266);
#8810=VERTEX_POINT('',#64289);
#8811=VERTEX_POINT('',#64290);
#8812=VERTEX_POINT('',#64314);
#8813=VERTEX_POINT('',#64315);
#8814=VERTEX_POINT('',#64339);
#8815=VERTEX_POINT('',#64340);
#8816=VERTEX_POINT('',#64363);
#8817=VERTEX_POINT('',#64364);
#8818=VERTEX_POINT('',#64388);
#8819=VERTEX_POINT('',#64389);
#8820=VERTEX_POINT('',#64413);
#8821=VERTEX_POINT('',#64414);
#8822=VERTEX_POINT('',#64437);
#8823=VERTEX_POINT('',#64438);
#8824=VERTEX_POINT('',#64462);
#8825=VERTEX_POINT('',#64463);
#8826=VERTEX_POINT('',#64487);
#8827=VERTEX_POINT('',#64488);
#8828=VERTEX_POINT('',#64511);
#8829=VERTEX_POINT('',#64512);
#8830=VERTEX_POINT('',#64535);
#8831=VERTEX_POINT('',#64536);
#8832=VERTEX_POINT('',#64560);
#8833=VERTEX_POINT('',#64561);
#8834=VERTEX_POINT('',#64585);
#8835=VERTEX_POINT('',#64586);
#8836=VERTEX_POINT('',#64609);
#8837=VERTEX_POINT('',#64610);
#8838=VERTEX_POINT('',#64634);
#8839=VERTEX_POINT('',#64635);
#8840=VERTEX_POINT('',#64659);
#8841=VERTEX_POINT('',#64660);
#8842=VERTEX_POINT('',#64683);
#8843=VERTEX_POINT('',#64684);
#8844=VERTEX_POINT('',#64708);
#8845=VERTEX_POINT('',#64709);
#8846=VERTEX_POINT('',#64733);
#8847=VERTEX_POINT('',#64734);
#8848=VERTEX_POINT('',#64757);
#8849=VERTEX_POINT('',#64758);
#8850=VERTEX_POINT('',#64781);
#8851=VERTEX_POINT('',#64782);
#8852=VERTEX_POINT('',#64806);
#8853=VERTEX_POINT('',#64807);
#8854=VERTEX_POINT('',#64831);
#8855=VERTEX_POINT('',#64832);
#8856=VERTEX_POINT('',#64855);
#8857=VERTEX_POINT('',#64856);
#8858=VERTEX_POINT('',#64880);
#8859=VERTEX_POINT('',#64881);
#8860=VERTEX_POINT('',#64905);
#8861=VERTEX_POINT('',#64906);
#8862=VERTEX_POINT('',#64929);
#8863=VERTEX_POINT('',#64930);
#8864=VERTEX_POINT('',#64954);
#8865=VERTEX_POINT('',#64955);
#8866=VERTEX_POINT('',#64978);
#8867=VERTEX_POINT('',#64979);
#8868=VERTEX_POINT('',#65003);
#8869=VERTEX_POINT('',#65004);
#8870=VERTEX_POINT('',#65027);
#8871=VERTEX_POINT('',#65028);
#8872=VERTEX_POINT('',#65052);
#8873=VERTEX_POINT('',#65053);
#8874=VERTEX_POINT('',#65077);
#8875=VERTEX_POINT('',#65078);
#8876=VERTEX_POINT('',#65101);
#8877=VERTEX_POINT('',#65102);
#8878=VERTEX_POINT('',#65126);
#8879=VERTEX_POINT('',#65127);
#8880=VERTEX_POINT('',#65151);
#8881=VERTEX_POINT('',#65152);
#8882=VERTEX_POINT('',#65175);
#8883=VERTEX_POINT('',#65176);
#8884=VERTEX_POINT('',#65200);
#8885=VERTEX_POINT('',#65201);
#8886=VERTEX_POINT('',#65224);
#8887=VERTEX_POINT('',#65225);
#8888=VERTEX_POINT('',#65249);
#8889=VERTEX_POINT('',#65250);
#8890=VERTEX_POINT('',#66812);
#8891=VERTEX_POINT('',#66941);
#8892=VERTEX_POINT('',#67058);
#8893=VERTEX_POINT('',#68609);
#8894=VERTEX_POINT('',#68844);
#8895=VERTEX_POINT('',#68845);
#8896=VERTEX_POINT('',#68847);
#8897=VERTEX_POINT('',#68849);
#8898=VERTEX_POINT('',#68851);
#8899=VERTEX_POINT('',#68853);
#8900=VERTEX_POINT('',#68857);
#8901=VERTEX_POINT('',#68858);
#8902=VERTEX_POINT('',#68860);
#8903=VERTEX_POINT('',#68862);
#8904=VERTEX_POINT('',#68864);
#8905=VERTEX_POINT('',#68866);
#8906=VERTEX_POINT('',#68869);
#8907=VERTEX_POINT('',#68884);
#8908=VERTEX_POINT('',#68889);
#11362=EDGE_CURVE('',#8646,#8647,#5551,.T.);
#11363=EDGE_CURVE('',#8646,#8648,#1122,.T.);
#11364=EDGE_CURVE('',#8648,#8649,#7552,.F.);
#11365=EDGE_CURVE('',#8649,#8647,#1123,.T.);
#11366=EDGE_CURVE('',#8650,#8651,#5552,.T.);
#11367=EDGE_CURVE('',#8650,#8646,#1124,.T.);
#11368=EDGE_CURVE('',#8647,#8651,#1125,.T.);
#11369=EDGE_CURVE('',#8652,#8653,#5553,.T.);
#11370=EDGE_CURVE('',#8652,#8650,#1126,.T.);
#11371=EDGE_CURVE('',#8651,#8653,#1127,.T.);
#11372=EDGE_CURVE('',#8654,#8655,#5554,.T.);
#11373=EDGE_CURVE('',#8654,#8652,#1128,.T.);
#11374=EDGE_CURVE('',#8653,#8655,#1129,.T.);
#11375=EDGE_CURVE('',#8656,#8657,#5555,.T.);
#11376=EDGE_CURVE('',#8656,#8654,#1130,.T.);
#11377=EDGE_CURVE('',#8655,#8657,#1131,.T.);
#11378=EDGE_CURVE('',#8658,#8659,#5556,.T.);
#11379=EDGE_CURVE('',#8658,#8656,#1132,.T.);
#11380=EDGE_CURVE('',#8657,#8659,#1133,.T.);
#11381=EDGE_CURVE('',#8660,#8661,#5557,.T.);
#11382=EDGE_CURVE('',#8660,#8658,#1134,.T.);
#11383=EDGE_CURVE('',#8659,#8661,#1135,.T.);
#11384=EDGE_CURVE('',#8662,#8663,#5558,.T.);
#11385=EDGE_CURVE('',#8662,#8660,#1136,.T.);
#11386=EDGE_CURVE('',#8661,#8663,#1137,.T.);
#11387=EDGE_CURVE('',#8664,#8665,#5559,.T.);
#11388=EDGE_CURVE('',#8664,#8662,#1138,.T.);
#11389=EDGE_CURVE('',#8663,#8665,#1139,.T.);
#11390=EDGE_CURVE('',#8666,#8667,#5560,.T.);
#11391=EDGE_CURVE('',#8666,#8664,#1140,.T.);
#11392=EDGE_CURVE('',#8665,#8667,#1141,.T.);
#11393=EDGE_CURVE('',#8668,#8669,#5561,.T.);
#11394=EDGE_CURVE('',#8668,#8666,#1142,.T.);
#11395=EDGE_CURVE('',#8667,#8669,#1143,.T.);
#11396=EDGE_CURVE('',#8670,#8671,#5562,.T.);
#11397=EDGE_CURVE('',#8670,#8668,#1144,.T.);
#11398=EDGE_CURVE('',#8669,#8671,#1145,.T.);
#11399=EDGE_CURVE('',#8672,#8673,#5563,.T.);
#11400=EDGE_CURVE('',#8672,#8670,#1146,.T.);
#11401=EDGE_CURVE('',#8671,#8673,#1147,.T.);
#11402=EDGE_CURVE('',#8674,#8675,#5564,.T.);
#11403=EDGE_CURVE('',#8674,#8672,#1148,.T.);
#11404=EDGE_CURVE('',#8673,#8675,#1149,.T.);
#11405=EDGE_CURVE('',#8676,#8677,#5565,.T.);
#11406=EDGE_CURVE('',#8676,#8674,#1150,.T.);
#11407=EDGE_CURVE('',#8675,#8677,#1151,.T.);
#11408=EDGE_CURVE('',#8678,#8679,#5566,.T.);
#11409=EDGE_CURVE('',#8678,#8676,#1152,.T.);
#11410=EDGE_CURVE('',#8677,#8679,#1153,.T.);
#11411=EDGE_CURVE('',#8680,#8681,#5567,.T.);
#11412=EDGE_CURVE('',#8680,#8678,#1154,.T.);
#11413=EDGE_CURVE('',#8679,#8681,#1155,.T.);
#11414=EDGE_CURVE('',#8682,#8683,#5568,.T.);
#11415=EDGE_CURVE('',#8682,#8680,#1156,.T.);
#11416=EDGE_CURVE('',#8681,#8683,#1157,.T.);
#11417=EDGE_CURVE('',#8684,#8685,#5569,.T.);
#11418=EDGE_CURVE('',#8684,#8682,#1158,.T.);
#11419=EDGE_CURVE('',#8683,#8685,#1159,.T.);
#11420=EDGE_CURVE('',#8686,#8687,#5570,.T.);
#11421=EDGE_CURVE('',#8686,#8684,#1160,.T.);
#11422=EDGE_CURVE('',#8685,#8687,#1161,.T.);
#11423=EDGE_CURVE('',#8688,#8689,#5571,.T.);
#11424=EDGE_CURVE('',#8688,#8686,#1162,.T.);
#11425=EDGE_CURVE('',#8687,#8689,#1163,.T.);
#11426=EDGE_CURVE('',#8690,#8691,#5572,.T.);
#11427=EDGE_CURVE('',#8690,#8688,#1164,.T.);
#11428=EDGE_CURVE('',#8689,#8691,#1165,.T.);
#11429=EDGE_CURVE('',#8692,#8693,#5573,.T.);
#11430=EDGE_CURVE('',#8692,#8690,#1166,.T.);
#11431=EDGE_CURVE('',#8691,#8693,#1167,.T.);
#11432=EDGE_CURVE('',#8694,#8695,#5574,.T.);
#11433=EDGE_CURVE('',#8694,#8692,#1168,.T.);
#11434=EDGE_CURVE('',#8693,#8695,#1169,.T.);
#11435=EDGE_CURVE('',#8696,#8697,#5575,.T.);
#11436=EDGE_CURVE('',#8696,#8694,#1170,.T.);
#11437=EDGE_CURVE('',#8695,#8697,#1171,.T.);
#11438=EDGE_CURVE('',#8698,#8699,#5576,.T.);
#11439=EDGE_CURVE('',#8698,#8696,#1172,.T.);
#11440=EDGE_CURVE('',#8697,#8699,#1173,.T.);
#11441=EDGE_CURVE('',#8700,#8701,#5577,.T.);
#11442=EDGE_CURVE('',#8700,#8698,#1174,.T.);
#11443=EDGE_CURVE('',#8699,#8701,#1175,.T.);
#11444=EDGE_CURVE('',#8702,#8703,#5578,.T.);
#11445=EDGE_CURVE('',#8702,#8700,#1176,.T.);
#11446=EDGE_CURVE('',#8701,#8703,#1177,.T.);
#11447=EDGE_CURVE('',#8704,#8705,#5579,.T.);
#11448=EDGE_CURVE('',#8704,#8702,#1178,.T.);
#11449=EDGE_CURVE('',#8703,#8705,#1179,.T.);
#11450=EDGE_CURVE('',#8706,#8707,#5580,.T.);
#11451=EDGE_CURVE('',#8706,#8704,#1180,.T.);
#11452=EDGE_CURVE('',#8705,#8707,#1181,.T.);
#11453=EDGE_CURVE('',#8708,#8709,#5581,.T.);
#11454=EDGE_CURVE('',#8708,#8706,#1182,.T.);
#11455=EDGE_CURVE('',#8707,#8709,#1183,.T.);
#11456=EDGE_CURVE('',#8710,#8711,#5582,.T.);
#11457=EDGE_CURVE('',#8710,#8708,#1184,.T.);
#11458=EDGE_CURVE('',#8709,#8711,#1185,.T.);
#11459=EDGE_CURVE('',#8712,#8713,#5583,.T.);
#11460=EDGE_CURVE('',#8712,#8710,#1186,.T.);
#11461=EDGE_CURVE('',#8711,#8713,#1187,.T.);
#11462=EDGE_CURVE('',#8714,#8715,#5584,.T.);
#11463=EDGE_CURVE('',#8714,#8712,#1188,.T.);
#11464=EDGE_CURVE('',#8713,#8715,#1189,.T.);
#11465=EDGE_CURVE('',#8716,#8717,#5585,.T.);
#11466=EDGE_CURVE('',#8716,#8714,#1190,.T.);
#11467=EDGE_CURVE('',#8715,#8717,#1191,.T.);
#11468=EDGE_CURVE('',#8718,#8719,#5586,.T.);
#11469=EDGE_CURVE('',#8718,#8716,#1192,.T.);
#11470=EDGE_CURVE('',#8717,#8719,#1193,.T.);
#11471=EDGE_CURVE('',#8720,#8721,#5587,.T.);
#11472=EDGE_CURVE('',#8720,#8718,#1194,.T.);
#11473=EDGE_CURVE('',#8719,#8721,#1195,.T.);
#11474=EDGE_CURVE('',#8722,#8723,#5588,.T.);
#11475=EDGE_CURVE('',#8722,#8720,#1196,.T.);
#11476=EDGE_CURVE('',#8721,#8723,#1197,.T.);
#11477=EDGE_CURVE('',#8724,#8725,#5589,.T.);
#11478=EDGE_CURVE('',#8724,#8722,#1198,.T.);
#11479=EDGE_CURVE('',#8723,#8725,#1199,.T.);
#11480=EDGE_CURVE('',#8726,#8727,#5590,.T.);
#11481=EDGE_CURVE('',#8726,#8724,#1200,.T.);
#11482=EDGE_CURVE('',#8725,#8727,#1201,.T.);
#11483=EDGE_CURVE('',#8728,#8729,#5591,.T.);
#11484=EDGE_CURVE('',#8728,#8726,#1202,.T.);
#11485=EDGE_CURVE('',#8727,#8729,#1203,.T.);
#11486=EDGE_CURVE('',#8730,#8731,#5592,.T.);
#11487=EDGE_CURVE('',#8730,#8728,#1204,.T.);
#11488=EDGE_CURVE('',#8729,#8731,#1205,.T.);
#11489=EDGE_CURVE('',#8732,#8733,#5593,.T.);
#11490=EDGE_CURVE('',#8732,#8730,#1206,.T.);
#11491=EDGE_CURVE('',#8731,#8733,#1207,.T.);
#11492=EDGE_CURVE('',#8734,#8735,#5594,.T.);
#11493=EDGE_CURVE('',#8734,#8732,#1208,.T.);
#11494=EDGE_CURVE('',#8733,#8735,#1209,.T.);
#11495=EDGE_CURVE('',#8736,#8737,#5595,.T.);
#11496=EDGE_CURVE('',#8736,#8734,#1210,.T.);
#11497=EDGE_CURVE('',#8735,#8737,#1211,.T.);
#11498=EDGE_CURVE('',#8738,#8739,#5596,.T.);
#11499=EDGE_CURVE('',#8738,#8736,#1212,.T.);
#11500=EDGE_CURVE('',#8737,#8739,#1213,.T.);
#11501=EDGE_CURVE('',#8740,#8741,#5597,.T.);
#11502=EDGE_CURVE('',#8740,#8738,#1214,.T.);
#11503=EDGE_CURVE('',#8739,#8741,#1215,.T.);
#11504=EDGE_CURVE('',#8742,#8743,#5598,.T.);
#11505=EDGE_CURVE('',#8742,#8740,#1216,.T.);
#11506=EDGE_CURVE('',#8741,#8743,#1217,.T.);
#11507=EDGE_CURVE('',#8744,#8745,#5599,.T.);
#11508=EDGE_CURVE('',#8744,#8742,#1218,.T.);
#11509=EDGE_CURVE('',#8743,#8745,#1219,.T.);
#11510=EDGE_CURVE('',#8746,#8747,#5600,.T.);
#11511=EDGE_CURVE('',#8746,#8744,#1220,.T.);
#11512=EDGE_CURVE('',#8745,#8747,#1221,.T.);
#11513=EDGE_CURVE('',#8748,#8749,#5601,.T.);
#11514=EDGE_CURVE('',#8748,#8746,#1222,.T.);
#11515=EDGE_CURVE('',#8747,#8749,#1223,.T.);
#11516=EDGE_CURVE('',#8750,#8751,#5602,.T.);
#11517=EDGE_CURVE('',#8750,#8748,#1224,.T.);
#11518=EDGE_CURVE('',#8749,#8751,#1225,.T.);
#11519=EDGE_CURVE('',#8752,#8753,#5603,.T.);
#11520=EDGE_CURVE('',#8752,#8750,#1226,.T.);
#11521=EDGE_CURVE('',#8751,#8753,#1227,.T.);
#11522=EDGE_CURVE('',#8754,#8755,#5604,.T.);
#11523=EDGE_CURVE('',#8754,#8752,#1228,.T.);
#11524=EDGE_CURVE('',#8753,#8755,#1229,.T.);
#11525=EDGE_CURVE('',#8756,#8757,#5605,.T.);
#11526=EDGE_CURVE('',#8756,#8754,#1230,.T.);
#11527=EDGE_CURVE('',#8755,#8757,#1231,.T.);
#11528=EDGE_CURVE('',#8758,#8759,#5606,.T.);
#11529=EDGE_CURVE('',#8758,#8756,#1232,.T.);
#11530=EDGE_CURVE('',#8757,#8759,#1233,.T.);
#11531=EDGE_CURVE('',#8760,#8761,#5607,.T.);
#11532=EDGE_CURVE('',#8760,#8758,#1234,.T.);
#11533=EDGE_CURVE('',#8759,#8761,#1235,.T.);
#11534=EDGE_CURVE('',#8762,#8763,#5608,.T.);
#11535=EDGE_CURVE('',#8762,#8760,#1236,.T.);
#11536=EDGE_CURVE('',#8761,#8763,#1237,.T.);
#11537=EDGE_CURVE('',#8764,#8765,#5609,.T.);
#11538=EDGE_CURVE('',#8764,#8762,#1238,.T.);
#11539=EDGE_CURVE('',#8763,#8765,#1239,.T.);
#11540=EDGE_CURVE('',#8766,#8767,#5610,.T.);
#11541=EDGE_CURVE('',#8766,#8764,#1240,.T.);
#11542=EDGE_CURVE('',#8765,#8767,#1241,.T.);
#11543=EDGE_CURVE('',#8768,#8769,#5611,.T.);
#11544=EDGE_CURVE('',#8768,#8770,#1242,.T.);
#11545=EDGE_CURVE('',#8771,#8770,#7553,.T.);
#11546=EDGE_CURVE('',#8769,#8771,#1243,.T.);
#11547=EDGE_CURVE('',#8772,#8773,#5612,.T.);
#11548=EDGE_CURVE('',#8772,#8768,#1244,.T.);
#11549=EDGE_CURVE('',#8773,#8769,#1245,.T.);
#11550=EDGE_CURVE('',#8774,#8775,#5613,.T.);
#11551=EDGE_CURVE('',#8774,#8772,#1246,.T.);
#11552=EDGE_CURVE('',#8775,#8773,#1247,.T.);
#11553=EDGE_CURVE('',#8776,#8777,#5614,.T.);
#11554=EDGE_CURVE('',#8776,#8774,#1248,.T.);
#11555=EDGE_CURVE('',#8777,#8775,#1249,.T.);
#11556=EDGE_CURVE('',#8778,#8779,#5615,.T.);
#11557=EDGE_CURVE('',#8778,#8776,#1250,.T.);
#11558=EDGE_CURVE('',#8779,#8777,#1251,.T.);
#11559=EDGE_CURVE('',#8780,#8781,#5616,.T.);
#11560=EDGE_CURVE('',#8780,#8778,#1252,.T.);
#11561=EDGE_CURVE('',#8781,#8779,#1253,.T.);
#11562=EDGE_CURVE('',#8782,#8783,#5617,.T.);
#11563=EDGE_CURVE('',#8782,#8780,#1254,.T.);
#11564=EDGE_CURVE('',#8783,#8781,#1255,.T.);
#11565=EDGE_CURVE('',#8784,#8785,#5618,.T.);
#11566=EDGE_CURVE('',#8784,#8782,#1256,.T.);
#11567=EDGE_CURVE('',#8785,#8783,#1257,.T.);
#11568=EDGE_CURVE('',#8786,#8787,#5619,.T.);
#11569=EDGE_CURVE('',#8786,#8784,#1258,.T.);
#11570=EDGE_CURVE('',#8787,#8785,#1259,.T.);
#11571=EDGE_CURVE('',#8788,#8789,#5620,.T.);
#11572=EDGE_CURVE('',#8788,#8786,#1260,.T.);
#11573=EDGE_CURVE('',#8789,#8787,#1261,.T.);
#11574=EDGE_CURVE('',#8790,#8791,#5621,.T.);
#11575=EDGE_CURVE('',#8790,#8788,#1262,.T.);
#11576=EDGE_CURVE('',#8791,#8789,#1263,.T.);
#11577=EDGE_CURVE('',#8792,#8793,#5622,.T.);
#11578=EDGE_CURVE('',#8792,#8790,#1264,.T.);
#11579=EDGE_CURVE('',#8793,#8791,#1265,.T.);
#11580=EDGE_CURVE('',#8794,#8795,#5623,.T.);
#11581=EDGE_CURVE('',#8794,#8792,#1266,.T.);
#11582=EDGE_CURVE('',#8795,#8793,#1267,.T.);
#11583=EDGE_CURVE('',#8796,#8797,#5624,.T.);
#11584=EDGE_CURVE('',#8796,#8794,#1268,.T.);
#11585=EDGE_CURVE('',#8797,#8795,#1269,.T.);
#11586=EDGE_CURVE('',#8798,#8799,#5625,.T.);
#11587=EDGE_CURVE('',#8798,#8796,#1270,.T.);
#11588=EDGE_CURVE('',#8799,#8797,#1271,.T.);
#11589=EDGE_CURVE('',#8800,#8801,#5626,.T.);
#11590=EDGE_CURVE('',#8800,#8798,#1272,.T.);
#11591=EDGE_CURVE('',#8801,#8799,#1273,.T.);
#11592=EDGE_CURVE('',#8802,#8803,#5627,.T.);
#11593=EDGE_CURVE('',#8802,#8800,#1274,.T.);
#11594=EDGE_CURVE('',#8803,#8801,#1275,.T.);
#11595=EDGE_CURVE('',#8804,#8805,#5628,.T.);
#11596=EDGE_CURVE('',#8804,#8802,#1276,.T.);
#11597=EDGE_CURVE('',#8805,#8803,#1277,.T.);
#11598=EDGE_CURVE('',#8806,#8807,#5629,.T.);
#11599=EDGE_CURVE('',#8806,#8804,#1278,.T.);
#11600=EDGE_CURVE('',#8807,#8805,#1279,.T.);
#11601=EDGE_CURVE('',#8808,#8809,#5630,.T.);
#11602=EDGE_CURVE('',#8808,#8806,#1280,.T.);
#11603=EDGE_CURVE('',#8809,#8807,#1281,.T.);
#11604=EDGE_CURVE('',#8810,#8811,#5631,.T.);
#11605=EDGE_CURVE('',#8810,#8808,#1282,.T.);
#11606=EDGE_CURVE('',#8811,#8809,#1283,.T.);
#11607=EDGE_CURVE('',#8812,#8813,#5632,.T.);
#11608=EDGE_CURVE('',#8812,#8810,#1284,.T.);
#11609=EDGE_CURVE('',#8813,#8811,#1285,.T.);
#11610=EDGE_CURVE('',#8814,#8815,#5633,.T.);
#11611=EDGE_CURVE('',#8814,#8812,#1286,.T.);
#11612=EDGE_CURVE('',#8815,#8813,#1287,.T.);
#11613=EDGE_CURVE('',#8816,#8817,#5634,.T.);
#11614=EDGE_CURVE('',#8816,#8814,#1288,.T.);
#11615=EDGE_CURVE('',#8817,#8815,#1289,.T.);
#11616=EDGE_CURVE('',#8818,#8819,#5635,.T.);
#11617=EDGE_CURVE('',#8818,#8816,#1290,.T.);
#11618=EDGE_CURVE('',#8819,#8817,#1291,.T.);
#11619=EDGE_CURVE('',#8820,#8821,#5636,.T.);
#11620=EDGE_CURVE('',#8820,#8818,#1292,.T.);
#11621=EDGE_CURVE('',#8821,#8819,#1293,.T.);
#11622=EDGE_CURVE('',#8822,#8823,#5637,.T.);
#11623=EDGE_CURVE('',#8822,#8820,#1294,.T.);
#11624=EDGE_CURVE('',#8823,#8821,#1295,.T.);
#11625=EDGE_CURVE('',#8824,#8825,#5638,.T.);
#11626=EDGE_CURVE('',#8824,#8822,#1296,.T.);
#11627=EDGE_CURVE('',#8825,#8823,#1297,.T.);
#11628=EDGE_CURVE('',#8826,#8827,#5639,.T.);
#11629=EDGE_CURVE('',#8826,#8824,#1298,.T.);
#11630=EDGE_CURVE('',#8827,#8825,#1299,.T.);
#11631=EDGE_CURVE('',#8828,#8829,#5640,.T.);
#11632=EDGE_CURVE('',#8828,#8826,#1300,.T.);
#11633=EDGE_CURVE('',#8829,#8827,#1301,.T.);
#11634=EDGE_CURVE('',#8830,#8831,#5641,.T.);
#11635=EDGE_CURVE('',#8830,#8828,#1302,.T.);
#11636=EDGE_CURVE('',#8831,#8829,#1303,.T.);
#11637=EDGE_CURVE('',#8832,#8833,#5642,.T.);
#11638=EDGE_CURVE('',#8832,#8830,#1304,.T.);
#11639=EDGE_CURVE('',#8833,#8831,#1305,.T.);
#11640=EDGE_CURVE('',#8834,#8835,#5643,.T.);
#11641=EDGE_CURVE('',#8834,#8832,#1306,.T.);
#11642=EDGE_CURVE('',#8835,#8833,#1307,.T.);
#11643=EDGE_CURVE('',#8836,#8837,#5644,.T.);
#11644=EDGE_CURVE('',#8836,#8834,#1308,.T.);
#11645=EDGE_CURVE('',#8837,#8835,#1309,.T.);
#11646=EDGE_CURVE('',#8838,#8839,#5645,.T.);
#11647=EDGE_CURVE('',#8838,#8836,#1310,.T.);
#11648=EDGE_CURVE('',#8839,#8837,#1311,.T.);
#11649=EDGE_CURVE('',#8840,#8841,#5646,.T.);
#11650=EDGE_CURVE('',#8840,#8838,#1312,.T.);
#11651=EDGE_CURVE('',#8841,#8839,#1313,.T.);
#11652=EDGE_CURVE('',#8842,#8843,#5647,.T.);
#11653=EDGE_CURVE('',#8842,#8840,#1314,.T.);
#11654=EDGE_CURVE('',#8843,#8841,#1315,.T.);
#11655=EDGE_CURVE('',#8844,#8845,#5648,.T.);
#11656=EDGE_CURVE('',#8844,#8842,#1316,.T.);
#11657=EDGE_CURVE('',#8845,#8843,#1317,.T.);
#11658=EDGE_CURVE('',#8846,#8847,#5649,.T.);
#11659=EDGE_CURVE('',#8846,#8844,#1318,.T.);
#11660=EDGE_CURVE('',#8847,#8845,#1319,.T.);
#11661=EDGE_CURVE('',#8848,#8849,#5650,.T.);
#11662=EDGE_CURVE('',#8848,#8846,#1320,.T.);
#11663=EDGE_CURVE('',#8849,#8847,#1321,.T.);
#11664=EDGE_CURVE('',#8850,#8851,#5651,.T.);
#11665=EDGE_CURVE('',#8850,#8848,#1322,.T.);
#11666=EDGE_CURVE('',#8851,#8849,#1323,.T.);
#11667=EDGE_CURVE('',#8852,#8853,#5652,.T.);
#11668=EDGE_CURVE('',#8852,#8850,#1324,.T.);
#11669=EDGE_CURVE('',#8853,#8851,#1325,.T.);
#11670=EDGE_CURVE('',#8854,#8855,#5653,.T.);
#11671=EDGE_CURVE('',#8854,#8852,#1326,.T.);
#11672=EDGE_CURVE('',#8855,#8853,#1327,.T.);
#11673=EDGE_CURVE('',#8856,#8857,#5654,.T.);
#11674=EDGE_CURVE('',#8856,#8854,#1328,.T.);
#11675=EDGE_CURVE('',#8857,#8855,#1329,.T.);
#11676=EDGE_CURVE('',#8858,#8859,#5655,.T.);
#11677=EDGE_CURVE('',#8858,#8856,#1330,.T.);
#11678=EDGE_CURVE('',#8859,#8857,#1331,.T.);
#11679=EDGE_CURVE('',#8860,#8861,#5656,.T.);
#11680=EDGE_CURVE('',#8860,#8858,#1332,.T.);
#11681=EDGE_CURVE('',#8861,#8859,#1333,.T.);
#11682=EDGE_CURVE('',#8862,#8863,#5657,.T.);
#11683=EDGE_CURVE('',#8862,#8860,#1334,.T.);
#11684=EDGE_CURVE('',#8863,#8861,#1335,.T.);
#11685=EDGE_CURVE('',#8864,#8865,#5658,.T.);
#11686=EDGE_CURVE('',#8864,#8862,#1336,.T.);
#11687=EDGE_CURVE('',#8865,#8863,#1337,.T.);
#11688=EDGE_CURVE('',#8866,#8867,#5659,.T.);
#11689=EDGE_CURVE('',#8866,#8864,#1338,.T.);
#11690=EDGE_CURVE('',#8867,#8865,#1339,.T.);
#11691=EDGE_CURVE('',#8868,#8869,#5660,.T.);
#11692=EDGE_CURVE('',#8868,#8866,#1340,.T.);
#11693=EDGE_CURVE('',#8869,#8867,#1341,.T.);
#11694=EDGE_CURVE('',#8870,#8871,#5661,.T.);
#11695=EDGE_CURVE('',#8870,#8868,#1342,.T.);
#11696=EDGE_CURVE('',#8871,#8869,#1343,.T.);
#11697=EDGE_CURVE('',#8872,#8873,#5662,.T.);
#11698=EDGE_CURVE('',#8872,#8870,#1344,.T.);
#11699=EDGE_CURVE('',#8873,#8871,#1345,.T.);
#11700=EDGE_CURVE('',#8874,#8875,#5663,.T.);
#11701=EDGE_CURVE('',#8874,#8872,#1346,.T.);
#11702=EDGE_CURVE('',#8875,#8873,#1347,.T.);
#11703=EDGE_CURVE('',#8876,#8877,#5664,.T.);
#11704=EDGE_CURVE('',#8876,#8874,#1348,.T.);
#11705=EDGE_CURVE('',#8877,#8875,#1349,.T.);
#11706=EDGE_CURVE('',#8878,#8879,#5665,.T.);
#11707=EDGE_CURVE('',#8878,#8876,#1350,.T.);
#11708=EDGE_CURVE('',#8879,#8877,#1351,.T.);
#11709=EDGE_CURVE('',#8880,#8881,#5666,.T.);
#11710=EDGE_CURVE('',#8880,#8878,#1352,.T.);
#11711=EDGE_CURVE('',#8881,#8879,#1353,.T.);
#11712=EDGE_CURVE('',#8882,#8883,#5667,.T.);
#11713=EDGE_CURVE('',#8882,#8880,#1354,.T.);
#11714=EDGE_CURVE('',#8883,#8881,#1355,.T.);
#11715=EDGE_CURVE('',#8884,#8885,#5668,.T.);
#11716=EDGE_CURVE('',#8884,#8882,#1356,.T.);
#11717=EDGE_CURVE('',#8885,#8883,#1357,.T.);
#11718=EDGE_CURVE('',#8886,#8887,#5669,.T.);
#11719=EDGE_CURVE('',#8886,#8884,#1358,.T.);
#11720=EDGE_CURVE('',#8887,#8885,#1359,.T.);
#11721=EDGE_CURVE('',#8888,#8889,#5670,.T.);
#11722=EDGE_CURVE('',#8888,#8886,#1360,.T.);
#11723=EDGE_CURVE('',#8889,#8887,#1361,.T.);
#11724=EDGE_CURVE('',#8890,#8771,#1362,.T.);
#11725=EDGE_CURVE('',#8767,#8890,#1363,.T.);
#11726=EDGE_CURVE('',#8891,#8649,#1364,.T.);
#11727=EDGE_CURVE('',#8891,#8889,#1365,.T.);
#11728=EDGE_CURVE('',#8892,#8891,#7554,.T.);
#11729=EDGE_CURVE('',#8892,#8888,#1366,.T.);
#11730=EDGE_CURVE('',#8770,#8893,#1367,.T.);
#11731=EDGE_CURVE('',#8648,#8892,#1368,.T.);
#11732=EDGE_CURVE('',#8893,#8766,#1369,.T.);
#11733=EDGE_CURVE('',#8893,#8890,#7555,.F.);
#11734=EDGE_CURVE('',#8894,#8895,#5671,.T.);
#11735=EDGE_CURVE('',#8895,#8896,#5672,.T.);
#11736=EDGE_CURVE('',#8896,#8897,#5673,.T.);
#11737=EDGE_CURVE('',#8897,#8898,#5674,.T.);
#11738=EDGE_CURVE('',#8898,#8899,#5675,.T.);
#11739=EDGE_CURVE('',#8899,#8894,#5676,.T.);
#11740=EDGE_CURVE('',#8900,#8901,#5677,.T.);
#11741=EDGE_CURVE('',#8902,#8900,#5678,.T.);
#11742=EDGE_CURVE('',#8903,#8902,#5679,.T.);
#11743=EDGE_CURVE('',#8904,#8903,#5680,.T.);
#11744=EDGE_CURVE('',#8905,#8904,#5681,.T.);
#11745=EDGE_CURVE('',#8901,#8905,#5682,.T.);
#11746=EDGE_CURVE('',#8906,#8906,#7556,.T.);
#11747=EDGE_CURVE('',#8900,#8894,#5683,.T.);
#11748=EDGE_CURVE('',#8902,#8899,#5684,.T.);
#11749=EDGE_CURVE('',#8903,#8898,#5685,.T.);
#11750=EDGE_CURVE('',#8904,#8897,#5686,.T.);
#11751=EDGE_CURVE('',#8905,#8896,#5687,.T.);
#11752=EDGE_CURVE('',#8901,#8895,#5688,.T.);
#11753=EDGE_CURVE('',#8906,#8907,#5689,.T.);
#11754=EDGE_CURVE('',#8907,#8907,#7557,.T.);
#11755=EDGE_CURVE('',#8907,#8908,#7558,.T.);
#16210=ORIENTED_EDGE('',*,*,#11362,.F.);
#16211=ORIENTED_EDGE('',*,*,#11363,.T.);
#16212=ORIENTED_EDGE('',*,*,#11364,.T.);
#16213=ORIENTED_EDGE('',*,*,#11365,.T.);
#16214=ORIENTED_EDGE('',*,*,#11366,.F.);
#16215=ORIENTED_EDGE('',*,*,#11367,.T.);
#16216=ORIENTED_EDGE('',*,*,#11362,.T.);
#16217=ORIENTED_EDGE('',*,*,#11368,.T.);
#16218=ORIENTED_EDGE('',*,*,#11369,.F.);
#16219=ORIENTED_EDGE('',*,*,#11370,.T.);
#16220=ORIENTED_EDGE('',*,*,#11366,.T.);
#16221=ORIENTED_EDGE('',*,*,#11371,.T.);
#16222=ORIENTED_EDGE('',*,*,#11372,.F.);
#16223=ORIENTED_EDGE('',*,*,#11373,.T.);
#16224=ORIENTED_EDGE('',*,*,#11369,.T.);
#16225=ORIENTED_EDGE('',*,*,#11374,.T.);
#16226=ORIENTED_EDGE('',*,*,#11375,.F.);
#16227=ORIENTED_EDGE('',*,*,#11376,.T.);
#16228=ORIENTED_EDGE('',*,*,#11372,.T.);
#16229=ORIENTED_EDGE('',*,*,#11377,.T.);
#16230=ORIENTED_EDGE('',*,*,#11378,.F.);
#16231=ORIENTED_EDGE('',*,*,#11379,.T.);
#16232=ORIENTED_EDGE('',*,*,#11375,.T.);
#16233=ORIENTED_EDGE('',*,*,#11380,.T.);
#16234=ORIENTED_EDGE('',*,*,#11381,.F.);
#16235=ORIENTED_EDGE('',*,*,#11382,.T.);
#16236=ORIENTED_EDGE('',*,*,#11378,.T.);
#16237=ORIENTED_EDGE('',*,*,#11383,.T.);
#16238=ORIENTED_EDGE('',*,*,#11384,.F.);
#16239=ORIENTED_EDGE('',*,*,#11385,.T.);
#16240=ORIENTED_EDGE('',*,*,#11381,.T.);
#16241=ORIENTED_EDGE('',*,*,#11386,.T.);
#16242=ORIENTED_EDGE('',*,*,#11387,.F.);
#16243=ORIENTED_EDGE('',*,*,#11388,.T.);
#16244=ORIENTED_EDGE('',*,*,#11384,.T.);
#16245=ORIENTED_EDGE('',*,*,#11389,.T.);
#16246=ORIENTED_EDGE('',*,*,#11390,.F.);
#16247=ORIENTED_EDGE('',*,*,#11391,.T.);
#16248=ORIENTED_EDGE('',*,*,#11387,.T.);
#16249=ORIENTED_EDGE('',*,*,#11392,.T.);
#16250=ORIENTED_EDGE('',*,*,#11393,.F.);
#16251=ORIENTED_EDGE('',*,*,#11394,.T.);
#16252=ORIENTED_EDGE('',*,*,#11390,.T.);
#16253=ORIENTED_EDGE('',*,*,#11395,.T.);
#16254=ORIENTED_EDGE('',*,*,#11396,.F.);
#16255=ORIENTED_EDGE('',*,*,#11397,.T.);
#16256=ORIENTED_EDGE('',*,*,#11393,.T.);
#16257=ORIENTED_EDGE('',*,*,#11398,.T.);
#16258=ORIENTED_EDGE('',*,*,#11399,.F.);
#16259=ORIENTED_EDGE('',*,*,#11400,.T.);
#16260=ORIENTED_EDGE('',*,*,#11396,.T.);
#16261=ORIENTED_EDGE('',*,*,#11401,.T.);
#16262=ORIENTED_EDGE('',*,*,#11402,.F.);
#16263=ORIENTED_EDGE('',*,*,#11403,.T.);
#16264=ORIENTED_EDGE('',*,*,#11399,.T.);
#16265=ORIENTED_EDGE('',*,*,#11404,.T.);
#16266=ORIENTED_EDGE('',*,*,#11405,.F.);
#16267=ORIENTED_EDGE('',*,*,#11406,.T.);
#16268=ORIENTED_EDGE('',*,*,#11402,.T.);
#16269=ORIENTED_EDGE('',*,*,#11407,.T.);
#16270=ORIENTED_EDGE('',*,*,#11408,.F.);
#16271=ORIENTED_EDGE('',*,*,#11409,.T.);
#16272=ORIENTED_EDGE('',*,*,#11405,.T.);
#16273=ORIENTED_EDGE('',*,*,#11410,.T.);
#16274=ORIENTED_EDGE('',*,*,#11411,.F.);
#16275=ORIENTED_EDGE('',*,*,#11412,.T.);
#16276=ORIENTED_EDGE('',*,*,#11408,.T.);
#16277=ORIENTED_EDGE('',*,*,#11413,.T.);
#16278=ORIENTED_EDGE('',*,*,#11414,.F.);
#16279=ORIENTED_EDGE('',*,*,#11415,.T.);
#16280=ORIENTED_EDGE('',*,*,#11411,.T.);
#16281=ORIENTED_EDGE('',*,*,#11416,.T.);
#16282=ORIENTED_EDGE('',*,*,#11417,.F.);
#16283=ORIENTED_EDGE('',*,*,#11418,.T.);
#16284=ORIENTED_EDGE('',*,*,#11414,.T.);
#16285=ORIENTED_EDGE('',*,*,#11419,.T.);
#16286=ORIENTED_EDGE('',*,*,#11420,.F.);
#16287=ORIENTED_EDGE('',*,*,#11421,.T.);
#16288=ORIENTED_EDGE('',*,*,#11417,.T.);
#16289=ORIENTED_EDGE('',*,*,#11422,.T.);
#16290=ORIENTED_EDGE('',*,*,#11423,.F.);
#16291=ORIENTED_EDGE('',*,*,#11424,.T.);
#16292=ORIENTED_EDGE('',*,*,#11420,.T.);
#16293=ORIENTED_EDGE('',*,*,#11425,.T.);
#16294=ORIENTED_EDGE('',*,*,#11426,.F.);
#16295=ORIENTED_EDGE('',*,*,#11427,.T.);
#16296=ORIENTED_EDGE('',*,*,#11423,.T.);
#16297=ORIENTED_EDGE('',*,*,#11428,.T.);
#16298=ORIENTED_EDGE('',*,*,#11429,.F.);
#16299=ORIENTED_EDGE('',*,*,#11430,.T.);
#16300=ORIENTED_EDGE('',*,*,#11426,.T.);
#16301=ORIENTED_EDGE('',*,*,#11431,.T.);
#16302=ORIENTED_EDGE('',*,*,#11432,.F.);
#16303=ORIENTED_EDGE('',*,*,#11433,.T.);
#16304=ORIENTED_EDGE('',*,*,#11429,.T.);
#16305=ORIENTED_EDGE('',*,*,#11434,.T.);
#16306=ORIENTED_EDGE('',*,*,#11435,.F.);
#16307=ORIENTED_EDGE('',*,*,#11436,.T.);
#16308=ORIENTED_EDGE('',*,*,#11432,.T.);
#16309=ORIENTED_EDGE('',*,*,#11437,.T.);
#16310=ORIENTED_EDGE('',*,*,#11438,.F.);
#16311=ORIENTED_EDGE('',*,*,#11439,.T.);
#16312=ORIENTED_EDGE('',*,*,#11435,.T.);
#16313=ORIENTED_EDGE('',*,*,#11440,.T.);
#16314=ORIENTED_EDGE('',*,*,#11441,.F.);
#16315=ORIENTED_EDGE('',*,*,#11442,.T.);
#16316=ORIENTED_EDGE('',*,*,#11438,.T.);
#16317=ORIENTED_EDGE('',*,*,#11443,.T.);
#16318=ORIENTED_EDGE('',*,*,#11444,.F.);
#16319=ORIENTED_EDGE('',*,*,#11445,.T.);
#16320=ORIENTED_EDGE('',*,*,#11441,.T.);
#16321=ORIENTED_EDGE('',*,*,#11446,.T.);
#16322=ORIENTED_EDGE('',*,*,#11447,.F.);
#16323=ORIENTED_EDGE('',*,*,#11448,.T.);
#16324=ORIENTED_EDGE('',*,*,#11444,.T.);
#16325=ORIENTED_EDGE('',*,*,#11449,.T.);
#16326=ORIENTED_EDGE('',*,*,#11450,.F.);
#16327=ORIENTED_EDGE('',*,*,#11451,.T.);
#16328=ORIENTED_EDGE('',*,*,#11447,.T.);
#16329=ORIENTED_EDGE('',*,*,#11452,.T.);
#16330=ORIENTED_EDGE('',*,*,#11453,.F.);
#16331=ORIENTED_EDGE('',*,*,#11454,.T.);
#16332=ORIENTED_EDGE('',*,*,#11450,.T.);
#16333=ORIENTED_EDGE('',*,*,#11455,.T.);
#16334=ORIENTED_EDGE('',*,*,#11456,.F.);
#16335=ORIENTED_EDGE('',*,*,#11457,.T.);
#16336=ORIENTED_EDGE('',*,*,#11453,.T.);
#16337=ORIENTED_EDGE('',*,*,#11458,.T.);
#16338=ORIENTED_EDGE('',*,*,#11459,.F.);
#16339=ORIENTED_EDGE('',*,*,#11460,.T.);
#16340=ORIENTED_EDGE('',*,*,#11456,.T.);
#16341=ORIENTED_EDGE('',*,*,#11461,.T.);
#16342=ORIENTED_EDGE('',*,*,#11462,.F.);
#16343=ORIENTED_EDGE('',*,*,#11463,.T.);
#16344=ORIENTED_EDGE('',*,*,#11459,.T.);
#16345=ORIENTED_EDGE('',*,*,#11464,.T.);
#16346=ORIENTED_EDGE('',*,*,#11465,.F.);
#16347=ORIENTED_EDGE('',*,*,#11466,.T.);
#16348=ORIENTED_EDGE('',*,*,#11462,.T.);
#16349=ORIENTED_EDGE('',*,*,#11467,.T.);
#16350=ORIENTED_EDGE('',*,*,#11468,.F.);
#16351=ORIENTED_EDGE('',*,*,#11469,.T.);
#16352=ORIENTED_EDGE('',*,*,#11465,.T.);
#16353=ORIENTED_EDGE('',*,*,#11470,.T.);
#16354=ORIENTED_EDGE('',*,*,#11471,.F.);
#16355=ORIENTED_EDGE('',*,*,#11472,.T.);
#16356=ORIENTED_EDGE('',*,*,#11468,.T.);
#16357=ORIENTED_EDGE('',*,*,#11473,.T.);
#16358=ORIENTED_EDGE('',*,*,#11474,.F.);
#16359=ORIENTED_EDGE('',*,*,#11475,.T.);
#16360=ORIENTED_EDGE('',*,*,#11471,.T.);
#16361=ORIENTED_EDGE('',*,*,#11476,.T.);
#16362=ORIENTED_EDGE('',*,*,#11477,.F.);
#16363=ORIENTED_EDGE('',*,*,#11478,.T.);
#16364=ORIENTED_EDGE('',*,*,#11474,.T.);
#16365=ORIENTED_EDGE('',*,*,#11479,.T.);
#16366=ORIENTED_EDGE('',*,*,#11480,.F.);
#16367=ORIENTED_EDGE('',*,*,#11481,.T.);
#16368=ORIENTED_EDGE('',*,*,#11477,.T.);
#16369=ORIENTED_EDGE('',*,*,#11482,.T.);
#16370=ORIENTED_EDGE('',*,*,#11483,.F.);
#16371=ORIENTED_EDGE('',*,*,#11484,.T.);
#16372=ORIENTED_EDGE('',*,*,#11480,.T.);
#16373=ORIENTED_EDGE('',*,*,#11485,.T.);
#16374=ORIENTED_EDGE('',*,*,#11486,.F.);
#16375=ORIENTED_EDGE('',*,*,#11487,.T.);
#16376=ORIENTED_EDGE('',*,*,#11483,.T.);
#16377=ORIENTED_EDGE('',*,*,#11488,.T.);
#16378=ORIENTED_EDGE('',*,*,#11489,.F.);
#16379=ORIENTED_EDGE('',*,*,#11490,.T.);
#16380=ORIENTED_EDGE('',*,*,#11486,.T.);
#16381=ORIENTED_EDGE('',*,*,#11491,.T.);
#16382=ORIENTED_EDGE('',*,*,#11492,.F.);
#16383=ORIENTED_EDGE('',*,*,#11493,.T.);
#16384=ORIENTED_EDGE('',*,*,#11489,.T.);
#16385=ORIENTED_EDGE('',*,*,#11494,.T.);
#16386=ORIENTED_EDGE('',*,*,#11495,.F.);
#16387=ORIENTED_EDGE('',*,*,#11496,.T.);
#16388=ORIENTED_EDGE('',*,*,#11492,.T.);
#16389=ORIENTED_EDGE('',*,*,#11497,.T.);
#16390=ORIENTED_EDGE('',*,*,#11498,.F.);
#16391=ORIENTED_EDGE('',*,*,#11499,.T.);
#16392=ORIENTED_EDGE('',*,*,#11495,.T.);
#16393=ORIENTED_EDGE('',*,*,#11500,.T.);
#16394=ORIENTED_EDGE('',*,*,#11501,.F.);
#16395=ORIENTED_EDGE('',*,*,#11502,.T.);
#16396=ORIENTED_EDGE('',*,*,#11498,.T.);
#16397=ORIENTED_EDGE('',*,*,#11503,.T.);
#16398=ORIENTED_EDGE('',*,*,#11504,.F.);
#16399=ORIENTED_EDGE('',*,*,#11505,.T.);
#16400=ORIENTED_EDGE('',*,*,#11501,.T.);
#16401=ORIENTED_EDGE('',*,*,#11506,.T.);
#16402=ORIENTED_EDGE('',*,*,#11507,.F.);
#16403=ORIENTED_EDGE('',*,*,#11508,.T.);
#16404=ORIENTED_EDGE('',*,*,#11504,.T.);
#16405=ORIENTED_EDGE('',*,*,#11509,.T.);
#16406=ORIENTED_EDGE('',*,*,#11510,.F.);
#16407=ORIENTED_EDGE('',*,*,#11511,.T.);
#16408=ORIENTED_EDGE('',*,*,#11507,.T.);
#16409=ORIENTED_EDGE('',*,*,#11512,.T.);
#16410=ORIENTED_EDGE('',*,*,#11513,.F.);
#16411=ORIENTED_EDGE('',*,*,#11514,.T.);
#16412=ORIENTED_EDGE('',*,*,#11510,.T.);
#16413=ORIENTED_EDGE('',*,*,#11515,.T.);
#16414=ORIENTED_EDGE('',*,*,#11516,.F.);
#16415=ORIENTED_EDGE('',*,*,#11517,.T.);
#16416=ORIENTED_EDGE('',*,*,#11513,.T.);
#16417=ORIENTED_EDGE('',*,*,#11518,.T.);
#16418=ORIENTED_EDGE('',*,*,#11519,.F.);
#16419=ORIENTED_EDGE('',*,*,#11520,.T.);
#16420=ORIENTED_EDGE('',*,*,#11516,.T.);
#16421=ORIENTED_EDGE('',*,*,#11521,.T.);
#16422=ORIENTED_EDGE('',*,*,#11522,.F.);
#16423=ORIENTED_EDGE('',*,*,#11523,.T.);
#16424=ORIENTED_EDGE('',*,*,#11519,.T.);
#16425=ORIENTED_EDGE('',*,*,#11524,.T.);
#16426=ORIENTED_EDGE('',*,*,#11525,.F.);
#16427=ORIENTED_EDGE('',*,*,#11526,.T.);
#16428=ORIENTED_EDGE('',*,*,#11522,.T.);
#16429=ORIENTED_EDGE('',*,*,#11527,.T.);
#16430=ORIENTED_EDGE('',*,*,#11528,.F.);
#16431=ORIENTED_EDGE('',*,*,#11529,.T.);
#16432=ORIENTED_EDGE('',*,*,#11525,.T.);
#16433=ORIENTED_EDGE('',*,*,#11530,.T.);
#16434=ORIENTED_EDGE('',*,*,#11531,.F.);
#16435=ORIENTED_EDGE('',*,*,#11532,.T.);
#16436=ORIENTED_EDGE('',*,*,#11528,.T.);
#16437=ORIENTED_EDGE('',*,*,#11533,.T.);
#16438=ORIENTED_EDGE('',*,*,#11534,.F.);
#16439=ORIENTED_EDGE('',*,*,#11535,.T.);
#16440=ORIENTED_EDGE('',*,*,#11531,.T.);
#16441=ORIENTED_EDGE('',*,*,#11536,.T.);
#16442=ORIENTED_EDGE('',*,*,#11537,.F.);
#16443=ORIENTED_EDGE('',*,*,#11538,.T.);
#16444=ORIENTED_EDGE('',*,*,#11534,.T.);
#16445=ORIENTED_EDGE('',*,*,#11539,.T.);
#16446=ORIENTED_EDGE('',*,*,#11540,.F.);
#16447=ORIENTED_EDGE('',*,*,#11541,.T.);
#16448=ORIENTED_EDGE('',*,*,#11537,.T.);
#16449=ORIENTED_EDGE('',*,*,#11542,.T.);
#16450=ORIENTED_EDGE('',*,*,#11543,.F.);
#16451=ORIENTED_EDGE('',*,*,#11544,.T.);
#16452=ORIENTED_EDGE('',*,*,#11545,.F.);
#16453=ORIENTED_EDGE('',*,*,#11546,.F.);
#16454=ORIENTED_EDGE('',*,*,#11547,.F.);
#16455=ORIENTED_EDGE('',*,*,#11548,.T.);
#16456=ORIENTED_EDGE('',*,*,#11543,.T.);
#16457=ORIENTED_EDGE('',*,*,#11549,.F.);
#16458=ORIENTED_EDGE('',*,*,#11550,.F.);
#16459=ORIENTED_EDGE('',*,*,#11551,.T.);
#16460=ORIENTED_EDGE('',*,*,#11547,.T.);
#16461=ORIENTED_EDGE('',*,*,#11552,.F.);
#16462=ORIENTED_EDGE('',*,*,#11553,.F.);
#16463=ORIENTED_EDGE('',*,*,#11554,.T.);
#16464=ORIENTED_EDGE('',*,*,#11550,.T.);
#16465=ORIENTED_EDGE('',*,*,#11555,.F.);
#16466=ORIENTED_EDGE('',*,*,#11556,.F.);
#16467=ORIENTED_EDGE('',*,*,#11557,.T.);
#16468=ORIENTED_EDGE('',*,*,#11553,.T.);
#16469=ORIENTED_EDGE('',*,*,#11558,.F.);
#16470=ORIENTED_EDGE('',*,*,#11559,.F.);
#16471=ORIENTED_EDGE('',*,*,#11560,.T.);
#16472=ORIENTED_EDGE('',*,*,#11556,.T.);
#16473=ORIENTED_EDGE('',*,*,#11561,.F.);
#16474=ORIENTED_EDGE('',*,*,#11562,.F.);
#16475=ORIENTED_EDGE('',*,*,#11563,.T.);
#16476=ORIENTED_EDGE('',*,*,#11559,.T.);
#16477=ORIENTED_EDGE('',*,*,#11564,.F.);
#16478=ORIENTED_EDGE('',*,*,#11565,.F.);
#16479=ORIENTED_EDGE('',*,*,#11566,.T.);
#16480=ORIENTED_EDGE('',*,*,#11562,.T.);
#16481=ORIENTED_EDGE('',*,*,#11567,.F.);
#16482=ORIENTED_EDGE('',*,*,#11568,.F.);
#16483=ORIENTED_EDGE('',*,*,#11569,.T.);
#16484=ORIENTED_EDGE('',*,*,#11565,.T.);
#16485=ORIENTED_EDGE('',*,*,#11570,.F.);
#16486=ORIENTED_EDGE('',*,*,#11571,.F.);
#16487=ORIENTED_EDGE('',*,*,#11572,.T.);
#16488=ORIENTED_EDGE('',*,*,#11568,.T.);
#16489=ORIENTED_EDGE('',*,*,#11573,.F.);
#16490=ORIENTED_EDGE('',*,*,#11574,.F.);
#16491=ORIENTED_EDGE('',*,*,#11575,.T.);
#16492=ORIENTED_EDGE('',*,*,#11571,.T.);
#16493=ORIENTED_EDGE('',*,*,#11576,.F.);
#16494=ORIENTED_EDGE('',*,*,#11577,.F.);
#16495=ORIENTED_EDGE('',*,*,#11578,.T.);
#16496=ORIENTED_EDGE('',*,*,#11574,.T.);
#16497=ORIENTED_EDGE('',*,*,#11579,.F.);
#16498=ORIENTED_EDGE('',*,*,#11580,.F.);
#16499=ORIENTED_EDGE('',*,*,#11581,.T.);
#16500=ORIENTED_EDGE('',*,*,#11577,.T.);
#16501=ORIENTED_EDGE('',*,*,#11582,.F.);
#16502=ORIENTED_EDGE('',*,*,#11583,.F.);
#16503=ORIENTED_EDGE('',*,*,#11584,.T.);
#16504=ORIENTED_EDGE('',*,*,#11580,.T.);
#16505=ORIENTED_EDGE('',*,*,#11585,.F.);
#16506=ORIENTED_EDGE('',*,*,#11586,.F.);
#16507=ORIENTED_EDGE('',*,*,#11587,.T.);
#16508=ORIENTED_EDGE('',*,*,#11583,.T.);
#16509=ORIENTED_EDGE('',*,*,#11588,.F.);
#16510=ORIENTED_EDGE('',*,*,#11589,.F.);
#16511=ORIENTED_EDGE('',*,*,#11590,.T.);
#16512=ORIENTED_EDGE('',*,*,#11586,.T.);
#16513=ORIENTED_EDGE('',*,*,#11591,.F.);
#16514=ORIENTED_EDGE('',*,*,#11592,.F.);
#16515=ORIENTED_EDGE('',*,*,#11593,.T.);
#16516=ORIENTED_EDGE('',*,*,#11589,.T.);
#16517=ORIENTED_EDGE('',*,*,#11594,.F.);
#16518=ORIENTED_EDGE('',*,*,#11595,.F.);
#16519=ORIENTED_EDGE('',*,*,#11596,.T.);
#16520=ORIENTED_EDGE('',*,*,#11592,.T.);
#16521=ORIENTED_EDGE('',*,*,#11597,.F.);
#16522=ORIENTED_EDGE('',*,*,#11598,.F.);
#16523=ORIENTED_EDGE('',*,*,#11599,.T.);
#16524=ORIENTED_EDGE('',*,*,#11595,.T.);
#16525=ORIENTED_EDGE('',*,*,#11600,.F.);
#16526=ORIENTED_EDGE('',*,*,#11601,.F.);
#16527=ORIENTED_EDGE('',*,*,#11602,.T.);
#16528=ORIENTED_EDGE('',*,*,#11598,.T.);
#16529=ORIENTED_EDGE('',*,*,#11603,.F.);
#16530=ORIENTED_EDGE('',*,*,#11604,.F.);
#16531=ORIENTED_EDGE('',*,*,#11605,.T.);
#16532=ORIENTED_EDGE('',*,*,#11601,.T.);
#16533=ORIENTED_EDGE('',*,*,#11606,.F.);
#16534=ORIENTED_EDGE('',*,*,#11607,.F.);
#16535=ORIENTED_EDGE('',*,*,#11608,.T.);
#16536=ORIENTED_EDGE('',*,*,#11604,.T.);
#16537=ORIENTED_EDGE('',*,*,#11609,.F.);
#16538=ORIENTED_EDGE('',*,*,#11610,.F.);
#16539=ORIENTED_EDGE('',*,*,#11611,.T.);
#16540=ORIENTED_EDGE('',*,*,#11607,.T.);
#16541=ORIENTED_EDGE('',*,*,#11612,.F.);
#16542=ORIENTED_EDGE('',*,*,#11613,.F.);
#16543=ORIENTED_EDGE('',*,*,#11614,.T.);
#16544=ORIENTED_EDGE('',*,*,#11610,.T.);
#16545=ORIENTED_EDGE('',*,*,#11615,.F.);
#16546=ORIENTED_EDGE('',*,*,#11616,.F.);
#16547=ORIENTED_EDGE('',*,*,#11617,.T.);
#16548=ORIENTED_EDGE('',*,*,#11613,.T.);
#16549=ORIENTED_EDGE('',*,*,#11618,.F.);
#16550=ORIENTED_EDGE('',*,*,#11619,.F.);
#16551=ORIENTED_EDGE('',*,*,#11620,.T.);
#16552=ORIENTED_EDGE('',*,*,#11616,.T.);
#16553=ORIENTED_EDGE('',*,*,#11621,.F.);
#16554=ORIENTED_EDGE('',*,*,#11622,.F.);
#16555=ORIENTED_EDGE('',*,*,#11623,.T.);
#16556=ORIENTED_EDGE('',*,*,#11619,.T.);
#16557=ORIENTED_EDGE('',*,*,#11624,.F.);
#16558=ORIENTED_EDGE('',*,*,#11625,.F.);
#16559=ORIENTED_EDGE('',*,*,#11626,.T.);
#16560=ORIENTED_EDGE('',*,*,#11622,.T.);
#16561=ORIENTED_EDGE('',*,*,#11627,.F.);
#16562=ORIENTED_EDGE('',*,*,#11628,.F.);
#16563=ORIENTED_EDGE('',*,*,#11629,.T.);
#16564=ORIENTED_EDGE('',*,*,#11625,.T.);
#16565=ORIENTED_EDGE('',*,*,#11630,.F.);
#16566=ORIENTED_EDGE('',*,*,#11631,.F.);
#16567=ORIENTED_EDGE('',*,*,#11632,.T.);
#16568=ORIENTED_EDGE('',*,*,#11628,.T.);
#16569=ORIENTED_EDGE('',*,*,#11633,.F.);
#16570=ORIENTED_EDGE('',*,*,#11634,.F.);
#16571=ORIENTED_EDGE('',*,*,#11635,.T.);
#16572=ORIENTED_EDGE('',*,*,#11631,.T.);
#16573=ORIENTED_EDGE('',*,*,#11636,.F.);
#16574=ORIENTED_EDGE('',*,*,#11637,.F.);
#16575=ORIENTED_EDGE('',*,*,#11638,.T.);
#16576=ORIENTED_EDGE('',*,*,#11634,.T.);
#16577=ORIENTED_EDGE('',*,*,#11639,.F.);
#16578=ORIENTED_EDGE('',*,*,#11640,.F.);
#16579=ORIENTED_EDGE('',*,*,#11641,.T.);
#16580=ORIENTED_EDGE('',*,*,#11637,.T.);
#16581=ORIENTED_EDGE('',*,*,#11642,.F.);
#16582=ORIENTED_EDGE('',*,*,#11643,.F.);
#16583=ORIENTED_EDGE('',*,*,#11644,.T.);
#16584=ORIENTED_EDGE('',*,*,#11640,.T.);
#16585=ORIENTED_EDGE('',*,*,#11645,.F.);
#16586=ORIENTED_EDGE('',*,*,#11646,.F.);
#16587=ORIENTED_EDGE('',*,*,#11647,.T.);
#16588=ORIENTED_EDGE('',*,*,#11643,.T.);
#16589=ORIENTED_EDGE('',*,*,#11648,.F.);
#16590=ORIENTED_EDGE('',*,*,#11649,.F.);
#16591=ORIENTED_EDGE('',*,*,#11650,.T.);
#16592=ORIENTED_EDGE('',*,*,#11646,.T.);
#16593=ORIENTED_EDGE('',*,*,#11651,.F.);
#16594=ORIENTED_EDGE('',*,*,#11652,.F.);
#16595=ORIENTED_EDGE('',*,*,#11653,.T.);
#16596=ORIENTED_EDGE('',*,*,#11649,.T.);
#16597=ORIENTED_EDGE('',*,*,#11654,.F.);
#16598=ORIENTED_EDGE('',*,*,#11655,.F.);
#16599=ORIENTED_EDGE('',*,*,#11656,.T.);
#16600=ORIENTED_EDGE('',*,*,#11652,.T.);
#16601=ORIENTED_EDGE('',*,*,#11657,.F.);
#16602=ORIENTED_EDGE('',*,*,#11658,.F.);
#16603=ORIENTED_EDGE('',*,*,#11659,.T.);
#16604=ORIENTED_EDGE('',*,*,#11655,.T.);
#16605=ORIENTED_EDGE('',*,*,#11660,.F.);
#16606=ORIENTED_EDGE('',*,*,#11661,.F.);
#16607=ORIENTED_EDGE('',*,*,#11662,.T.);
#16608=ORIENTED_EDGE('',*,*,#11658,.T.);
#16609=ORIENTED_EDGE('',*,*,#11663,.F.);
#16610=ORIENTED_EDGE('',*,*,#11664,.F.);
#16611=ORIENTED_EDGE('',*,*,#11665,.T.);
#16612=ORIENTED_EDGE('',*,*,#11661,.T.);
#16613=ORIENTED_EDGE('',*,*,#11666,.F.);
#16614=ORIENTED_EDGE('',*,*,#11667,.F.);
#16615=ORIENTED_EDGE('',*,*,#11668,.T.);
#16616=ORIENTED_EDGE('',*,*,#11664,.T.);
#16617=ORIENTED_EDGE('',*,*,#11669,.F.);
#16618=ORIENTED_EDGE('',*,*,#11670,.F.);
#16619=ORIENTED_EDGE('',*,*,#11671,.T.);
#16620=ORIENTED_EDGE('',*,*,#11667,.T.);
#16621=ORIENTED_EDGE('',*,*,#11672,.F.);
#16622=ORIENTED_EDGE('',*,*,#11673,.F.);
#16623=ORIENTED_EDGE('',*,*,#11674,.T.);
#16624=ORIENTED_EDGE('',*,*,#11670,.T.);
#16625=ORIENTED_EDGE('',*,*,#11675,.F.);
#16626=ORIENTED_EDGE('',*,*,#11676,.F.);
#16627=ORIENTED_EDGE('',*,*,#11677,.T.);
#16628=ORIENTED_EDGE('',*,*,#11673,.T.);
#16629=ORIENTED_EDGE('',*,*,#11678,.F.);
#16630=ORIENTED_EDGE('',*,*,#11679,.F.);
#16631=ORIENTED_EDGE('',*,*,#11680,.T.);
#16632=ORIENTED_EDGE('',*,*,#11676,.T.);
#16633=ORIENTED_EDGE('',*,*,#11681,.F.);
#16634=ORIENTED_EDGE('',*,*,#11682,.F.);
#16635=ORIENTED_EDGE('',*,*,#11683,.T.);
#16636=ORIENTED_EDGE('',*,*,#11679,.T.);
#16637=ORIENTED_EDGE('',*,*,#11684,.F.);
#16638=ORIENTED_EDGE('',*,*,#11685,.F.);
#16639=ORIENTED_EDGE('',*,*,#11686,.T.);
#16640=ORIENTED_EDGE('',*,*,#11682,.T.);
#16641=ORIENTED_EDGE('',*,*,#11687,.F.);
#16642=ORIENTED_EDGE('',*,*,#11688,.F.);
#16643=ORIENTED_EDGE('',*,*,#11689,.T.);
#16644=ORIENTED_EDGE('',*,*,#11685,.T.);
#16645=ORIENTED_EDGE('',*,*,#11690,.F.);
#16646=ORIENTED_EDGE('',*,*,#11691,.F.);
#16647=ORIENTED_EDGE('',*,*,#11692,.T.);
#16648=ORIENTED_EDGE('',*,*,#11688,.T.);
#16649=ORIENTED_EDGE('',*,*,#11693,.F.);
#16650=ORIENTED_EDGE('',*,*,#11694,.F.);
#16651=ORIENTED_EDGE('',*,*,#11695,.T.);
#16652=ORIENTED_EDGE('',*,*,#11691,.T.);
#16653=ORIENTED_EDGE('',*,*,#11696,.F.);
#16654=ORIENTED_EDGE('',*,*,#11697,.F.);
#16655=ORIENTED_EDGE('',*,*,#11698,.T.);
#16656=ORIENTED_EDGE('',*,*,#11694,.T.);
#16657=ORIENTED_EDGE('',*,*,#11699,.F.);
#16658=ORIENTED_EDGE('',*,*,#11700,.F.);
#16659=ORIENTED_EDGE('',*,*,#11701,.T.);
#16660=ORIENTED_EDGE('',*,*,#11697,.T.);
#16661=ORIENTED_EDGE('',*,*,#11702,.F.);
#16662=ORIENTED_EDGE('',*,*,#11703,.F.);
#16663=ORIENTED_EDGE('',*,*,#11704,.T.);
#16664=ORIENTED_EDGE('',*,*,#11700,.T.);
#16665=ORIENTED_EDGE('',*,*,#11705,.F.);
#16666=ORIENTED_EDGE('',*,*,#11706,.F.);
#16667=ORIENTED_EDGE('',*,*,#11707,.T.);
#16668=ORIENTED_EDGE('',*,*,#11703,.T.);
#16669=ORIENTED_EDGE('',*,*,#11708,.F.);
#16670=ORIENTED_EDGE('',*,*,#11709,.F.);
#16671=ORIENTED_EDGE('',*,*,#11710,.T.);
#16672=ORIENTED_EDGE('',*,*,#11706,.T.);
#16673=ORIENTED_EDGE('',*,*,#11711,.F.);
#16674=ORIENTED_EDGE('',*,*,#11712,.F.);
#16675=ORIENTED_EDGE('',*,*,#11713,.T.);
#16676=ORIENTED_EDGE('',*,*,#11709,.T.);
#16677=ORIENTED_EDGE('',*,*,#11714,.F.);
#16678=ORIENTED_EDGE('',*,*,#11715,.F.);
#16679=ORIENTED_EDGE('',*,*,#11716,.T.);
#16680=ORIENTED_EDGE('',*,*,#11712,.T.);
#16681=ORIENTED_EDGE('',*,*,#11717,.F.);
#16682=ORIENTED_EDGE('',*,*,#11718,.F.);
#16683=ORIENTED_EDGE('',*,*,#11719,.T.);
#16684=ORIENTED_EDGE('',*,*,#11715,.T.);
#16685=ORIENTED_EDGE('',*,*,#11720,.F.);
#16686=ORIENTED_EDGE('',*,*,#11721,.F.);
#16687=ORIENTED_EDGE('',*,*,#11722,.T.);
#16688=ORIENTED_EDGE('',*,*,#11718,.T.);
#16689=ORIENTED_EDGE('',*,*,#11723,.F.);
#16690=ORIENTED_EDGE('',*,*,#11724,.F.);
#16691=ORIENTED_EDGE('',*,*,#11725,.F.);
#16692=ORIENTED_EDGE('',*,*,#11542,.F.);
#16693=ORIENTED_EDGE('',*,*,#11539,.F.);
#16694=ORIENTED_EDGE('',*,*,#11536,.F.);
#16695=ORIENTED_EDGE('',*,*,#11533,.F.);
#16696=ORIENTED_EDGE('',*,*,#11530,.F.);
#16697=ORIENTED_EDGE('',*,*,#11527,.F.);
#16698=ORIENTED_EDGE('',*,*,#11524,.F.);
#16699=ORIENTED_EDGE('',*,*,#11521,.F.);
#16700=ORIENTED_EDGE('',*,*,#11518,.F.);
#16701=ORIENTED_EDGE('',*,*,#11515,.F.);
#16702=ORIENTED_EDGE('',*,*,#11512,.F.);
#16703=ORIENTED_EDGE('',*,*,#11509,.F.);
#16704=ORIENTED_EDGE('',*,*,#11506,.F.);
#16705=ORIENTED_EDGE('',*,*,#11503,.F.);
#16706=ORIENTED_EDGE('',*,*,#11500,.F.);
#16707=ORIENTED_EDGE('',*,*,#11497,.F.);
#16708=ORIENTED_EDGE('',*,*,#11494,.F.);
#16709=ORIENTED_EDGE('',*,*,#11491,.F.);
#16710=ORIENTED_EDGE('',*,*,#11488,.F.);
#16711=ORIENTED_EDGE('',*,*,#11485,.F.);
#16712=ORIENTED_EDGE('',*,*,#11482,.F.);
#16713=ORIENTED_EDGE('',*,*,#11479,.F.);
#16714=ORIENTED_EDGE('',*,*,#11476,.F.);
#16715=ORIENTED_EDGE('',*,*,#11473,.F.);
#16716=ORIENTED_EDGE('',*,*,#11470,.F.);
#16717=ORIENTED_EDGE('',*,*,#11467,.F.);
#16718=ORIENTED_EDGE('',*,*,#11464,.F.);
#16719=ORIENTED_EDGE('',*,*,#11461,.F.);
#16720=ORIENTED_EDGE('',*,*,#11458,.F.);
#16721=ORIENTED_EDGE('',*,*,#11455,.F.);
#16722=ORIENTED_EDGE('',*,*,#11452,.F.);
#16723=ORIENTED_EDGE('',*,*,#11449,.F.);
#16724=ORIENTED_EDGE('',*,*,#11446,.F.);
#16725=ORIENTED_EDGE('',*,*,#11443,.F.);
#16726=ORIENTED_EDGE('',*,*,#11440,.F.);
#16727=ORIENTED_EDGE('',*,*,#11437,.F.);
#16728=ORIENTED_EDGE('',*,*,#11434,.F.);
#16729=ORIENTED_EDGE('',*,*,#11431,.F.);
#16730=ORIENTED_EDGE('',*,*,#11428,.F.);
#16731=ORIENTED_EDGE('',*,*,#11425,.F.);
#16732=ORIENTED_EDGE('',*,*,#11422,.F.);
#16733=ORIENTED_EDGE('',*,*,#11419,.F.);
#16734=ORIENTED_EDGE('',*,*,#11416,.F.);
#16735=ORIENTED_EDGE('',*,*,#11413,.F.);
#16736=ORIENTED_EDGE('',*,*,#11410,.F.);
#16737=ORIENTED_EDGE('',*,*,#11407,.F.);
#16738=ORIENTED_EDGE('',*,*,#11404,.F.);
#16739=ORIENTED_EDGE('',*,*,#11401,.F.);
#16740=ORIENTED_EDGE('',*,*,#11398,.F.);
#16741=ORIENTED_EDGE('',*,*,#11395,.F.);
#16742=ORIENTED_EDGE('',*,*,#11392,.F.);
#16743=ORIENTED_EDGE('',*,*,#11389,.F.);
#16744=ORIENTED_EDGE('',*,*,#11386,.F.);
#16745=ORIENTED_EDGE('',*,*,#11383,.F.);
#16746=ORIENTED_EDGE('',*,*,#11380,.F.);
#16747=ORIENTED_EDGE('',*,*,#11377,.F.);
#16748=ORIENTED_EDGE('',*,*,#11374,.F.);
#16749=ORIENTED_EDGE('',*,*,#11371,.F.);
#16750=ORIENTED_EDGE('',*,*,#11368,.F.);
#16751=ORIENTED_EDGE('',*,*,#11365,.F.);
#16752=ORIENTED_EDGE('',*,*,#11726,.F.);
#16753=ORIENTED_EDGE('',*,*,#11727,.T.);
#16754=ORIENTED_EDGE('',*,*,#11723,.T.);
#16755=ORIENTED_EDGE('',*,*,#11720,.T.);
#16756=ORIENTED_EDGE('',*,*,#11717,.T.);
#16757=ORIENTED_EDGE('',*,*,#11714,.T.);
#16758=ORIENTED_EDGE('',*,*,#11711,.T.);
#16759=ORIENTED_EDGE('',*,*,#11708,.T.);
#16760=ORIENTED_EDGE('',*,*,#11705,.T.);
#16761=ORIENTED_EDGE('',*,*,#11702,.T.);
#16762=ORIENTED_EDGE('',*,*,#11699,.T.);
#16763=ORIENTED_EDGE('',*,*,#11696,.T.);
#16764=ORIENTED_EDGE('',*,*,#11693,.T.);
#16765=ORIENTED_EDGE('',*,*,#11690,.T.);
#16766=ORIENTED_EDGE('',*,*,#11687,.T.);
#16767=ORIENTED_EDGE('',*,*,#11684,.T.);
#16768=ORIENTED_EDGE('',*,*,#11681,.T.);
#16769=ORIENTED_EDGE('',*,*,#11678,.T.);
#16770=ORIENTED_EDGE('',*,*,#11675,.T.);
#16771=ORIENTED_EDGE('',*,*,#11672,.T.);
#16772=ORIENTED_EDGE('',*,*,#11669,.T.);
#16773=ORIENTED_EDGE('',*,*,#11666,.T.);
#16774=ORIENTED_EDGE('',*,*,#11663,.T.);
#16775=ORIENTED_EDGE('',*,*,#11660,.T.);
#16776=ORIENTED_EDGE('',*,*,#11657,.T.);
#16777=ORIENTED_EDGE('',*,*,#11654,.T.);
#16778=ORIENTED_EDGE('',*,*,#11651,.T.);
#16779=ORIENTED_EDGE('',*,*,#11648,.T.);
#16780=ORIENTED_EDGE('',*,*,#11645,.T.);
#16781=ORIENTED_EDGE('',*,*,#11642,.T.);
#16782=ORIENTED_EDGE('',*,*,#11639,.T.);
#16783=ORIENTED_EDGE('',*,*,#11636,.T.);
#16784=ORIENTED_EDGE('',*,*,#11633,.T.);
#16785=ORIENTED_EDGE('',*,*,#11630,.T.);
#16786=ORIENTED_EDGE('',*,*,#11627,.T.);
#16787=ORIENTED_EDGE('',*,*,#11624,.T.);
#16788=ORIENTED_EDGE('',*,*,#11621,.T.);
#16789=ORIENTED_EDGE('',*,*,#11618,.T.);
#16790=ORIENTED_EDGE('',*,*,#11615,.T.);
#16791=ORIENTED_EDGE('',*,*,#11612,.T.);
#16792=ORIENTED_EDGE('',*,*,#11609,.T.);
#16793=ORIENTED_EDGE('',*,*,#11606,.T.);
#16794=ORIENTED_EDGE('',*,*,#11603,.T.);
#16795=ORIENTED_EDGE('',*,*,#11600,.T.);
#16796=ORIENTED_EDGE('',*,*,#11597,.T.);
#16797=ORIENTED_EDGE('',*,*,#11594,.T.);
#16798=ORIENTED_EDGE('',*,*,#11591,.T.);
#16799=ORIENTED_EDGE('',*,*,#11588,.T.);
#16800=ORIENTED_EDGE('',*,*,#11585,.T.);
#16801=ORIENTED_EDGE('',*,*,#11582,.T.);
#16802=ORIENTED_EDGE('',*,*,#11579,.T.);
#16803=ORIENTED_EDGE('',*,*,#11576,.T.);
#16804=ORIENTED_EDGE('',*,*,#11573,.T.);
#16805=ORIENTED_EDGE('',*,*,#11570,.T.);
#16806=ORIENTED_EDGE('',*,*,#11567,.T.);
#16807=ORIENTED_EDGE('',*,*,#11564,.T.);
#16808=ORIENTED_EDGE('',*,*,#11561,.T.);
#16809=ORIENTED_EDGE('',*,*,#11558,.T.);
#16810=ORIENTED_EDGE('',*,*,#11555,.T.);
#16811=ORIENTED_EDGE('',*,*,#11552,.T.);
#16812=ORIENTED_EDGE('',*,*,#11549,.T.);
#16813=ORIENTED_EDGE('',*,*,#11546,.T.);
#16814=ORIENTED_EDGE('',*,*,#11721,.T.);
#16815=ORIENTED_EDGE('',*,*,#11727,.F.);
#16816=ORIENTED_EDGE('',*,*,#11728,.F.);
#16817=ORIENTED_EDGE('',*,*,#11729,.T.);
#16818=ORIENTED_EDGE('',*,*,#11730,.F.);
#16819=ORIENTED_EDGE('',*,*,#11544,.F.);
#16820=ORIENTED_EDGE('',*,*,#11548,.F.);
#16821=ORIENTED_EDGE('',*,*,#11551,.F.);
#16822=ORIENTED_EDGE('',*,*,#11554,.F.);
#16823=ORIENTED_EDGE('',*,*,#11557,.F.);
#16824=ORIENTED_EDGE('',*,*,#11560,.F.);
#16825=ORIENTED_EDGE('',*,*,#11563,.F.);
#16826=ORIENTED_EDGE('',*,*,#11566,.F.);
#16827=ORIENTED_EDGE('',*,*,#11569,.F.);
#16828=ORIENTED_EDGE('',*,*,#11572,.F.);
#16829=ORIENTED_EDGE('',*,*,#11575,.F.);
#16830=ORIENTED_EDGE('',*,*,#11578,.F.);
#16831=ORIENTED_EDGE('',*,*,#11581,.F.);
#16832=ORIENTED_EDGE('',*,*,#11584,.F.);
#16833=ORIENTED_EDGE('',*,*,#11587,.F.);
#16834=ORIENTED_EDGE('',*,*,#11590,.F.);
#16835=ORIENTED_EDGE('',*,*,#11593,.F.);
#16836=ORIENTED_EDGE('',*,*,#11596,.F.);
#16837=ORIENTED_EDGE('',*,*,#11599,.F.);
#16838=ORIENTED_EDGE('',*,*,#11602,.F.);
#16839=ORIENTED_EDGE('',*,*,#11605,.F.);
#16840=ORIENTED_EDGE('',*,*,#11608,.F.);
#16841=ORIENTED_EDGE('',*,*,#11611,.F.);
#16842=ORIENTED_EDGE('',*,*,#11614,.F.);
#16843=ORIENTED_EDGE('',*,*,#11617,.F.);
#16844=ORIENTED_EDGE('',*,*,#11620,.F.);
#16845=ORIENTED_EDGE('',*,*,#11623,.F.);
#16846=ORIENTED_EDGE('',*,*,#11626,.F.);
#16847=ORIENTED_EDGE('',*,*,#11629,.F.);
#16848=ORIENTED_EDGE('',*,*,#11632,.F.);
#16849=ORIENTED_EDGE('',*,*,#11635,.F.);
#16850=ORIENTED_EDGE('',*,*,#11638,.F.);
#16851=ORIENTED_EDGE('',*,*,#11641,.F.);
#16852=ORIENTED_EDGE('',*,*,#11644,.F.);
#16853=ORIENTED_EDGE('',*,*,#11647,.F.);
#16854=ORIENTED_EDGE('',*,*,#11650,.F.);
#16855=ORIENTED_EDGE('',*,*,#11653,.F.);
#16856=ORIENTED_EDGE('',*,*,#11656,.F.);
#16857=ORIENTED_EDGE('',*,*,#11659,.F.);
#16858=ORIENTED_EDGE('',*,*,#11662,.F.);
#16859=ORIENTED_EDGE('',*,*,#11665,.F.);
#16860=ORIENTED_EDGE('',*,*,#11668,.F.);
#16861=ORIENTED_EDGE('',*,*,#11671,.F.);
#16862=ORIENTED_EDGE('',*,*,#11674,.F.);
#16863=ORIENTED_EDGE('',*,*,#11677,.F.);
#16864=ORIENTED_EDGE('',*,*,#11680,.F.);
#16865=ORIENTED_EDGE('',*,*,#11683,.F.);
#16866=ORIENTED_EDGE('',*,*,#11686,.F.);
#16867=ORIENTED_EDGE('',*,*,#11689,.F.);
#16868=ORIENTED_EDGE('',*,*,#11692,.F.);
#16869=ORIENTED_EDGE('',*,*,#11695,.F.);
#16870=ORIENTED_EDGE('',*,*,#11698,.F.);
#16871=ORIENTED_EDGE('',*,*,#11701,.F.);
#16872=ORIENTED_EDGE('',*,*,#11704,.F.);
#16873=ORIENTED_EDGE('',*,*,#11707,.F.);
#16874=ORIENTED_EDGE('',*,*,#11710,.F.);
#16875=ORIENTED_EDGE('',*,*,#11713,.F.);
#16876=ORIENTED_EDGE('',*,*,#11716,.F.);
#16877=ORIENTED_EDGE('',*,*,#11719,.F.);
#16878=ORIENTED_EDGE('',*,*,#11722,.F.);
#16879=ORIENTED_EDGE('',*,*,#11729,.F.);
#16880=ORIENTED_EDGE('',*,*,#11731,.F.);
#16881=ORIENTED_EDGE('',*,*,#11363,.F.);
#16882=ORIENTED_EDGE('',*,*,#11367,.F.);
#16883=ORIENTED_EDGE('',*,*,#11370,.F.);
#16884=ORIENTED_EDGE('',*,*,#11373,.F.);
#16885=ORIENTED_EDGE('',*,*,#11376,.F.);
#16886=ORIENTED_EDGE('',*,*,#11379,.F.);
#16887=ORIENTED_EDGE('',*,*,#11382,.F.);
#16888=ORIENTED_EDGE('',*,*,#11385,.F.);
#16889=ORIENTED_EDGE('',*,*,#11388,.F.);
#16890=ORIENTED_EDGE('',*,*,#11391,.F.);
#16891=ORIENTED_EDGE('',*,*,#11394,.F.);
#16892=ORIENTED_EDGE('',*,*,#11397,.F.);
#16893=ORIENTED_EDGE('',*,*,#11400,.F.);
#16894=ORIENTED_EDGE('',*,*,#11403,.F.);
#16895=ORIENTED_EDGE('',*,*,#11406,.F.);
#16896=ORIENTED_EDGE('',*,*,#11409,.F.);
#16897=ORIENTED_EDGE('',*,*,#11412,.F.);
#16898=ORIENTED_EDGE('',*,*,#11415,.F.);
#16899=ORIENTED_EDGE('',*,*,#11418,.F.);
#16900=ORIENTED_EDGE('',*,*,#11421,.F.);
#16901=ORIENTED_EDGE('',*,*,#11424,.F.);
#16902=ORIENTED_EDGE('',*,*,#11427,.F.);
#16903=ORIENTED_EDGE('',*,*,#11430,.F.);
#16904=ORIENTED_EDGE('',*,*,#11433,.F.);
#16905=ORIENTED_EDGE('',*,*,#11436,.F.);
#16906=ORIENTED_EDGE('',*,*,#11439,.F.);
#16907=ORIENTED_EDGE('',*,*,#11442,.F.);
#16908=ORIENTED_EDGE('',*,*,#11445,.F.);
#16909=ORIENTED_EDGE('',*,*,#11448,.F.);
#16910=ORIENTED_EDGE('',*,*,#11451,.F.);
#16911=ORIENTED_EDGE('',*,*,#11454,.F.);
#16912=ORIENTED_EDGE('',*,*,#11457,.F.);
#16913=ORIENTED_EDGE('',*,*,#11460,.F.);
#16914=ORIENTED_EDGE('',*,*,#11463,.F.);
#16915=ORIENTED_EDGE('',*,*,#11466,.F.);
#16916=ORIENTED_EDGE('',*,*,#11469,.F.);
#16917=ORIENTED_EDGE('',*,*,#11472,.F.);
#16918=ORIENTED_EDGE('',*,*,#11475,.F.);
#16919=ORIENTED_EDGE('',*,*,#11478,.F.);
#16920=ORIENTED_EDGE('',*,*,#11481,.F.);
#16921=ORIENTED_EDGE('',*,*,#11484,.F.);
#16922=ORIENTED_EDGE('',*,*,#11487,.F.);
#16923=ORIENTED_EDGE('',*,*,#11490,.F.);
#16924=ORIENTED_EDGE('',*,*,#11493,.F.);
#16925=ORIENTED_EDGE('',*,*,#11496,.F.);
#16926=ORIENTED_EDGE('',*,*,#11499,.F.);
#16927=ORIENTED_EDGE('',*,*,#11502,.F.);
#16928=ORIENTED_EDGE('',*,*,#11505,.F.);
#16929=ORIENTED_EDGE('',*,*,#11508,.F.);
#16930=ORIENTED_EDGE('',*,*,#11511,.F.);
#16931=ORIENTED_EDGE('',*,*,#11514,.F.);
#16932=ORIENTED_EDGE('',*,*,#11517,.F.);
#16933=ORIENTED_EDGE('',*,*,#11520,.F.);
#16934=ORIENTED_EDGE('',*,*,#11523,.F.);
#16935=ORIENTED_EDGE('',*,*,#11526,.F.);
#16936=ORIENTED_EDGE('',*,*,#11529,.F.);
#16937=ORIENTED_EDGE('',*,*,#11532,.F.);
#16938=ORIENTED_EDGE('',*,*,#11535,.F.);
#16939=ORIENTED_EDGE('',*,*,#11538,.F.);
#16940=ORIENTED_EDGE('',*,*,#11541,.F.);
#16941=ORIENTED_EDGE('',*,*,#11732,.F.);
#16942=ORIENTED_EDGE('',*,*,#11540,.T.);
#16943=ORIENTED_EDGE('',*,*,#11725,.T.);
#16944=ORIENTED_EDGE('',*,*,#11733,.F.);
#16945=ORIENTED_EDGE('',*,*,#11732,.T.);
#16946=ORIENTED_EDGE('',*,*,#11734,.T.);
#16947=ORIENTED_EDGE('',*,*,#11735,.T.);
#16948=ORIENTED_EDGE('',*,*,#11736,.T.);
#16949=ORIENTED_EDGE('',*,*,#11737,.T.);
#16950=ORIENTED_EDGE('',*,*,#11738,.T.);
#16951=ORIENTED_EDGE('',*,*,#11739,.T.);
#16952=ORIENTED_EDGE('',*,*,#11731,.T.);
#16953=ORIENTED_EDGE('',*,*,#11728,.T.);
#16954=ORIENTED_EDGE('',*,*,#11726,.T.);
#16955=ORIENTED_EDGE('',*,*,#11364,.F.);
#16956=ORIENTED_EDGE('',*,*,#11740,.F.);
#16957=ORIENTED_EDGE('',*,*,#11741,.F.);
#16958=ORIENTED_EDGE('',*,*,#11742,.F.);
#16959=ORIENTED_EDGE('',*,*,#11743,.F.);
#16960=ORIENTED_EDGE('',*,*,#11744,.F.);
#16961=ORIENTED_EDGE('',*,*,#11745,.F.);
#16962=ORIENTED_EDGE('',*,*,#11746,.F.);
#16963=ORIENTED_EDGE('',*,*,#11741,.T.);
#16964=ORIENTED_EDGE('',*,*,#11747,.T.);
#16965=ORIENTED_EDGE('',*,*,#11739,.F.);
#16966=ORIENTED_EDGE('',*,*,#11748,.F.);
#16967=ORIENTED_EDGE('',*,*,#11742,.T.);
#16968=ORIENTED_EDGE('',*,*,#11748,.T.);
#16969=ORIENTED_EDGE('',*,*,#11738,.F.);
#16970=ORIENTED_EDGE('',*,*,#11749,.F.);
#16971=ORIENTED_EDGE('',*,*,#11743,.T.);
#16972=ORIENTED_EDGE('',*,*,#11749,.T.);
#16973=ORIENTED_EDGE('',*,*,#11737,.F.);
#16974=ORIENTED_EDGE('',*,*,#11750,.F.);
#16975=ORIENTED_EDGE('',*,*,#11744,.T.);
#16976=ORIENTED_EDGE('',*,*,#11750,.T.);
#16977=ORIENTED_EDGE('',*,*,#11736,.F.);
#16978=ORIENTED_EDGE('',*,*,#11751,.F.);
#16979=ORIENTED_EDGE('',*,*,#11745,.T.);
#16980=ORIENTED_EDGE('',*,*,#11751,.T.);
#16981=ORIENTED_EDGE('',*,*,#11735,.F.);
#16982=ORIENTED_EDGE('',*,*,#11752,.F.);
#16983=ORIENTED_EDGE('',*,*,#11740,.T.);
#16984=ORIENTED_EDGE('',*,*,#11752,.T.);
#16985=ORIENTED_EDGE('',*,*,#11734,.F.);
#16986=ORIENTED_EDGE('',*,*,#11747,.F.);
#16987=ORIENTED_EDGE('',*,*,#11746,.T.);
#16988=ORIENTED_EDGE('',*,*,#11753,.T.);
#16989=ORIENTED_EDGE('',*,*,#11754,.F.);
#16990=ORIENTED_EDGE('',*,*,#11753,.F.);
#16991=ORIENTED_EDGE('',*,*,#11730,.T.);
#16992=ORIENTED_EDGE('',*,*,#11733,.T.);
#16993=ORIENTED_EDGE('',*,*,#11724,.T.);
#16994=ORIENTED_EDGE('',*,*,#11545,.T.);
#16995=ORIENTED_EDGE('',*,*,#11754,.T.);
#16996=ORIENTED_EDGE('',*,*,#11755,.T.);
#16997=ORIENTED_EDGE('',*,*,#11755,.F.);
#20124=CYLINDRICAL_SURFACE('',#22810,4.942);
#20125=CYLINDRICAL_SURFACE('',#22812,4.942);
#20126=CYLINDRICAL_SURFACE('',#22813,4.942);
#20127=CYLINDRICAL_SURFACE('',#22814,4.942);
#20128=CYLINDRICAL_SURFACE('',#22815,4.942);
#20129=CYLINDRICAL_SURFACE('',#22816,4.942);
#20130=CYLINDRICAL_SURFACE('',#22817,4.942);
#20131=CYLINDRICAL_SURFACE('',#22818,4.942);
#20132=CYLINDRICAL_SURFACE('',#22819,4.942);
#20133=CYLINDRICAL_SURFACE('',#22820,4.942);
#20134=CYLINDRICAL_SURFACE('',#22821,4.942);
#20135=CYLINDRICAL_SURFACE('',#22822,4.942);
#20136=CYLINDRICAL_SURFACE('',#22823,4.942);
#20137=CYLINDRICAL_SURFACE('',#22824,4.942);
#20138=CYLINDRICAL_SURFACE('',#22825,4.942);
#20139=CYLINDRICAL_SURFACE('',#22826,4.942);
#20140=CYLINDRICAL_SURFACE('',#22827,4.942);
#20141=CYLINDRICAL_SURFACE('',#22828,4.942);
#20142=CYLINDRICAL_SURFACE('',#22829,4.942);
#20143=CYLINDRICAL_SURFACE('',#22830,4.942);
#20144=CYLINDRICAL_SURFACE('',#22831,4.942);
#20145=CYLINDRICAL_SURFACE('',#22832,4.942);
#20146=CYLINDRICAL_SURFACE('',#22833,4.942);
#20147=CYLINDRICAL_SURFACE('',#22834,4.942);
#20148=CYLINDRICAL_SURFACE('',#22835,4.942);
#20149=CYLINDRICAL_SURFACE('',#22836,4.942);
#20150=CYLINDRICAL_SURFACE('',#22837,4.942);
#20151=CYLINDRICAL_SURFACE('',#22838,4.942);
#20152=CYLINDRICAL_SURFACE('',#22839,4.942);
#20153=CYLINDRICAL_SURFACE('',#22840,4.942);
#20154=CYLINDRICAL_SURFACE('',#22841,4.942);
#20155=CYLINDRICAL_SURFACE('',#22842,4.942);
#20156=CYLINDRICAL_SURFACE('',#22843,4.942);
#20157=CYLINDRICAL_SURFACE('',#22844,4.942);
#20158=CYLINDRICAL_SURFACE('',#22845,4.942);
#20159=CYLINDRICAL_SURFACE('',#22846,4.942);
#20160=CYLINDRICAL_SURFACE('',#22847,4.942);
#20161=CYLINDRICAL_SURFACE('',#22848,4.942);
#20162=CYLINDRICAL_SURFACE('',#22849,4.942);
#20163=CYLINDRICAL_SURFACE('',#22850,4.942);
#20164=CYLINDRICAL_SURFACE('',#22851,4.942);
#20165=CYLINDRICAL_SURFACE('',#22852,4.942);
#20166=CYLINDRICAL_SURFACE('',#22853,4.942);
#20167=CYLINDRICAL_SURFACE('',#22854,4.942);
#20168=CYLINDRICAL_SURFACE('',#22855,4.942);
#20169=CYLINDRICAL_SURFACE('',#22856,4.942);
#20170=CYLINDRICAL_SURFACE('',#22857,4.942);
#20171=CYLINDRICAL_SURFACE('',#22858,4.942);
#20172=CYLINDRICAL_SURFACE('',#22859,4.942);
#20173=CYLINDRICAL_SURFACE('',#22860,4.942);
#20174=CYLINDRICAL_SURFACE('',#22861,4.942);
#20175=CYLINDRICAL_SURFACE('',#22862,4.942);
#20176=CYLINDRICAL_SURFACE('',#22863,4.942);
#20177=CYLINDRICAL_SURFACE('',#22864,4.942);
#20178=CYLINDRICAL_SURFACE('',#22865,4.942);
#20179=CYLINDRICAL_SURFACE('',#22866,4.942);
#20180=CYLINDRICAL_SURFACE('',#22867,4.942);
#20181=CYLINDRICAL_SURFACE('',#22868,4.942);
#20182=CYLINDRICAL_SURFACE('',#22869,4.942);
#20183=CYLINDRICAL_SURFACE('',#22870,4.942);
#20184=CYLINDRICAL_SURFACE('',#22871,4.372);
#20185=CYLINDRICAL_SURFACE('',#22873,4.372);
#20186=CYLINDRICAL_SURFACE('',#22874,4.372);
#20187=CYLINDRICAL_SURFACE('',#22875,4.372);
#20188=CYLINDRICAL_SURFACE('',#22876,4.372);
#20189=CYLINDRICAL_SURFACE('',#22877,4.372);
#20190=CYLINDRICAL_SURFACE('',#22878,4.372);
#20191=CYLINDRICAL_SURFACE('',#22879,4.372);
#20192=CYLINDRICAL_SURFACE('',#22880,4.372);
#20193=CYLINDRICAL_SURFACE('',#22881,4.372);
#20194=CYLINDRICAL_SURFACE('',#22882,4.372);
#20195=CYLINDRICAL_SURFACE('',#22883,4.372);
#20196=CYLINDRICAL_SURFACE('',#22884,4.372);
#20197=CYLINDRICAL_SURFACE('',#22885,4.372);
#20198=CYLINDRICAL_SURFACE('',#22886,4.372);
#20199=CYLINDRICAL_SURFACE('',#22887,4.372);
#20200=CYLINDRICAL_SURFACE('',#22888,4.372);
#20201=CYLINDRICAL_SURFACE('',#22889,4.372);
#20202=CYLINDRICAL_SURFACE('',#22890,4.372);
#20203=CYLINDRICAL_SURFACE('',#22891,4.372);
#20204=CYLINDRICAL_SURFACE('',#22892,4.372);
#20205=CYLINDRICAL_SURFACE('',#22893,4.372);
#20206=CYLINDRICAL_SURFACE('',#22894,4.372);
#20207=CYLINDRICAL_SURFACE('',#22895,4.372);
#20208=CYLINDRICAL_SURFACE('',#22896,4.372);
#20209=CYLINDRICAL_SURFACE('',#22897,4.372);
#20210=CYLINDRICAL_SURFACE('',#22898,4.372);
#20211=CYLINDRICAL_SURFACE('',#22899,4.372);
#20212=CYLINDRICAL_SURFACE('',#22900,4.372);
#20213=CYLINDRICAL_SURFACE('',#22901,4.372);
#20214=CYLINDRICAL_SURFACE('',#22902,4.372);
#20215=CYLINDRICAL_SURFACE('',#22903,4.372);
#20216=CYLINDRICAL_SURFACE('',#22904,4.372);
#20217=CYLINDRICAL_SURFACE('',#22905,4.372);
#20218=CYLINDRICAL_SURFACE('',#22906,4.372);
#20219=CYLINDRICAL_SURFACE('',#22907,4.372);
#20220=CYLINDRICAL_SURFACE('',#22908,4.372);
#20221=CYLINDRICAL_SURFACE('',#22909,4.372);
#20222=CYLINDRICAL_SURFACE('',#22910,4.372);
#20223=CYLINDRICAL_SURFACE('',#22911,4.372);
#20224=CYLINDRICAL_SURFACE('',#22912,4.372);
#20225=CYLINDRICAL_SURFACE('',#22913,4.372);
#20226=CYLINDRICAL_SURFACE('',#22914,4.372);
#20227=CYLINDRICAL_SURFACE('',#22915,4.372);
#20228=CYLINDRICAL_SURFACE('',#22916,4.372);
#20229=CYLINDRICAL_SURFACE('',#22917,4.372);
#20230=CYLINDRICAL_SURFACE('',#22918,4.372);
#20231=CYLINDRICAL_SURFACE('',#22919,4.372);
#20232=CYLINDRICAL_SURFACE('',#22920,4.372);
#20233=CYLINDRICAL_SURFACE('',#22921,4.372);
#20234=CYLINDRICAL_SURFACE('',#22922,4.372);
#20235=CYLINDRICAL_SURFACE('',#22923,4.372);
#20236=CYLINDRICAL_SURFACE('',#22924,4.372);
#20237=CYLINDRICAL_SURFACE('',#22925,4.372);
#20238=CYLINDRICAL_SURFACE('',#22926,4.372);
#20239=CYLINDRICAL_SURFACE('',#22927,4.372);
#20240=CYLINDRICAL_SURFACE('',#22928,4.372);
#20241=CYLINDRICAL_SURFACE('',#22929,4.372);
#20242=CYLINDRICAL_SURFACE('',#22930,4.372);
#20243=CYLINDRICAL_SURFACE('',#22931,4.372);
#20244=CYLINDRICAL_SURFACE('',#22932,4.372);
#20245=CYLINDRICAL_SURFACE('',#22934,4.942);
#20246=CYLINDRICAL_SURFACE('',#22945,5.);
#21206=ADVANCED_FACE('',(#3086),#20124,.T.);
#21207=ADVANCED_FACE('',(#3087),#20125,.T.);
#21208=ADVANCED_FACE('',(#3088),#20126,.T.);
#21209=ADVANCED_FACE('',(#3089),#20127,.T.);
#21210=ADVANCED_FACE('',(#3090),#20128,.T.);
#21211=ADVANCED_FACE('',(#3091),#20129,.T.);
#21212=ADVANCED_FACE('',(#3092),#20130,.T.);
#21213=ADVANCED_FACE('',(#3093),#20131,.T.);
#21214=ADVANCED_FACE('',(#3094),#20132,.T.);
#21215=ADVANCED_FACE('',(#3095),#20133,.T.);
#21216=ADVANCED_FACE('',(#3096),#20134,.T.);
#21217=ADVANCED_FACE('',(#3097),#20135,.T.);
#21218=ADVANCED_FACE('',(#3098),#20136,.T.);
#21219=ADVANCED_FACE('',(#3099),#20137,.T.);
#21220=ADVANCED_FACE('',(#3100),#20138,.T.);
#21221=ADVANCED_FACE('',(#3101),#20139,.T.);
#21222=ADVANCED_FACE('',(#3102),#20140,.T.);
#21223=ADVANCED_FACE('',(#3103),#20141,.T.);
#21224=ADVANCED_FACE('',(#3104),#20142,.T.);
#21225=ADVANCED_FACE('',(#3105),#20143,.T.);
#21226=ADVANCED_FACE('',(#3106),#20144,.T.);
#21227=ADVANCED_FACE('',(#3107),#20145,.T.);
#21228=ADVANCED_FACE('',(#3108),#20146,.T.);
#21229=ADVANCED_FACE('',(#3109),#20147,.T.);
#21230=ADVANCED_FACE('',(#3110),#20148,.T.);
#21231=ADVANCED_FACE('',(#3111),#20149,.T.);
#21232=ADVANCED_FACE('',(#3112),#20150,.T.);
#21233=ADVANCED_FACE('',(#3113),#20151,.T.);
#21234=ADVANCED_FACE('',(#3114),#20152,.T.);
#21235=ADVANCED_FACE('',(#3115),#20153,.T.);
#21236=ADVANCED_FACE('',(#3116),#20154,.T.);
#21237=ADVANCED_FACE('',(#3117),#20155,.T.);
#21238=ADVANCED_FACE('',(#3118),#20156,.T.);
#21239=ADVANCED_FACE('',(#3119),#20157,.T.);
#21240=ADVANCED_FACE('',(#3120),#20158,.T.);
#21241=ADVANCED_FACE('',(#3121),#20159,.T.);
#21242=ADVANCED_FACE('',(#3122),#20160,.T.);
#21243=ADVANCED_FACE('',(#3123),#20161,.T.);
#21244=ADVANCED_FACE('',(#3124),#20162,.T.);
#21245=ADVANCED_FACE('',(#3125),#20163,.T.);
#21246=ADVANCED_FACE('',(#3126),#20164,.T.);
#21247=ADVANCED_FACE('',(#3127),#20165,.T.);
#21248=ADVANCED_FACE('',(#3128),#20166,.T.);
#21249=ADVANCED_FACE('',(#3129),#20167,.T.);
#21250=ADVANCED_FACE('',(#3130),#20168,.T.);
#21251=ADVANCED_FACE('',(#3131),#20169,.T.);
#21252=ADVANCED_FACE('',(#3132),#20170,.T.);
#21253=ADVANCED_FACE('',(#3133),#20171,.T.);
#21254=ADVANCED_FACE('',(#3134),#20172,.T.);
#21255=ADVANCED_FACE('',(#3135),#20173,.T.);
#21256=ADVANCED_FACE('',(#3136),#20174,.T.);
#21257=ADVANCED_FACE('',(#3137),#20175,.T.);
#21258=ADVANCED_FACE('',(#3138),#20176,.T.);
#21259=ADVANCED_FACE('',(#3139),#20177,.T.);
#21260=ADVANCED_FACE('',(#3140),#20178,.T.);
#21261=ADVANCED_FACE('',(#3141),#20179,.T.);
#21262=ADVANCED_FACE('',(#3142),#20180,.T.);
#21263=ADVANCED_FACE('',(#3143),#20181,.T.);
#21264=ADVANCED_FACE('',(#3144),#20182,.T.);
#21265=ADVANCED_FACE('',(#3145),#20183,.T.);
#21266=ADVANCED_FACE('',(#3146),#20184,.T.);
#21267=ADVANCED_FACE('',(#3147),#20185,.T.);
#21268=ADVANCED_FACE('',(#3148),#20186,.T.);
#21269=ADVANCED_FACE('',(#3149),#20187,.T.);
#21270=ADVANCED_FACE('',(#3150),#20188,.T.);
#21271=ADVANCED_FACE('',(#3151),#20189,.T.);
#21272=ADVANCED_FACE('',(#3152),#20190,.T.);
#21273=ADVANCED_FACE('',(#3153),#20191,.T.);
#21274=ADVANCED_FACE('',(#3154),#20192,.T.);
#21275=ADVANCED_FACE('',(#3155),#20193,.T.);
#21276=ADVANCED_FACE('',(#3156),#20194,.T.);
#21277=ADVANCED_FACE('',(#3157),#20195,.T.);
#21278=ADVANCED_FACE('',(#3158),#20196,.T.);
#21279=ADVANCED_FACE('',(#3159),#20197,.T.);
#21280=ADVANCED_FACE('',(#3160),#20198,.T.);
#21281=ADVANCED_FACE('',(#3161),#20199,.T.);
#21282=ADVANCED_FACE('',(#3162),#20200,.T.);
#21283=ADVANCED_FACE('',(#3163),#20201,.T.);
#21284=ADVANCED_FACE('',(#3164),#20202,.T.);
#21285=ADVANCED_FACE('',(#3165),#20203,.T.);
#21286=ADVANCED_FACE('',(#3166),#20204,.T.);
#21287=ADVANCED_FACE('',(#3167),#20205,.T.);
#21288=ADVANCED_FACE('',(#3168),#20206,.T.);
#21289=ADVANCED_FACE('',(#3169),#20207,.T.);
#21290=ADVANCED_FACE('',(#3170),#20208,.T.);
#21291=ADVANCED_FACE('',(#3171),#20209,.T.);
#21292=ADVANCED_FACE('',(#3172),#20210,.T.);
#21293=ADVANCED_FACE('',(#3173),#20211,.T.);
#21294=ADVANCED_FACE('',(#3174),#20212,.T.);
#21295=ADVANCED_FACE('',(#3175),#20213,.T.);
#21296=ADVANCED_FACE('',(#3176),#20214,.T.);
#21297=ADVANCED_FACE('',(#3177),#20215,.T.);
#21298=ADVANCED_FACE('',(#3178),#20216,.T.);
#21299=ADVANCED_FACE('',(#3179),#20217,.T.);
#21300=ADVANCED_FACE('',(#3180),#20218,.T.);
#21301=ADVANCED_FACE('',(#3181),#20219,.T.);
#21302=ADVANCED_FACE('',(#3182),#20220,.T.);
#21303=ADVANCED_FACE('',(#3183),#20221,.T.);
#21304=ADVANCED_FACE('',(#3184),#20222,.T.);
#21305=ADVANCED_FACE('',(#3185),#20223,.T.);
#21306=ADVANCED_FACE('',(#3186),#20224,.T.);
#21307=ADVANCED_FACE('',(#3187),#20225,.T.);
#21308=ADVANCED_FACE('',(#3188),#20226,.T.);
#21309=ADVANCED_FACE('',(#3189),#20227,.T.);
#21310=ADVANCED_FACE('',(#3190),#20228,.T.);
#21311=ADVANCED_FACE('',(#3191),#20229,.T.);
#21312=ADVANCED_FACE('',(#3192),#20230,.T.);
#21313=ADVANCED_FACE('',(#3193),#20231,.T.);
#21314=ADVANCED_FACE('',(#3194),#20232,.T.);
#21315=ADVANCED_FACE('',(#3195),#20233,.T.);
#21316=ADVANCED_FACE('',(#3196),#20234,.T.);
#21317=ADVANCED_FACE('',(#3197),#20235,.T.);
#21318=ADVANCED_FACE('',(#3198),#20236,.T.);
#21319=ADVANCED_FACE('',(#3199),#20237,.T.);
#21320=ADVANCED_FACE('',(#3200),#20238,.T.);
#21321=ADVANCED_FACE('',(#3201),#20239,.T.);
#21322=ADVANCED_FACE('',(#3202),#20240,.T.);
#21323=ADVANCED_FACE('',(#3203),#20241,.T.);
#21324=ADVANCED_FACE('',(#3204),#20242,.T.);
#21325=ADVANCED_FACE('',(#3205),#20243,.T.);
#21326=ADVANCED_FACE('',(#3206),#356,.F.);
#21327=ADVANCED_FACE('',(#3207),#20244,.T.);
#21328=ADVANCED_FACE('',(#3208),#357,.F.);
#21329=ADVANCED_FACE('',(#3209),#20245,.T.);
#21330=ADVANCED_FACE('',(#3210,#2353),#2488,.T.);
#21331=ADVANCED_FACE('',(#3211,#2354),#2489,.F.);
#21332=ADVANCED_FACE('',(#3212),#2490,.T.);
#21333=ADVANCED_FACE('',(#3213),#2491,.T.);
#21334=ADVANCED_FACE('',(#3214),#2492,.T.);
#21335=ADVANCED_FACE('',(#3215),#2493,.T.);
#21336=ADVANCED_FACE('',(#3216),#2494,.T.);
#21337=ADVANCED_FACE('',(#3217),#2495,.T.);
#21338=ADVANCED_FACE('',(#3218),#20246,.T.);
#21339=ADVANCED_FACE('',(#3219),#2496,.T.);
#21340=ADVANCED_FACE('',(#3220),#13,.T.);
#21822=CLOSED_SHELL('',(#21206,#21207,#21208,#21209,#21210,#21211,#21212,
#21213,#21214,#21215,#21216,#21217,#21218,#21219,#21220,#21221,#21222,#21223,
#21224,#21225,#21226,#21227,#21228,#21229,#21230,#21231,#21232,#21233,#21234,
#21235,#21236,#21237,#21238,#21239,#21240,#21241,#21242,#21243,#21244,#21245,
#21246,#21247,#21248,#21249,#21250,#21251,#21252,#21253,#21254,#21255,#21256,
#21257,#21258,#21259,#21260,#21261,#21262,#21263,#21264,#21265,#21266,#21267,
#21268,#21269,#21270,#21271,#21272,#21273,#21274,#21275,#21276,#21277,#21278,
#21279,#21280,#21281,#21282,#21283,#21284,#21285,#21286,#21287,#21288,#21289,
#21290,#21291,#21292,#21293,#21294,#21295,#21296,#21297,#21298,#21299,#21300,
#21301,#21302,#21303,#21304,#21305,#21306,#21307,#21308,#21309,#21310,#21311,
#21312,#21313,#21314,#21315,#21316,#21317,#21318,#21319,#21320,#21321,#21322,
#21323,#21324,#21325,#21326,#21327,#21328,#21329,#21330,#21331,#21332,#21333,
#21334,#21335,#21336,#21337,#21338,#21339,#21340));
#22809=AXIS2_PLACEMENT_3D('',#60844,#25655,#25656);
#22810=AXIS2_PLACEMENT_3D('',#60845,#25657,#25658);
#22811=AXIS2_PLACEMENT_3D('',#60861,#25660,#25661);
#22812=AXIS2_PLACEMENT_3D('',#60872,#25662,#25663);
#22813=AXIS2_PLACEMENT_3D('',#60920,#25665,#25666);
#22814=AXIS2_PLACEMENT_3D('',#60968,#25668,#25669);
#22815=AXIS2_PLACEMENT_3D('',#61019,#25671,#25672);
#22816=AXIS2_PLACEMENT_3D('',#61067,#25674,#25675);
#22817=AXIS2_PLACEMENT_3D('',#61115,#25677,#25678);
#22818=AXIS2_PLACEMENT_3D('',#61163,#25680,#25681);
#22819=AXIS2_PLACEMENT_3D('',#61217,#25683,#25684);
#22820=AXIS2_PLACEMENT_3D('',#61265,#25686,#25687);
#22821=AXIS2_PLACEMENT_3D('',#61313,#25689,#25690);
#22822=AXIS2_PLACEMENT_3D('',#61367,#25692,#25693);
#22823=AXIS2_PLACEMENT_3D('',#61415,#25695,#25696);
#22824=AXIS2_PLACEMENT_3D('',#61463,#25698,#25699);
#22825=AXIS2_PLACEMENT_3D('',#61514,#25701,#25702);
#22826=AXIS2_PLACEMENT_3D('',#61565,#25704,#25705);
#22827=AXIS2_PLACEMENT_3D('',#61613,#25707,#25708);
#22828=AXIS2_PLACEMENT_3D('',#61661,#25710,#25711);
#22829=AXIS2_PLACEMENT_3D('',#61715,#25713,#25714);
#22830=AXIS2_PLACEMENT_3D('',#61763,#25716,#25717);
#22831=AXIS2_PLACEMENT_3D('',#61811,#25719,#25720);
#22832=AXIS2_PLACEMENT_3D('',#61865,#25722,#25723);
#22833=AXIS2_PLACEMENT_3D('',#61913,#25725,#25726);
#22834=AXIS2_PLACEMENT_3D('',#61961,#25728,#25729);
#22835=AXIS2_PLACEMENT_3D('',#62009,#25731,#25732);
#22836=AXIS2_PLACEMENT_3D('',#62063,#25734,#25735);
#22837=AXIS2_PLACEMENT_3D('',#62111,#25737,#25738);
#22838=AXIS2_PLACEMENT_3D('',#62159,#25740,#25741);
#22839=AXIS2_PLACEMENT_3D('',#62213,#25743,#25744);
#22840=AXIS2_PLACEMENT_3D('',#62261,#25746,#25747);
#22841=AXIS2_PLACEMENT_3D('',#62309,#25749,#25750);
#22842=AXIS2_PLACEMENT_3D('',#62363,#25752,#25753);
#22843=AXIS2_PLACEMENT_3D('',#62411,#25755,#25756);
#22844=AXIS2_PLACEMENT_3D('',#62459,#25758,#25759);
#22845=AXIS2_PLACEMENT_3D('',#62507,#25761,#25762);
#22846=AXIS2_PLACEMENT_3D('',#62561,#25764,#25765);
#22847=AXIS2_PLACEMENT_3D('',#62609,#25767,#25768);
#22848=AXIS2_PLACEMENT_3D('',#62657,#25770,#25771);
#22849=AXIS2_PLACEMENT_3D('',#62711,#25773,#25774);
#22850=AXIS2_PLACEMENT_3D('',#62759,#25776,#25777);
#22851=AXIS2_PLACEMENT_3D('',#62807,#25779,#25780);
#22852=AXIS2_PLACEMENT_3D('',#62861,#25782,#25783);
#22853=AXIS2_PLACEMENT_3D('',#62909,#25785,#25786);
#22854=AXIS2_PLACEMENT_3D('',#62957,#25788,#25789);
#22855=AXIS2_PLACEMENT_3D('',#63005,#25791,#25792);
#22856=AXIS2_PLACEMENT_3D('',#63059,#25794,#25795);
#22857=AXIS2_PLACEMENT_3D('',#63107,#25797,#25798);
#22858=AXIS2_PLACEMENT_3D('',#63155,#25800,#25801);
#22859=AXIS2_PLACEMENT_3D('',#63209,#25803,#25804);
#22860=AXIS2_PLACEMENT_3D('',#63257,#25806,#25807);
#22861=AXIS2_PLACEMENT_3D('',#63305,#25809,#25810);
#22862=AXIS2_PLACEMENT_3D('',#63359,#25812,#25813);
#22863=AXIS2_PLACEMENT_3D('',#63407,#25815,#25816);
#22864=AXIS2_PLACEMENT_3D('',#63455,#25818,#25819);
#22865=AXIS2_PLACEMENT_3D('',#63503,#25821,#25822);
#22866=AXIS2_PLACEMENT_3D('',#63557,#25824,#25825);
#22867=AXIS2_PLACEMENT_3D('',#63605,#25827,#25828);
#22868=AXIS2_PLACEMENT_3D('',#63653,#25830,#25831);
#22869=AXIS2_PLACEMENT_3D('',#63707,#25833,#25834);
#22870=AXIS2_PLACEMENT_3D('',#63755,#25836,#25837);
#22871=AXIS2_PLACEMENT_3D('',#63803,#25839,#25840);
#22872=AXIS2_PLACEMENT_3D('',#63815,#25842,#25843);
#22873=AXIS2_PLACEMENT_3D('',#63821,#25844,#25845);
#22874=AXIS2_PLACEMENT_3D('',#63846,#25847,#25848);
#22875=AXIS2_PLACEMENT_3D('',#63870,#25850,#25851);
#22876=AXIS2_PLACEMENT_3D('',#63895,#25853,#25854);
#22877=AXIS2_PLACEMENT_3D('',#63920,#25856,#25857);
#22878=AXIS2_PLACEMENT_3D('',#63944,#25859,#25860);
#22879=AXIS2_PLACEMENT_3D('',#63969,#25862,#25863);
#22880=AXIS2_PLACEMENT_3D('',#63994,#25865,#25866);
#22881=AXIS2_PLACEMENT_3D('',#64018,#25868,#25869);
#22882=AXIS2_PLACEMENT_3D('',#64042,#25871,#25872);
#22883=AXIS2_PLACEMENT_3D('',#64067,#25874,#25875);
#22884=AXIS2_PLACEMENT_3D('',#64092,#25877,#25878);
#22885=AXIS2_PLACEMENT_3D('',#64116,#25880,#25881);
#22886=AXIS2_PLACEMENT_3D('',#64141,#25883,#25884);
#22887=AXIS2_PLACEMENT_3D('',#64166,#25886,#25887);
#22888=AXIS2_PLACEMENT_3D('',#64190,#25889,#25890);
#22889=AXIS2_PLACEMENT_3D('',#64215,#25892,#25893);
#22890=AXIS2_PLACEMENT_3D('',#64240,#25895,#25896);
#22891=AXIS2_PLACEMENT_3D('',#64264,#25898,#25899);
#22892=AXIS2_PLACEMENT_3D('',#64288,#25901,#25902);
#22893=AXIS2_PLACEMENT_3D('',#64313,#25904,#25905);
#22894=AXIS2_PLACEMENT_3D('',#64338,#25907,#25908);
#22895=AXIS2_PLACEMENT_3D('',#64362,#25910,#25911);
#22896=AXIS2_PLACEMENT_3D('',#64387,#25913,#25914);
#22897=AXIS2_PLACEMENT_3D('',#64412,#25916,#25917);
#22898=AXIS2_PLACEMENT_3D('',#64436,#25919,#25920);
#22899=AXIS2_PLACEMENT_3D('',#64461,#25922,#25923);
#22900=AXIS2_PLACEMENT_3D('',#64486,#25925,#25926);
#22901=AXIS2_PLACEMENT_3D('',#64510,#25928,#25929);
#22902=AXIS2_PLACEMENT_3D('',#64534,#25931,#25932);
#22903=AXIS2_PLACEMENT_3D('',#64559,#25934,#25935);
#22904=AXIS2_PLACEMENT_3D('',#64584,#25937,#25938);
#22905=AXIS2_PLACEMENT_3D('',#64608,#25940,#25941);
#22906=AXIS2_PLACEMENT_3D('',#64633,#25943,#25944);
#22907=AXIS2_PLACEMENT_3D('',#64658,#25946,#25947);
#22908=AXIS2_PLACEMENT_3D('',#64682,#25949,#25950);
#22909=AXIS2_PLACEMENT_3D('',#64707,#25952,#25953);
#22910=AXIS2_PLACEMENT_3D('',#64732,#25955,#25956);
#22911=AXIS2_PLACEMENT_3D('',#64756,#25958,#25959);
#22912=AXIS2_PLACEMENT_3D('',#64780,#25961,#25962);
#22913=AXIS2_PLACEMENT_3D('',#64805,#25964,#25965);
#22914=AXIS2_PLACEMENT_3D('',#64830,#25967,#25968);
#22915=AXIS2_PLACEMENT_3D('',#64854,#25970,#25971);
#22916=AXIS2_PLACEMENT_3D('',#64879,#25973,#25974);
#22917=AXIS2_PLACEMENT_3D('',#64904,#25976,#25977);
#22918=AXIS2_PLACEMENT_3D('',#64928,#25979,#25980);
#22919=AXIS2_PLACEMENT_3D('',#64953,#25982,#25983);
#22920=AXIS2_PLACEMENT_3D('',#64977,#25985,#25986);
#22921=AXIS2_PLACEMENT_3D('',#65002,#25988,#25989);
#22922=AXIS2_PLACEMENT_3D('',#65026,#25991,#25992);
#22923=AXIS2_PLACEMENT_3D('',#65051,#25994,#25995);
#22924=AXIS2_PLACEMENT_3D('',#65076,#25997,#25998);
#22925=AXIS2_PLACEMENT_3D('',#65100,#26000,#26001);
#22926=AXIS2_PLACEMENT_3D('',#65125,#26003,#26004);
#22927=AXIS2_PLACEMENT_3D('',#65150,#26006,#26007);
#22928=AXIS2_PLACEMENT_3D('',#65174,#26009,#26010);
#22929=AXIS2_PLACEMENT_3D('',#65199,#26012,#26013);
#22930=AXIS2_PLACEMENT_3D('',#65223,#26015,#26016);
#22931=AXIS2_PLACEMENT_3D('',#65248,#26018,#26019);
#22932=AXIS2_PLACEMENT_3D('',#67057,#26021,#26022);
#22933=AXIS2_PLACEMENT_3D('',#67059,#26023,#26024);
#22934=AXIS2_PLACEMENT_3D('',#68841,#26025,#26026);
#22935=AXIS2_PLACEMENT_3D('',#68842,#26027,#26028);
#22936=AXIS2_PLACEMENT_3D('',#68843,#26029,#26030);
#22937=AXIS2_PLACEMENT_3D('',#68856,#26037,#26038);
#22938=AXIS2_PLACEMENT_3D('',#68870,#26045,#26046);
#22939=AXIS2_PLACEMENT_3D('',#68871,#26047,#26048);
#22940=AXIS2_PLACEMENT_3D('',#68874,#26051,#26052);
#22941=AXIS2_PLACEMENT_3D('',#68876,#26054,#26055);
#22942=AXIS2_PLACEMENT_3D('',#68878,#26057,#26058);
#22943=AXIS2_PLACEMENT_3D('',#68880,#26060,#26061);
#22944=AXIS2_PLACEMENT_3D('',#68882,#26063,#26064);
#22945=AXIS2_PLACEMENT_3D('',#68883,#26065,#26066);
#22946=AXIS2_PLACEMENT_3D('',#68886,#26068,#26069);
#22947=AXIS2_PLACEMENT_3D('',#68887,#26070,#26071);
#22948=AXIS2_PLACEMENT_3D('',#68888,#26072,#26073);
#22949=AXIS2_PLACEMENT_3D('',#68890,#26074,#26075);
#25655=DIRECTION('axis',(0.,0.,1.));
#25656=DIRECTION('refdir',(1.,0.,0.));
#25657=DIRECTION('center_axis',(0.,0.,1.));
#25658=DIRECTION('ref_axis',(1.,0.,0.));
#25659=DIRECTION('',(0.,0.,-1.));
#25660=DIRECTION('center_axis',(0.,0.,-1.));
#25661=DIRECTION('ref_axis',(1.,0.,0.));
#25662=DIRECTION('center_axis',(0.,0.,1.));
#25663=DIRECTION('ref_axis',(1.,0.,0.));
#25664=DIRECTION('',(0.,0.,-1.));
#25665=DIRECTION('center_axis',(0.,0.,1.));
#25666=DIRECTION('ref_axis',(1.,0.,0.));
#25667=DIRECTION('',(0.,0.,-1.));
#25668=DIRECTION('center_axis',(0.,0.,1.));
#25669=DIRECTION('ref_axis',(1.,0.,0.));
#25670=DIRECTION('',(0.,0.,-1.));
#25671=DIRECTION('center_axis',(0.,0.,1.));
#25672=DIRECTION('ref_axis',(1.,0.,0.));
#25673=DIRECTION('',(0.,0.,-1.));
#25674=DIRECTION('center_axis',(0.,0.,1.));
#25675=DIRECTION('ref_axis',(1.,0.,0.));
#25676=DIRECTION('',(0.,0.,-1.));
#25677=DIRECTION('center_axis',(0.,0.,1.));
#25678=DIRECTION('ref_axis',(1.,0.,0.));
#25679=DIRECTION('',(0.,0.,-1.));
#25680=DIRECTION('center_axis',(0.,0.,1.));
#25681=DIRECTION('ref_axis',(1.,0.,0.));
#25682=DIRECTION('',(0.,0.,-1.));
#25683=DIRECTION('center_axis',(0.,0.,1.));
#25684=DIRECTION('ref_axis',(1.,0.,0.));
#25685=DIRECTION('',(0.,0.,-1.));
#25686=DIRECTION('center_axis',(0.,0.,1.));
#25687=DIRECTION('ref_axis',(1.,0.,0.));
#25688=DIRECTION('',(0.,0.,-1.));
#25689=DIRECTION('center_axis',(0.,0.,1.));
#25690=DIRECTION('ref_axis',(1.,0.,0.));
#25691=DIRECTION('',(0.,0.,-1.));
#25692=DIRECTION('center_axis',(0.,0.,1.));
#25693=DIRECTION('ref_axis',(1.,0.,0.));
#25694=DIRECTION('',(0.,0.,-1.));
#25695=DIRECTION('center_axis',(0.,0.,1.));
#25696=DIRECTION('ref_axis',(1.,0.,0.));
#25697=DIRECTION('',(0.,0.,-1.));
#25698=DIRECTION('center_axis',(0.,0.,1.));
#25699=DIRECTION('ref_axis',(1.,0.,0.));
#25700=DIRECTION('',(0.,0.,-1.));
#25701=DIRECTION('center_axis',(0.,0.,1.));
#25702=DIRECTION('ref_axis',(1.,0.,0.));
#25703=DIRECTION('',(0.,0.,-1.));
#25704=DIRECTION('center_axis',(0.,0.,1.));
#25705=DIRECTION('ref_axis',(1.,0.,0.));
#25706=DIRECTION('',(0.,0.,-1.));
#25707=DIRECTION('center_axis',(0.,0.,1.));
#25708=DIRECTION('ref_axis',(1.,0.,0.));
#25709=DIRECTION('',(0.,0.,-1.));
#25710=DIRECTION('center_axis',(0.,0.,1.));
#25711=DIRECTION('ref_axis',(1.,0.,0.));
#25712=DIRECTION('',(0.,0.,-1.));
#25713=DIRECTION('center_axis',(0.,0.,1.));
#25714=DIRECTION('ref_axis',(1.,0.,0.));
#25715=DIRECTION('',(0.,0.,-1.));
#25716=DIRECTION('center_axis',(0.,0.,1.));
#25717=DIRECTION('ref_axis',(1.,0.,0.));
#25718=DIRECTION('',(0.,0.,-1.));
#25719=DIRECTION('center_axis',(0.,0.,1.));
#25720=DIRECTION('ref_axis',(1.,0.,0.));
#25721=DIRECTION('',(0.,0.,-1.));
#25722=DIRECTION('center_axis',(0.,0.,1.));
#25723=DIRECTION('ref_axis',(1.,0.,0.));
#25724=DIRECTION('',(0.,0.,-1.));
#25725=DIRECTION('center_axis',(0.,0.,1.));
#25726=DIRECTION('ref_axis',(1.,0.,0.));
#25727=DIRECTION('',(0.,0.,-1.));
#25728=DIRECTION('center_axis',(0.,0.,1.));
#25729=DIRECTION('ref_axis',(1.,0.,0.));
#25730=DIRECTION('',(0.,0.,-1.));
#25731=DIRECTION('center_axis',(0.,0.,1.));
#25732=DIRECTION('ref_axis',(1.,0.,0.));
#25733=DIRECTION('',(0.,0.,-1.));
#25734=DIRECTION('center_axis',(0.,0.,1.));
#25735=DIRECTION('ref_axis',(1.,0.,0.));
#25736=DIRECTION('',(0.,0.,-1.));
#25737=DIRECTION('center_axis',(0.,0.,1.));
#25738=DIRECTION('ref_axis',(1.,0.,0.));
#25739=DIRECTION('',(0.,0.,-1.));
#25740=DIRECTION('center_axis',(0.,0.,1.));
#25741=DIRECTION('ref_axis',(1.,0.,0.));
#25742=DIRECTION('',(0.,0.,-1.));
#25743=DIRECTION('center_axis',(0.,0.,1.));
#25744=DIRECTION('ref_axis',(1.,0.,0.));
#25745=DIRECTION('',(0.,0.,-1.));
#25746=DIRECTION('center_axis',(0.,0.,1.));
#25747=DIRECTION('ref_axis',(1.,0.,0.));
#25748=DIRECTION('',(0.,0.,-1.));
#25749=DIRECTION('center_axis',(0.,0.,1.));
#25750=DIRECTION('ref_axis',(1.,0.,0.));
#25751=DIRECTION('',(0.,0.,-1.));
#25752=DIRECTION('center_axis',(0.,0.,1.));
#25753=DIRECTION('ref_axis',(1.,0.,0.));
#25754=DIRECTION('',(0.,0.,-1.));
#25755=DIRECTION('center_axis',(0.,0.,1.));
#25756=DIRECTION('ref_axis',(1.,0.,0.));
#25757=DIRECTION('',(0.,0.,-1.));
#25758=DIRECTION('center_axis',(0.,0.,1.));
#25759=DIRECTION('ref_axis',(1.,0.,0.));
#25760=DIRECTION('',(0.,0.,-1.));
#25761=DIRECTION('center_axis',(0.,0.,1.));
#25762=DIRECTION('ref_axis',(1.,0.,0.));
#25763=DIRECTION('',(0.,0.,-1.));
#25764=DIRECTION('center_axis',(0.,0.,1.));
#25765=DIRECTION('ref_axis',(1.,0.,0.));
#25766=DIRECTION('',(0.,0.,-1.));
#25767=DIRECTION('center_axis',(0.,0.,1.));
#25768=DIRECTION('ref_axis',(1.,0.,0.));
#25769=DIRECTION('',(0.,0.,-1.));
#25770=DIRECTION('center_axis',(0.,0.,1.));
#25771=DIRECTION('ref_axis',(1.,0.,0.));
#25772=DIRECTION('',(0.,0.,-1.));
#25773=DIRECTION('center_axis',(0.,0.,1.));
#25774=DIRECTION('ref_axis',(1.,0.,0.));
#25775=DIRECTION('',(0.,0.,-1.));
#25776=DIRECTION('center_axis',(0.,0.,1.));
#25777=DIRECTION('ref_axis',(1.,0.,0.));
#25778=DIRECTION('',(0.,0.,-1.));
#25779=DIRECTION('center_axis',(0.,0.,1.));
#25780=DIRECTION('ref_axis',(1.,0.,0.));
#25781=DIRECTION('',(0.,0.,-1.));
#25782=DIRECTION('center_axis',(0.,0.,1.));
#25783=DIRECTION('ref_axis',(1.,0.,0.));
#25784=DIRECTION('',(0.,0.,-1.));
#25785=DIRECTION('center_axis',(0.,0.,1.));
#25786=DIRECTION('ref_axis',(1.,0.,0.));
#25787=DIRECTION('',(0.,0.,-1.));
#25788=DIRECTION('center_axis',(0.,0.,1.));
#25789=DIRECTION('ref_axis',(1.,0.,0.));
#25790=DIRECTION('',(0.,0.,-1.));
#25791=DIRECTION('center_axis',(0.,0.,1.));
#25792=DIRECTION('ref_axis',(1.,0.,0.));
#25793=DIRECTION('',(0.,0.,-1.));
#25794=DIRECTION('center_axis',(0.,0.,1.));
#25795=DIRECTION('ref_axis',(1.,0.,0.));
#25796=DIRECTION('',(0.,0.,-1.));
#25797=DIRECTION('center_axis',(0.,0.,1.));
#25798=DIRECTION('ref_axis',(1.,0.,0.));
#25799=DIRECTION('',(0.,0.,-1.));
#25800=DIRECTION('center_axis',(0.,0.,1.));
#25801=DIRECTION('ref_axis',(1.,0.,0.));
#25802=DIRECTION('',(0.,0.,-1.));
#25803=DIRECTION('center_axis',(0.,0.,1.));
#25804=DIRECTION('ref_axis',(1.,0.,0.));
#25805=DIRECTION('',(0.,0.,-1.));
#25806=DIRECTION('center_axis',(0.,0.,1.));
#25807=DIRECTION('ref_axis',(1.,0.,0.));
#25808=DIRECTION('',(0.,0.,-1.));
#25809=DIRECTION('center_axis',(0.,0.,1.));
#25810=DIRECTION('ref_axis',(1.,0.,0.));
#25811=DIRECTION('',(0.,0.,-1.));
#25812=DIRECTION('center_axis',(0.,0.,1.));
#25813=DIRECTION('ref_axis',(1.,0.,0.));
#25814=DIRECTION('',(0.,0.,-1.));
#25815=DIRECTION('center_axis',(0.,0.,1.));
#25816=DIRECTION('ref_axis',(1.,0.,0.));
#25817=DIRECTION('',(0.,0.,-1.));
#25818=DIRECTION('center_axis',(0.,0.,1.));
#25819=DIRECTION('ref_axis',(1.,0.,0.));
#25820=DIRECTION('',(0.,0.,-1.));
#25821=DIRECTION('center_axis',(0.,0.,1.));
#25822=DIRECTION('ref_axis',(1.,0.,0.));
#25823=DIRECTION('',(0.,0.,-1.));
#25824=DIRECTION('center_axis',(0.,0.,1.));
#25825=DIRECTION('ref_axis',(1.,0.,0.));
#25826=DIRECTION('',(0.,0.,-1.));
#25827=DIRECTION('center_axis',(0.,0.,1.));
#25828=DIRECTION('ref_axis',(1.,0.,0.));
#25829=DIRECTION('',(0.,0.,-1.));
#25830=DIRECTION('center_axis',(0.,0.,1.));
#25831=DIRECTION('ref_axis',(1.,0.,0.));
#25832=DIRECTION('',(0.,0.,-1.));
#25833=DIRECTION('center_axis',(0.,0.,1.));
#25834=DIRECTION('ref_axis',(1.,0.,0.));
#25835=DIRECTION('',(0.,0.,-1.));
#25836=DIRECTION('center_axis',(0.,0.,1.));
#25837=DIRECTION('ref_axis',(1.,0.,0.));
#25838=DIRECTION('',(0.,0.,-1.));
#25839=DIRECTION('center_axis',(0.,0.,1.));
#25840=DIRECTION('ref_axis',(-0.457630590434842,-0.889142419805881,0.));
#25841=DIRECTION('',(0.,0.,1.));
#25842=DIRECTION('center_axis',(0.,0.,1.));
#25843=DIRECTION('ref_axis',(1.,-8.75189148499889E-13,0.));
#25844=DIRECTION('center_axis',(0.,0.,1.));
#25845=DIRECTION('ref_axis',(1.,-8.75189148499889E-13,0.));
#25846=DIRECTION('',(0.,0.,1.));
#25847=DIRECTION('center_axis',(0.,0.,1.));
#25848=DIRECTION('ref_axis',(1.,-8.75189148499889E-13,0.));
#25849=DIRECTION('',(0.,0.,1.));
#25850=DIRECTION('center_axis',(0.,0.,1.));
#25851=DIRECTION('ref_axis',(1.,-8.75189148499889E-13,0.));
#25852=DIRECTION('',(0.,0.,1.));
#25853=DIRECTION('center_axis',(0.,0.,1.));
#25854=DIRECTION('ref_axis',(1.,-8.75189148499889E-13,0.));
#25855=DIRECTION('',(0.,0.,1.));
#25856=DIRECTION('center_axis',(0.,0.,1.));
#25857=DIRECTION('ref_axis',(1.,-8.75189148499889E-13,0.));
#25858=DIRECTION('',(0.,0.,1.));
#25859=DIRECTION('center_axis',(0.,0.,1.));
#25860=DIRECTION('ref_axis',(1.,-8.75189148499889E-13,0.));
#25861=DIRECTION('',(0.,0.,1.));
#25862=DIRECTION('center_axis',(0.,0.,1.));
#25863=DIRECTION('ref_axis',(1.,-8.75189148499889E-13,0.));
#25864=DIRECTION('',(0.,0.,1.));
#25865=DIRECTION('center_axis',(0.,0.,1.));
#25866=DIRECTION('ref_axis',(1.,-8.75189148499889E-13,0.));
#25867=DIRECTION('',(0.,0.,1.));
#25868=DIRECTION('center_axis',(0.,0.,1.));
#25869=DIRECTION('ref_axis',(1.,-8.75189148499889E-13,0.));
#25870=DIRECTION('',(0.,0.,1.));
#25871=DIRECTION('center_axis',(0.,0.,1.));
#25872=DIRECTION('ref_axis',(1.,-8.75189148499889E-13,0.));
#25873=DIRECTION('',(0.,0.,1.));
#25874=DIRECTION('center_axis',(0.,0.,1.));
#25875=DIRECTION('ref_axis',(1.,-8.75189148499889E-13,0.));
#25876=DIRECTION('',(0.,0.,1.));
#25877=DIRECTION('center_axis',(0.,0.,1.));
#25878=DIRECTION('ref_axis',(1.,-8.75189148499889E-13,0.));
#25879=DIRECTION('',(0.,0.,1.));
#25880=DIRECTION('center_axis',(0.,0.,1.));
#25881=DIRECTION('ref_axis',(1.,-8.75189148499889E-13,0.));
#25882=DIRECTION('',(0.,0.,1.));
#25883=DIRECTION('center_axis',(0.,0.,1.));
#25884=DIRECTION('ref_axis',(1.,-8.75189148499889E-13,0.));
#25885=DIRECTION('',(0.,0.,1.));
#25886=DIRECTION('center_axis',(0.,0.,1.));
#25887=DIRECTION('ref_axis',(1.,-8.75189148499889E-13,0.));
#25888=DIRECTION('',(0.,0.,1.));
#25889=DIRECTION('center_axis',(0.,0.,1.));
#25890=DIRECTION('ref_axis',(1.,-8.75189148499889E-13,0.));
#25891=DIRECTION('',(0.,0.,1.));
#25892=DIRECTION('center_axis',(0.,0.,1.));
#25893=DIRECTION('ref_axis',(1.,-8.75189148499889E-13,0.));
#25894=DIRECTION('',(0.,0.,1.));
#25895=DIRECTION('center_axis',(0.,0.,1.));
#25896=DIRECTION('ref_axis',(1.,-8.75189148499889E-13,0.));
#25897=DIRECTION('',(0.,0.,1.));
#25898=DIRECTION('center_axis',(0.,0.,1.));
#25899=DIRECTION('ref_axis',(1.,-8.75189148499889E-13,0.));
#25900=DIRECTION('',(0.,0.,1.));
#25901=DIRECTION('center_axis',(0.,0.,1.));
#25902=DIRECTION('ref_axis',(1.,-8.75189148499889E-13,0.));
#25903=DIRECTION('',(0.,0.,1.));
#25904=DIRECTION('center_axis',(0.,0.,1.));
#25905=DIRECTION('ref_axis',(1.,-8.75189148499889E-13,0.));
#25906=DIRECTION('',(0.,0.,1.));
#25907=DIRECTION('center_axis',(0.,0.,1.));
#25908=DIRECTION('ref_axis',(1.,-8.75189148499889E-13,0.));
#25909=DIRECTION('',(0.,0.,1.));
#25910=DIRECTION('center_axis',(0.,0.,1.));
#25911=DIRECTION('ref_axis',(1.,-8.75189148499889E-13,0.));
#25912=DIRECTION('',(0.,0.,1.));
#25913=DIRECTION('center_axis',(0.,0.,1.));
#25914=DIRECTION('ref_axis',(1.,-8.75189148499889E-13,0.));
#25915=DIRECTION('',(0.,0.,1.));
#25916=DIRECTION('center_axis',(0.,0.,1.));
#25917=DIRECTION('ref_axis',(1.,-8.75189148499889E-13,0.));
#25918=DIRECTION('',(0.,0.,1.));
#25919=DIRECTION('center_axis',(0.,0.,1.));
#25920=DIRECTION('ref_axis',(1.,-8.75189148499889E-13,0.));
#25921=DIRECTION('',(0.,0.,1.));
#25922=DIRECTION('center_axis',(0.,0.,1.));
#25923=DIRECTION('ref_axis',(1.,-8.75189148499889E-13,0.));
#25924=DIRECTION('',(0.,0.,1.));
#25925=DIRECTION('center_axis',(0.,0.,1.));
#25926=DIRECTION('ref_axis',(1.,-8.75189148499889E-13,0.));
#25927=DIRECTION('',(0.,0.,1.));
#25928=DIRECTION('center_axis',(0.,0.,1.));
#25929=DIRECTION('ref_axis',(1.,-8.75189148499889E-13,0.));
#25930=DIRECTION('',(0.,0.,1.));
#25931=DIRECTION('center_axis',(0.,0.,1.));
#25932=DIRECTION('ref_axis',(1.,-8.75189148499889E-13,0.));
#25933=DIRECTION('',(0.,0.,1.));
#25934=DIRECTION('center_axis',(0.,0.,1.));
#25935=DIRECTION('ref_axis',(1.,-8.75189148499889E-13,0.));
#25936=DIRECTION('',(0.,0.,1.));
#25937=DIRECTION('center_axis',(0.,0.,1.));
#25938=DIRECTION('ref_axis',(1.,-8.75189148499889E-13,0.));
#25939=DIRECTION('',(0.,0.,1.));
#25940=DIRECTION('center_axis',(0.,0.,1.));
#25941=DIRECTION('ref_axis',(1.,-8.75189148499889E-13,0.));
#25942=DIRECTION('',(0.,0.,1.));
#25943=DIRECTION('center_axis',(0.,0.,1.));
#25944=DIRECTION('ref_axis',(1.,-8.75189148499889E-13,0.));
#25945=DIRECTION('',(0.,0.,1.));
#25946=DIRECTION('center_axis',(0.,0.,1.));
#25947=DIRECTION('ref_axis',(1.,-8.75189148499889E-13,0.));
#25948=DIRECTION('',(0.,0.,1.));
#25949=DIRECTION('center_axis',(0.,0.,1.));
#25950=DIRECTION('ref_axis',(1.,-8.75189148499889E-13,0.));
#25951=DIRECTION('',(0.,0.,1.));
#25952=DIRECTION('center_axis',(0.,0.,1.));
#25953=DIRECTION('ref_axis',(1.,-8.75189148499889E-13,0.));
#25954=DIRECTION('',(0.,0.,1.));
#25955=DIRECTION('center_axis',(0.,0.,1.));
#25956=DIRECTION('ref_axis',(1.,-8.75189148499889E-13,0.));
#25957=DIRECTION('',(0.,0.,1.));
#25958=DIRECTION('center_axis',(0.,0.,1.));
#25959=DIRECTION('ref_axis',(1.,-8.75189148499889E-13,0.));
#25960=DIRECTION('',(0.,0.,1.));
#25961=DIRECTION('center_axis',(0.,0.,1.));
#25962=DIRECTION('ref_axis',(1.,-8.75189148499889E-13,0.));
#25963=DIRECTION('',(0.,0.,1.));
#25964=DIRECTION('center_axis',(0.,0.,1.));
#25965=DIRECTION('ref_axis',(1.,-8.75189148499889E-13,0.));
#25966=DIRECTION('',(0.,0.,1.));
#25967=DIRECTION('center_axis',(0.,0.,1.));
#25968=DIRECTION('ref_axis',(1.,-8.75189148499889E-13,0.));
#25969=DIRECTION('',(0.,0.,1.));
#25970=DIRECTION('center_axis',(0.,0.,1.));
#25971=DIRECTION('ref_axis',(1.,-8.75189148499889E-13,0.));
#25972=DIRECTION('',(0.,0.,1.));
#25973=DIRECTION('center_axis',(0.,0.,1.));
#25974=DIRECTION('ref_axis',(1.,-8.75189148499889E-13,0.));
#25975=DIRECTION('',(0.,0.,1.));
#25976=DIRECTION('center_axis',(0.,0.,1.));
#25977=DIRECTION('ref_axis',(1.,-8.75189148499889E-13,0.));
#25978=DIRECTION('',(0.,0.,1.));
#25979=DIRECTION('center_axis',(0.,0.,1.));
#25980=DIRECTION('ref_axis',(1.,-8.75189148499889E-13,0.));
#25981=DIRECTION('',(0.,0.,1.));
#25982=DIRECTION('center_axis',(0.,0.,1.));
#25983=DIRECTION('ref_axis',(1.,-8.75189148499889E-13,0.));
#25984=DIRECTION('',(0.,0.,1.));
#25985=DIRECTION('center_axis',(0.,0.,1.));
#25986=DIRECTION('ref_axis',(1.,-8.75189148499889E-13,0.));
#25987=DIRECTION('',(0.,0.,1.));
#25988=DIRECTION('center_axis',(0.,0.,1.));
#25989=DIRECTION('ref_axis',(1.,-8.75189148499889E-13,0.));
#25990=DIRECTION('',(0.,0.,1.));
#25991=DIRECTION('center_axis',(0.,0.,1.));
#25992=DIRECTION('ref_axis',(1.,-8.75189148499889E-13,0.));
#25993=DIRECTION('',(0.,0.,1.));
#25994=DIRECTION('center_axis',(0.,0.,1.));
#25995=DIRECTION('ref_axis',(1.,-8.75189148499889E-13,0.));
#25996=DIRECTION('',(0.,0.,1.));
#25997=DIRECTION('center_axis',(0.,0.,1.));
#25998=DIRECTION('ref_axis',(1.,-8.75189148499889E-13,0.));
#25999=DIRECTION('',(0.,0.,1.));
#26000=DIRECTION('center_axis',(0.,0.,1.));
#26001=DIRECTION('ref_axis',(1.,-8.75189148499889E-13,0.));
#26002=DIRECTION('',(0.,0.,1.));
#26003=DIRECTION('center_axis',(0.,0.,1.));
#26004=DIRECTION('ref_axis',(1.,-8.75189148499889E-13,0.));
#26005=DIRECTION('',(0.,0.,1.));
#26006=DIRECTION('center_axis',(0.,0.,1.));
#26007=DIRECTION('ref_axis',(1.,-8.75189148499889E-13,0.));
#26008=DIRECTION('',(0.,0.,1.));
#26009=DIRECTION('center_axis',(0.,0.,1.));
#26010=DIRECTION('ref_axis',(1.,-8.75189148499889E-13,0.));
#26011=DIRECTION('',(0.,0.,1.));
#26012=DIRECTION('center_axis',(0.,0.,1.));
#26013=DIRECTION('ref_axis',(1.,-8.75189148499889E-13,0.));
#26014=DIRECTION('',(0.,0.,1.));
#26015=DIRECTION('center_axis',(0.,0.,1.));
#26016=DIRECTION('ref_axis',(1.,-8.75189148499889E-13,0.));
#26017=DIRECTION('',(0.,0.,1.));
#26018=DIRECTION('center_axis',(0.,0.,1.));
#26019=DIRECTION('ref_axis',(1.,-8.75189148499889E-13,0.));
#26020=DIRECTION('',(0.,0.,1.));
#26021=DIRECTION('center_axis',(0.,0.,1.));
#26022=DIRECTION('ref_axis',(1.,-8.75189148499889E-13,0.));
#26023=DIRECTION('center_axis',(0.,0.,-1.));
#26024=DIRECTION('ref_axis',(1.,-8.75189148499889E-13,0.));
#26025=DIRECTION('center_axis',(0.,0.,1.));
#26026=DIRECTION('ref_axis',(1.,0.,0.));
#26027=DIRECTION('center_axis',(0.,0.,-1.));
#26028=DIRECTION('ref_axis',(1.,0.,0.));
#26029=DIRECTION('center_axis',(0.,0.,1.));
#26030=DIRECTION('ref_axis',(1.,0.,0.));
#26031=DIRECTION('',(0.5,0.866025403784439,0.));
#26032=DIRECTION('',(-0.5,0.866025403784439,0.));
#26033=DIRECTION('',(-1.,1.20185167898973E-16,0.));
#26034=DIRECTION('',(-0.5,-0.866025403784439,0.));
#26035=DIRECTION('',(0.5,-0.866025403784439,0.));
#26036=DIRECTION('',(1.,-2.40370335797945E-16,0.));
#26037=DIRECTION('center_axis',(0.,0.,1.));
#26038=DIRECTION('ref_axis',(1.,0.,0.));
#26039=DIRECTION('',(0.5,0.866025403784439,0.));
#26040=DIRECTION('',(1.,-2.40370335797945E-16,0.));
#26041=DIRECTION('',(0.5,-0.866025403784439,0.));
#26042=DIRECTION('',(-0.5,-0.866025403784439,0.));
#26043=DIRECTION('',(-1.,1.20185167898973E-16,0.));
#26044=DIRECTION('',(-0.5,0.866025403784439,0.));
#26045=DIRECTION('center_axis',(0.,0.,-1.));
#26046=DIRECTION('ref_axis',(1.,0.,0.));
#26047=DIRECTION('center_axis',(-2.40370335797945E-16,-1.,0.));
#26048=DIRECTION('ref_axis',(1.,-2.40370335797945E-16,0.));
#26049=DIRECTION('',(0.,0.,1.));
#26050=DIRECTION('',(0.,0.,1.));
#26051=DIRECTION('center_axis',(-0.866025403784439,-0.5,0.));
#26052=DIRECTION('ref_axis',(0.5,-0.866025403784439,0.));
#26053=DIRECTION('',(0.,0.,1.));
#26054=DIRECTION('center_axis',(-0.866025403784439,0.5,0.));
#26055=DIRECTION('ref_axis',(-0.5,-0.866025403784439,0.));
#26056=DIRECTION('',(0.,0.,1.));
#26057=DIRECTION('center_axis',(1.20185167898973E-16,1.,0.));
#26058=DIRECTION('ref_axis',(-1.,1.20185167898973E-16,0.));
#26059=DIRECTION('',(0.,0.,1.));
#26060=DIRECTION('center_axis',(0.866025403784439,0.5,0.));
#26061=DIRECTION('ref_axis',(-0.5,0.866025403784439,0.));
#26062=DIRECTION('',(0.,0.,1.));
#26063=DIRECTION('center_axis',(0.866025403784439,-0.5,0.));
#26064=DIRECTION('ref_axis',(0.5,0.866025403784439,0.));
#26065=DIRECTION('center_axis',(0.,0.,1.));
#26066=DIRECTION('ref_axis',(1.,0.,0.));
#26067=DIRECTION('',(0.,0.,-1.));
#26068=DIRECTION('center_axis',(0.,0.,-1.));
#26069=DIRECTION('ref_axis',(1.,0.,0.));
#26070=DIRECTION('center_axis',(0.,0.,1.));
#26071=DIRECTION('ref_axis',(1.,0.,0.));
#26072=DIRECTION('center_axis',(6.12323399573677E-17,0.,1.));
#26073=DIRECTION('ref_axis',(1.,0.,0.));
#26074=DIRECTION('center_axis',(1.22464679914735E-16,-1.,0.));
#26075=DIRECTION('ref_axis',(-1.,-1.22464679914735E-16,0.));
#60844=CARTESIAN_POINT('',(0.,0.,0.));
#60845=CARTESIAN_POINT('Origin',(0.,0.,16.));
#60846=CARTESIAN_POINT('',(-4.94751652564198,0.00256483971322934,26.3223204546569));
#60847=CARTESIAN_POINT('',(-4.94433041235646,0.00147179461986118,26.1776795453432));
#60848=CARTESIAN_POINT('',(-4.942,-6.05220448138622E-16,16.));
#60849=CARTESIAN_POINT('',(2.16917135428601,4.44050218283304,26.));
#60850=CARTESIAN_POINT('Ctrl Pts',(-4.94751652564198,0.00256483971322934,
26.3223204546569));
#60851=CARTESIAN_POINT('Ctrl Pts',(-4.94869886604438,0.171401137605494,
26.3168647682864));
#60852=CARTESIAN_POINT('Ctrl Pts',(-4.9408321732254,0.340133662244093,26.311409081916));
#60853=CARTESIAN_POINT('Ctrl Pts',(-4.92355817442292,0.507901950004805,
26.3059533955455));
#60854=CARTESIAN_POINT('Ctrl Pts',(-4.75600008116697,2.13525730225587,26.2530331414635));
#60855=CARTESIAN_POINT('Ctrl Pts',(-3.70330534691493,3.67188727651734,26.2001128873815));
#60856=CARTESIAN_POINT('Ctrl Pts',(-2.24451326222463,4.41286251356918,26.1471926332996));
#60857=CARTESIAN_POINT('Ctrl Pts',(-0.892016301737719,5.09984646860033,
26.0981284221997));
#60858=CARTESIAN_POINT('Ctrl Pts',(0.80955341496604,5.10290231670094,26.0490642110999));
#60859=CARTESIAN_POINT('Ctrl Pts',(2.17574200330363,4.4448669900444,26.));
#60860=CARTESIAN_POINT('',(-2.16917135428577,4.44050218283316,26.));
#60861=CARTESIAN_POINT('Origin',(0.,0.,26.));
#60862=CARTESIAN_POINT('Ctrl Pts',(-2.16917135428577,4.44050218283316,26.));
#60863=CARTESIAN_POINT('Ctrl Pts',(-2.90742207776898,4.07986902565299,26.026460127041));
#60864=CARTESIAN_POINT('Ctrl Pts',(-3.54838487149729,3.53163056089739,26.0529202540819));
#60865=CARTESIAN_POINT('Ctrl Pts',(-4.02597159025063,2.86203897562359,26.0793803811229));
#60866=CARTESIAN_POINT('Ctrl Pts',(-4.50355830900396,2.19244739034978,26.1058405081639));
#60867=CARTESIAN_POINT('Ctrl Pts',(-4.81776895278232,1.40150268455777,26.1323006352049));
#60868=CARTESIAN_POINT('Ctrl Pts',(-4.91302280979298,0.586752670320857,
26.1587607622459));
#60869=CARTESIAN_POINT('Ctrl Pts',(-4.93572472976967,0.39257271577962,26.1650670232783));
#60870=CARTESIAN_POINT('Ctrl Pts',(-4.94598956917588,0.197040583288091,
26.1713732843108));
#60871=CARTESIAN_POINT('Ctrl Pts',(-4.94433041235646,0.00147179461986118,
26.1776795453432));
#60872=CARTESIAN_POINT('Origin',(0.,0.,16.));
#60873=CARTESIAN_POINT('',(-4.93516121822955,0.00250487983550263,27.3223204546569));
#60874=CARTESIAN_POINT('',(-4.93474635697119,0.00209204260276723,27.1776795453432));
#60875=CARTESIAN_POINT('',(-4.942,-6.05220448138622E-16,16.));
#60876=CARTESIAN_POINT('Ctrl Pts',(-4.93516121822955,0.00250487983550263,
27.3223204546569));
#60877=CARTESIAN_POINT('Ctrl Pts',(-4.93820686879495,0.665010559781625,
27.3010529594449));
#60878=CARTESIAN_POINT('Ctrl Pts',(-4.81416865933799,1.32642295622759,27.2797854642328));
#60879=CARTESIAN_POINT('Ctrl Pts',(-4.55764236207275,1.93168318346768,27.2585179690208));
#60880=CARTESIAN_POINT('Ctrl Pts',(-3.91932380623715,3.43776204663053,27.2055977149389));
#60881=CARTESIAN_POINT('Ctrl Pts',(-2.46067639950694,4.59616252449921,27.1526774608569));
#60882=CARTESIAN_POINT('Ctrl Pts',(-0.849145821918294,4.87674835967949,
27.0997572067749));
#60883=CARTESIAN_POINT('Ctrl Pts',(0.762384755670364,5.15733419485977,27.046836952693));
#60884=CARTESIAN_POINT('Ctrl Pts',(2.52679850411746,4.56010538735165,26.993916698611));
#60885=CARTESIAN_POINT('Ctrl Pts',(3.63656998987608,3.35842905030792,26.940996444529));
#60886=CARTESIAN_POINT('Ctrl Pts',(4.7463414756347,2.15675271326421,26.8880761904471));
#60887=CARTESIAN_POINT('Ctrl Pts',(5.20147069870486,0.350628846684903,26.8351559363651));
#60888=CARTESIAN_POINT('Ctrl Pts',(4.79388038130065,-1.23355926618448,26.7822356822831));
#60889=CARTESIAN_POINT('Ctrl Pts',(4.38629006389643,-2.81774737905389,26.7293154282012));
#60890=CARTESIAN_POINT('Ctrl Pts',(3.11598020601782,-4.17999973821337,26.6763951741192));
#60891=CARTESIAN_POINT('Ctrl Pts',(1.56388702368888,-4.69668637868557,26.6234749200373));
#60892=CARTESIAN_POINT('Ctrl Pts',(0.011793841359943,-5.21337301915776,
26.5705546659553));
#60893=CARTESIAN_POINT('Ctrl Pts',(-1.82208266541932,-4.88449394094269,
26.5176344118733));
#60894=CARTESIAN_POINT('Ctrl Pts',(-3.09781019267902,-3.86101403671482,
26.4647141577914));
#60895=CARTESIAN_POINT('Ctrl Pts',(-4.24201965745686,-2.94304733269382,
26.4172495900799));
#60896=CARTESIAN_POINT('Ctrl Pts',(-4.93723014327371,-1.46631393177114,
26.3697850223684));
#60897=CARTESIAN_POINT('Ctrl Pts',(-4.94751652564198,0.00256483971322934,
26.3223204546569));
#60898=CARTESIAN_POINT('Ctrl Pts',(-4.94433041235646,0.00147179461986118,
26.1776795453432));
#60899=CARTESIAN_POINT('Ctrl Pts',(-4.93206642200618,-1.44411412527272,
26.2242935383928));
#60900=CARTESIAN_POINT('Ctrl Pts',(-4.26830822622625,-2.89170283737207,
26.2709075314422));
#60901=CARTESIAN_POINT('Ctrl Pts',(-3.16027114216866,-3.81000496542323,
26.3175215244917));
#60902=CARTESIAN_POINT('Ctrl Pts',(-1.90233119357243,-4.85254131044005,
26.3704417785737));
#60903=CARTESIAN_POINT('Ctrl Pts',(-0.071770729429417,-5.21289273822024,
26.4233620326557));
#60904=CARTESIAN_POINT('Ctrl Pts',(1.48894305049924,-4.72167819128264,26.4762822867377));
#60905=CARTESIAN_POINT('Ctrl Pts',(3.0496568304279,-4.23046364434503,26.5292025408196));
#60906=CARTESIAN_POINT('Ctrl Pts',(4.34052392614221,-2.88768312268964,26.5821227949016));
#60907=CARTESIAN_POINT('Ctrl Pts',(4.77319109373772,-1.30997581823277,26.6350430489835));
#60908=CARTESIAN_POINT('Ctrl Pts',(5.20585826133323,0.267731486224089,26.6879633030655));
#60909=CARTESIAN_POINT('Ctrl Pts',(4.78032550080995,2.08036557348242,26.7408835571475));
#60910=CARTESIAN_POINT('Ctrl Pts',(3.69010138443177,3.29954694578963,26.7938038112294));
#60911=CARTESIAN_POINT('Ctrl Pts',(2.59987726805358,4.51872831809683,26.8467240653114));
#60912=CARTESIAN_POINT('Ctrl Pts',(0.844961795820489,5.14445697545292,26.8996443193934));
#60913=CARTESIAN_POINT('Ctrl Pts',(-0.770932625263734,4.88981277963295,
26.9525645734753));
#60914=CARTESIAN_POINT('Ctrl Pts',(-2.38682704634796,4.63516858381299,27.0054848275573));
#60915=CARTESIAN_POINT('Ctrl Pts',(-3.86370041628332,3.50015153481698,27.0584050816393));
#60916=CARTESIAN_POINT('Ctrl Pts',(-4.52604495623161,2.00446386165791,27.1113253357212));
#60917=CARTESIAN_POINT('Ctrl Pts',(-4.80287247849846,1.37933979454018,27.1334434055952));
#60918=CARTESIAN_POINT('Ctrl Pts',(-4.93741567156095,0.691212705388757,
27.1555614754692));
#60919=CARTESIAN_POINT('Ctrl Pts',(-4.93474635697119,0.00209204260276723,
27.1776795453432));
#60920=CARTESIAN_POINT('Origin',(0.,0.,16.));
#60921=CARTESIAN_POINT('',(-4.93883733219525,-0.00423015144557837,28.3223204546569));
#60922=CARTESIAN_POINT('',(-4.93956784471338,-0.00436622746695347,28.1776795453432));
#60923=CARTESIAN_POINT('',(-4.942,-6.05220448138622E-16,16.));
#60924=CARTESIAN_POINT('Ctrl Pts',(-4.93883733219525,-0.00423015144557837,
28.3223204546569));
#60925=CARTESIAN_POINT('Ctrl Pts',(-4.92943499320705,1.14867573667121,28.2852411506033));
#60926=CARTESIAN_POINT('Ctrl Pts',(-4.52687920768094,2.30749865084404,28.2481618465497));
#60927=CARTESIAN_POINT('Ctrl Pts',(-3.78946858460819,3.18489002165513,28.2110825424962));
#60928=CARTESIAN_POINT('Ctrl Pts',(-2.73702279222337,4.43711887162355,28.1581622884142));
#60929=CARTESIAN_POINT('Ctrl Pts',(-1.00249392936347,5.11608531143494,28.1052420343322));
#60930=CARTESIAN_POINT('Ctrl Pts',(0.62037219239006,4.91108322945104,28.0523217802503));
#60931=CARTESIAN_POINT('Ctrl Pts',(2.2432383141436,4.70608114746714,27.9994015261683));
#60932=CARTESIAN_POINT('Ctrl Pts',(3.75444169479077,3.61711054368793,27.9464812720863));
#60933=CARTESIAN_POINT('Ctrl Pts',(4.46243050532182,2.1425023369291,27.8935610180044));
#60934=CARTESIAN_POINT('Ctrl Pts',(5.17041931585287,0.667894130170271,27.8406407639224));
#60935=CARTESIAN_POINT('Ctrl Pts',(5.07519355626782,-1.19235167956817,27.7877205098404));
#60936=CARTESIAN_POINT('Ctrl Pts',(4.22033397580047,-2.58696076330049,27.7348002557585));
#60937=CARTESIAN_POINT('Ctrl Pts',(3.36547439533311,-3.98156984703282,27.6818800016765));
#60938=CARTESIAN_POINT('Ctrl Pts',(1.75098099398345,-4.91054220475902,27.6289597475946));
#60939=CARTESIAN_POINT('Ctrl Pts',(0.115662973237938,-4.94876098597613,
27.5760394935126));
#60940=CARTESIAN_POINT('Ctrl Pts',(-1.51965504750756,-4.98697976719323,
27.5231192394306));
#60941=CARTESIAN_POINT('Ctrl Pts',(-3.17579768764892,-4.13444497190124,
27.4701989853487));
#60942=CARTESIAN_POINT('Ctrl Pts',(-4.09487415524911,-2.78129895002674,
27.4172787312667));
#60943=CARTESIAN_POINT('Ctrl Pts',(-4.6445938479574,-1.97195278400361,27.3856259723968));
#60944=CARTESIAN_POINT('Ctrl Pts',(-4.9306283269799,-0.98351309398954,27.3539732135268));
#60945=CARTESIAN_POINT('Ctrl Pts',(-4.93516121822955,0.00250487983550263,
27.3223204546569));
#60946=CARTESIAN_POINT('Ctrl Pts',(-4.93474635697119,0.00209204260276723,
27.1776795453432));
#60947=CARTESIAN_POINT('Ctrl Pts',(-4.93102900187776,-0.957594843168012,
27.2084817295512));
#60948=CARTESIAN_POINT('Ctrl Pts',(-4.66120098345796,-1.91920867090262,
27.2392839137591));
#60949=CARTESIAN_POINT('Ctrl Pts',(-4.13896060662357,-2.7152702966968,27.2700860979671));
#60950=CARTESIAN_POINT('Ctrl Pts',(-3.24171600710599,-4.08295848457032,
27.3230063520491));
#60951=CARTESIAN_POINT('Ctrl Pts',(-1.59941109810958,-4.96197656299522,
27.375926606131));
#60952=CARTESIAN_POINT('Ctrl Pts',(0.0363198151755977,-4.94999037586593,
27.428846860213));
#60953=CARTESIAN_POINT('Ctrl Pts',(1.67205072846078,-4.93800418873663,27.481767114295));
#60954=CARTESIAN_POINT('Ctrl Pts',(3.30120764603473,-4.03501373605313,27.5346873683769));
#60955=CARTESIAN_POINT('Ctrl Pts',(4.17831072893992,-2.65428408264511,27.5876076224589));
#60956=CARTESIAN_POINT('Ctrl Pts',(5.0554138118451,-1.27355442923711,27.6405278765408));
#60957=CARTESIAN_POINT('Ctrl Pts',(5.18046306008153,0.584914424895401,27.6934481306228));
#60958=CARTESIAN_POINT('Ctrl Pts',(4.49620935947501,2.07068111644173,27.7463683847048));
#60959=CARTESIAN_POINT('Ctrl Pts',(3.81195565886849,3.55644780798807,27.7992886387867));
#60960=CARTESIAN_POINT('Ctrl Pts',(2.318399009419,4.66951233694822,27.8522088928687));
#60961=CARTESIAN_POINT('Ctrl Pts',(0.69902662395141,4.900507696898,27.9051291469507));
#60962=CARTESIAN_POINT('Ctrl Pts',(-0.920345761516168,5.13150305684779,
27.9580494010326));
#60963=CARTESIAN_POINT('Ctrl Pts',(-2.66553388300184,4.48042924778721,28.0109696551146));
#60964=CARTESIAN_POINT('Ctrl Pts',(-3.73791972674343,3.24523368575399,28.0638899091965));
#60965=CARTESIAN_POINT('Ctrl Pts',(-4.5065378238221,2.35992391786528,28.1018197879121));
#60966=CARTESIAN_POINT('Ctrl Pts',(-4.92952982972571,1.17454424098757,28.1397496666277));
#60967=CARTESIAN_POINT('Ctrl Pts',(-4.93956784471338,-0.00436622746695347,
28.1776795453432));
#60968=CARTESIAN_POINT('Origin',(0.,0.,16.));
#60969=CARTESIAN_POINT('',(-4.95011095070931,-1.6828919353247E-5,29.3223204546569));
#60970=CARTESIAN_POINT('',(-4.9500545842803,0.000473333830474247,29.1776795453432));
#60971=CARTESIAN_POINT('',(-4.942,-6.05220448138622E-16,16.));
#60972=CARTESIAN_POINT('Ctrl Pts',(-4.95011089075521,-1.68287949581236E-5,
29.3223204546569));
#60973=CARTESIAN_POINT('Ctrl Pts',(-4.95002830796364,1.63484509113909,29.2694293417618));
#60974=CARTESIAN_POINT('Ctrl Pts',(-4.06015814856933,3.2697840224184,29.2165382288666));
#60975=CARTESIAN_POINT('Ctrl Pts',(-2.68714856385847,4.15726245203154,29.1636471159715));
#60976=CARTESIAN_POINT('Ctrl Pts',(-1.31338249801809,5.04522985178176,29.1107268618895));
#60977=CARTESIAN_POINT('Ctrl Pts',(0.544055526265072,5.1849128728298,29.0578066078076));
#60978=CARTESIAN_POINT('Ctrl Pts',(2.03517352301083,4.51239041724249,29.0048863537256));
#60979=CARTESIAN_POINT('Ctrl Pts',(3.52629151975661,3.83986796165517,28.9519660996436));
#60980=CARTESIAN_POINT('Ctrl Pts',(4.65108948896497,2.3551400294325,28.8990458455617));
#60981=CARTESIAN_POINT('Ctrl Pts',(4.89484265904535,0.737640825291349,28.8461255914797));
#60982=CARTESIAN_POINT('Ctrl Pts',(5.13859582912572,-0.879858378849781,
28.7932053373978));
#60983=CARTESIAN_POINT('Ctrl Pts',(4.50130420007813,-2.63012885490939,28.7402850833158));
#60984=CARTESIAN_POINT('Ctrl Pts',(3.27460223530322,-3.71222015364772,28.6873648292338));
#60985=CARTESIAN_POINT('Ctrl Pts',(2.04790027052829,-4.79431145238607,28.6344445751519));
#60986=CARTESIAN_POINT('Ctrl Pts',(0.231787970026049,-5.20822357380314,
28.5815243210699));
#60987=CARTESIAN_POINT('Ctrl Pts',(-1.34265409528112,-4.76454391006902,
28.5286040669879));
#60988=CARTESIAN_POINT('Ctrl Pts',(-2.91709616058829,-4.3208642463349,28.475683812906));
#60989=CARTESIAN_POINT('Ctrl Pts',(-4.24986799070038,-3.01959279744957,
28.422763558824));
#60990=CARTESIAN_POINT('Ctrl Pts',(-4.73107254480156,-1.45621144294418,
28.369843304742));
#60991=CARTESIAN_POINT('Ctrl Pts',(-4.87511450807598,-0.988234742120547,
28.3540023547137));
#60992=CARTESIAN_POINT('Ctrl Pts',(-4.94285418164439,-0.496772420704347,
28.3381614046853));
#60993=CARTESIAN_POINT('Ctrl Pts',(-4.93883733219525,-0.00423015144557837,
28.3223204546569));
#60994=CARTESIAN_POINT('Ctrl Pts',(-4.93956784471338,-0.00436622746695347,
28.1776795453432));
#60995=CARTESIAN_POINT('Ctrl Pts',(-4.9435349971983,-0.470286790462875,
28.1926699207096));
#60996=CARTESIAN_POINT('Ctrl Pts',(-4.88300154657712,-0.935196907127989,
28.207660296076));
#60997=CARTESIAN_POINT('Ctrl Pts',(-4.75381137141076,-1.38017405347592,
28.2226506714425));
#60998=CARTESIAN_POINT('Ctrl Pts',(-4.29773360633903,-2.95106891566672,
28.2755709255244));
#60999=CARTESIAN_POINT('Ctrl Pts',(-2.98599451019808,-4.27354132504245,
28.3284911796064));
#61000=CARTESIAN_POINT('Ctrl Pts',(-1.41886776017779,-4.74240604726615,
28.3814114336883));
#61001=CARTESIAN_POINT('Ctrl Pts',(0.148258989842506,-5.21127076948986,
28.4343316877703));
#61002=CARTESIAN_POINT('Ctrl Pts',(1.97077339374215,-4.82652780456152,28.4872519418523));
#61003=CARTESIAN_POINT('Ctrl Pts',(3.21466598259635,-3.76424227707361,28.5401721959342));
#61004=CARTESIAN_POINT('Ctrl Pts',(4.45855857145055,-2.7019567495857,28.5930924500162));
#61005=CARTESIAN_POINT('Ctrl Pts',(5.1238293452593,-0.962128659538206,28.6460127040981));
#61006=CARTESIAN_POINT('Ctrl Pts',(4.90603973778863,0.659070540261458,28.6989329581801));
#61007=CARTESIAN_POINT('Ctrl Pts',(4.68825013031796,2.28026974006111,28.7518532122621));
#61008=CARTESIAN_POINT('Ctrl Pts',(3.58740014156788,3.78284004961294,28.8047734663441));
#61009=CARTESIAN_POINT('Ctrl Pts',(2.10725580021387,4.47918211041389,28.857693720426));
#61010=CARTESIAN_POINT('Ctrl Pts',(0.627111458859856,5.17552417121484,28.910613974508));
#61011=CARTESIAN_POINT('Ctrl Pts',(-1.23232723509808,5.0656379832649,28.9635342285899));
#61012=CARTESIAN_POINT('Ctrl Pts',(-2.62015287286002,4.19980926793105,29.0164544826719));
#61013=CARTESIAN_POINT('Ctrl Pts',(-4.00797851062198,3.33398055259719,29.0693747367538));
#61014=CARTESIAN_POINT('Ctrl Pts',(-4.92419109218792,1.71220930987939,29.1222949908358));
#61015=CARTESIAN_POINT('Ctrl Pts',(-4.94951767608282,0.0766427647882502,
29.1752152449178));
#61016=CARTESIAN_POINT('Ctrl Pts',(-4.94991079785034,0.0512553373413882,
29.1760366783929));
#61017=CARTESIAN_POINT('Ctrl Pts',(-4.95008927347619,0.0258645861152391,
29.1768581118681));
#61018=CARTESIAN_POINT('Ctrl Pts',(-4.9500545842803,0.000473333830474247,
29.1776795453432));
#61019=CARTESIAN_POINT('Origin',(0.,0.,16.));
#61020=CARTESIAN_POINT('',(-4.93888642291793,0.00424076360118208,30.3223204546569));
#61021=CARTESIAN_POINT('',(-4.93818673588435,0.0040670116119004,30.1776795453432));
#61022=CARTESIAN_POINT('',(-4.942,-6.05220448138622E-16,16.));
#61023=CARTESIAN_POINT('Ctrl Pts',(-4.93888642291793,0.00424076360118208,
30.3223204546569));
#61024=CARTESIAN_POINT('Ctrl Pts',(-4.94290141421135,0.49495855667818,30.3065377870022));
#61025=CARTESIAN_POINT('Ctrl Pts',(-4.87566910369714,0.984600773625852,
30.2907551193474));
#61026=CARTESIAN_POINT('Ctrl Pts',(-4.7326693925228,1.45101307944963,30.2749724516927));
#61027=CARTESIAN_POINT('Ctrl Pts',(-4.25318257733109,3.01492218981842,30.2220521976108));
#61028=CARTESIAN_POINT('Ctrl Pts',(-2.92184129195003,4.31765692360063,30.1691319435288));
#61029=CARTESIAN_POINT('Ctrl Pts',(-1.3478876419775,4.76306597049205,30.1162116894468));
#61030=CARTESIAN_POINT('Ctrl Pts',(0.226066007995039,5.20847501738348,30.0632914353649));
#61031=CARTESIAN_POINT('Ctrl Pts',(2.04263202255905,4.79655837738413,30.0103711812829));
#61032=CARTESIAN_POINT('Ctrl Pts',(3.27052205003055,3.71581539574951,29.9574509272009));
#61033=CARTESIAN_POINT('Ctrl Pts',(4.49841207750204,2.6350724141149,29.904530673119));
#61034=CARTESIAN_POINT('Ctrl Pts',(5.13762611788102,0.885503090845023,29.851610419037));
#61035=CARTESIAN_POINT('Ctrl Pts',(4.89565006291192,-0.732262930536752,
29.798690164955));
#61036=CARTESIAN_POINT('Ctrl Pts',(4.65367400794282,-2.35002895191851,29.7457699108731));
#61037=CARTESIAN_POINT('Ctrl Pts',(3.53050785762567,-3.83599167141216,29.6928496567911));
#61038=CARTESIAN_POINT('Ctrl Pts',(2.04012959776072,-4.51015185496902,29.6399294027091));
#61039=CARTESIAN_POINT('Ctrl Pts',(0.549751337895761,-5.18431203852589,
29.5870091486272));
#61040=CARTESIAN_POINT('Ctrl Pts',(-1.307839031517,-5.04666968614595,29.5340888945452));
#61041=CARTESIAN_POINT('Ctrl Pts',(-2.68257979015076,-4.16021203843222,
29.4811686404633));
#61042=CARTESIAN_POINT('Ctrl Pts',(-4.05807756664059,-3.27326625194488,
29.4282192451945));
#61043=CARTESIAN_POINT('Ctrl Pts',(-4.95019356454733,-1.6366802542765,29.3752698499257));
#61044=CARTESIAN_POINT('Ctrl Pts',(-4.95011089075521,-1.68287949581236E-5,
29.3223204546569));
#61045=CARTESIAN_POINT('Ctrl Pts',(-4.9500545842803,0.000473333830474247,
29.1776795453432));
#61046=CARTESIAN_POINT('Ctrl Pts',(-4.94785444726563,-1.60994837137546,
29.2297783659501));
#61047=CARTESIAN_POINT('Ctrl Pts',(-4.08816932384676,-3.22238565418073,
29.2818771865568));
#61048=CARTESIAN_POINT('Ctrl Pts',(-2.74893267905414,-4.11666957233305,
29.3339760071636));
#61049=CARTESIAN_POINT('Ctrl Pts',(-1.38858051190673,-5.0250535168987,29.3868962612456));
#61050=CARTESIAN_POINT('Ctrl Pts',(0.466564408611941,-5.19245955856552,
29.4398165153276));
#61051=CARTESIAN_POINT('Ctrl Pts',(1.96755945318719,-4.54228015350161,29.4927367694096));
#61052=CARTESIAN_POINT('Ctrl Pts',(3.46855449776245,-3.8921007484377,29.5456570234915));
#61053=CARTESIAN_POINT('Ctrl Pts',(4.61539966639428,-2.42433589664307,29.5985772775735));
#61054=CARTESIAN_POINT('Ctrl Pts',(4.88328108437524,-0.810657201852559,
29.6514975316554));
#61055=CARTESIAN_POINT('Ctrl Pts',(5.15116250235621,0.803021492937955,29.7044177857374));
#61056=CARTESIAN_POINT('Ctrl Pts',(4.54008016968629,2.56261403072434,29.7573380398194));
#61057=CARTESIAN_POINT('Ctrl Pts',(3.3296746999557,3.66290398769728,29.8102582939013));
#61058=CARTESIAN_POINT('Ctrl Pts',(2.11926923022511,4.76319394467022,29.8631785479833));
#61059=CARTESIAN_POINT('Ctrl Pts',(0.309540623433855,5.20418132082974,29.9160988020653));
#61060=CARTESIAN_POINT('Ctrl Pts',(-1.27135167326916,4.78406356027939,29.9690190561472));
#61061=CARTESIAN_POINT('Ctrl Pts',(-2.85224396997218,4.36394579972904,30.0219393102292));
#61062=CARTESIAN_POINT('Ctrl Pts',(-4.20429995658695,3.0827229024688,30.0748595643112));
#61063=CARTESIAN_POINT('Ctrl Pts',(-4.70879816265426,1.5267020327104,30.1277798183931));
#61064=CARTESIAN_POINT('Ctrl Pts',(-4.86736582366476,1.03763272218799,30.1444130607098));
#61065=CARTESIAN_POINT('Ctrl Pts',(-4.94220382950374,0.521416307353422,
30.1610463030265));
#61066=CARTESIAN_POINT('Ctrl Pts',(-4.93818673588435,0.0040670116119004,
30.1776795453432));
#61067=CARTESIAN_POINT('Origin',(0.,0.,16.));
#61068=CARTESIAN_POINT('',(-4.9351415428321,-0.00248504100164359,31.3223204546569));
#61069=CARTESIAN_POINT('',(-4.93557330743154,-0.0028385321285674,31.1776795453432));
#61070=CARTESIAN_POINT('',(-4.942,-6.05220448138622E-16,16.));
#61071=CARTESIAN_POINT('Ctrl Pts',(-4.9351415428321,-0.00248504100164359,
31.3223204546569));
#61072=CARTESIAN_POINT('Ctrl Pts',(-4.93066017409234,0.981733357670619,
31.2907259781606));
#61073=CARTESIAN_POINT('Ctrl Pts',(-4.6457448695693,1.96834170751759,31.2591315016643));
#61074=CARTESIAN_POINT('Ctrl Pts',(-4.09792294976925,2.77680140323666,31.227537025168));
#61075=CARTESIAN_POINT('Ctrl Pts',(-3.18032980050788,4.13095875151604,31.1746167710861));
#61076=CARTESIAN_POINT('Ctrl Pts',(-1.52513305096331,4.98530711426681,31.1216965170041));
#61077=CARTESIAN_POINT('Ctrl Pts',(0.110223986946674,4.94888363249201,31.0687762629222));
#61078=CARTESIAN_POINT('Ctrl Pts',(1.74558102485669,4.91246015071721,31.0158560088402));
#61079=CARTESIAN_POINT('Ctrl Pts',(3.36109835113211,3.98526482441679,30.9629357547582));
#61080=CARTESIAN_POINT('Ctrl Pts',(4.2174905639687,2.59159639567501,30.9100155006763));
#61081=CARTESIAN_POINT('Ctrl Pts',(5.0738827768053,1.19792796693324,30.8570952465943));
#61082=CARTESIAN_POINT('Ctrl Pts',(5.17114987620307,-0.662213564249888,
30.8041749925123));
#61083=CARTESIAN_POINT('Ctrl Pts',(4.46478095192916,-2.13759902381238,30.7512547384304));
#61084=CARTESIAN_POINT('Ctrl Pts',(3.75841202765526,-3.61298448337487,30.6983344843484));
#61085=CARTESIAN_POINT('Ctrl Pts',(2.2484070797097,-4.70361387131672,30.6454142302665));
#61086=CARTESIAN_POINT('Ctrl Pts',(0.625767434156371,-4.91039852288288,
30.5924939761845));
#61087=CARTESIAN_POINT('Ctrl Pts',(-0.996872211396971,-5.11718317444904,
30.5395737221025));
#61088=CARTESIAN_POINT('Ctrl Pts',(-2.73214655455809,-4.44012308963949,
30.4866534680206));
#61089=CARTESIAN_POINT('Ctrl Pts',(-3.78596755363747,-3.18905130375701,
30.4337332139386));
#61090=CARTESIAN_POINT('Ctrl Pts',(-4.52550233311024,-2.31109280977609,
30.3965956275114));
#61091=CARTESIAN_POINT('Ctrl Pts',(-4.92943890178742,-1.1504483453926,30.3594580410841));
#61092=CARTESIAN_POINT('Ctrl Pts',(-4.93888642291793,0.00424076360118208,
30.3223204546569));
#61093=CARTESIAN_POINT('Ctrl Pts',(-4.93818673588435,0.0040670116119004,
30.1776795453432));
#61094=CARTESIAN_POINT('Ctrl Pts',(-4.92942306127099,-1.12458004491972,
30.2139665571085));
#61095=CARTESIAN_POINT('Ctrl Pts',(-4.54535955813864,-2.25861888984588,
30.2502535688737));
#61096=CARTESIAN_POINT('Ctrl Pts',(-3.83660874069347,-3.12794382961597,
30.286540580639));
#61097=CARTESIAN_POINT('Ctrl Pts',(-2.80298068714555,-4.39574997992736,
30.339460834721));
#61098=CARTESIAN_POINT('Ctrl Pts',(-1.0787841545299,-5.10054343829356,30.3923810888029));
#61099=CARTESIAN_POINT('Ctrl Pts',(0.546962191086786,-4.91979995442398,
30.4453013428849));
#61100=CARTESIAN_POINT('Ctrl Pts',(2.17270853670347,-4.73905647055441,30.4982215969669));
#61101=CARTESIAN_POINT('Ctrl Pts',(3.7000046953212,-3.67277604444905,30.5511418510488));
#61102=CARTESIAN_POINT('Ctrl Pts',(4.4299366186172,-2.20890488388769,30.6040621051308));
#61103=CARTESIAN_POINT('Ctrl Pts',(5.1598685419132,-0.745033723326325,30.6569823592128));
#61104=CARTESIAN_POINT('Ctrl Pts',(5.09243622988746,1.11642817169105,30.7099026132947));
#61105=CARTESIAN_POINT('Ctrl Pts',(4.25849773850338,2.52364740836047,30.7628228673767));
#61106=CARTESIAN_POINT('Ctrl Pts',(3.42455924711931,3.93086664502988,30.8157431214587));
#61107=CARTESIAN_POINT('Ctrl Pts',(1.8241145763769,4.88384322335134,30.8686633755406));
#61108=CARTESIAN_POINT('Ctrl Pts',(0.189551650661496,4.9464805066113,30.9215836296226));
#61109=CARTESIAN_POINT('Ctrl Pts',(-1.44501127505389,5.00911778987126,30.9745038837045));
#61110=CARTESIAN_POINT('Ctrl Pts',(-3.11369245574226,4.18141577806974,31.0274241377865));
#61111=CARTESIAN_POINT('Ctrl Pts',(-4.05287789782628,2.84214355302423,31.0803443918685));
#61112=CARTESIAN_POINT('Ctrl Pts',(-4.62868616337827,2.0210447769463,31.1127894430267));
#61113=CARTESIAN_POINT('Ctrl Pts',(-4.93028912913986,1.0076552769297,31.145234494185));
#61114=CARTESIAN_POINT('Ctrl Pts',(-4.93557330743154,-0.0028385321285674,
31.1776795453432));
#61115=CARTESIAN_POINT('Origin',(0.,0.,16.));
#61116=CARTESIAN_POINT('',(-4.94795422753399,-0.0028972882267797,32.3223204546569));
#61117=CARTESIAN_POINT('',(-4.94851874366221,-0.00251525819571033,32.1776795453432));
#61118=CARTESIAN_POINT('',(-4.942,-6.05220448138622E-16,16.));
#61119=CARTESIAN_POINT('Ctrl Pts',(-4.94795422753399,-0.0028972882267797,
32.3223204546569));
#61120=CARTESIAN_POINT('Ctrl Pts',(-4.93774012235113,1.46412544671205,32.2749141693191));
#61121=CARTESIAN_POINT('Ctrl Pts',(-4.24380482164535,2.93954073272814,32.2275078839812));
#61122=CARTESIAN_POINT('Ctrl Pts',(-3.10183998936669,3.85774379859783,32.1801015986434));
#61123=CARTESIAN_POINT('Ctrl Pts',(-1.82704976595674,4.88274584628794,32.1271813445614));
#61124=CARTESIAN_POINT('Ctrl Pts',(0.00605460139836145,5.21337522038518,
32.0742610904795));
#61125=CARTESIAN_POINT('Ctrl Pts',(1.55861655774584,4.69833086969986,32.0213408363975));
#61126=CARTESIAN_POINT('Ctrl Pts',(3.11117851409333,4.18328651901453,31.9684205823155));
#61127=CARTESIAN_POINT('Ctrl Pts',(4.38319805943319,2.82256844354664,31.9155003282335));
#61128=CARTESIAN_POINT('Ctrl Pts',(4.79257962264663,1.23886201646757,31.8625800741516));
#61129=CARTESIAN_POINT('Ctrl Pts',(5.20196118586006,-0.344844410611489,
31.8096598200696));
#61130=CARTESIAN_POINT('Ctrl Pts',(4.74870476694708,-2.15153918930172,31.7567395659877));
#61131=CARTESIAN_POINT('Ctrl Pts',(3.64022742565071,-3.35445119576896,31.7038193119057));
#61132=CARTESIAN_POINT('Ctrl Pts',(2.53175008435434,-4.5573632022362,31.6508990578238));
#61133=CARTESIAN_POINT('Ctrl Pts',(0.768051820674579,-5.15649243648045,
31.5979788037418));
#61134=CARTESIAN_POINT('Ctrl Pts',(-0.843772103495588,-4.87766821059161,
31.5450585496598));
#61135=CARTESIAN_POINT('Ctrl Pts',(-2.45559602766576,-4.59884398470276,
31.4921382955779));
#61136=CARTESIAN_POINT('Ctrl Pts',(-3.91554561232635,-3.44206629868081,
31.4392180414959));
#61137=CARTESIAN_POINT('Ctrl Pts',(-4.55552563016757,-1.93669428876581,
31.386297787414));
#61138=CARTESIAN_POINT('Ctrl Pts',(-4.81342445844275,-1.33006022730727,
31.3649720098283));
#61139=CARTESIAN_POINT('Ctrl Pts',(-4.93816639665535,-0.66681706968053,
31.3436462322426));
#61140=CARTESIAN_POINT('Ctrl Pts',(-4.9351415428321,-0.00248504100164359,
31.3223204546569));
#61141=CARTESIAN_POINT('Ctrl Pts',(-4.93557330743154,-0.0028385321285674,
31.1776795453432));
#61142=CARTESIAN_POINT('Ctrl Pts',(-4.93890801084376,-0.640534114505631,
31.1981547482669));
#61143=CARTESIAN_POINT('Ctrl Pts',(-4.82423274680824,-1.27707647808528,
31.2186299511906));
#61144=CARTESIAN_POINT('Ctrl Pts',(-4.58598979744053,-1.86340999470999,
31.2391051541143));
#61145=CARTESIAN_POINT('Ctrl Pts',(-3.97022655149108,-3.3788488791092,31.2920254081963));
#61146=CARTESIAN_POINT('Ctrl Pts',(-2.5290103561125,-4.55888420961813,31.3449456622783));
#61147=CARTESIAN_POINT('Ctrl Pts',(-0.921863753563045,-4.86351379667883,
31.3978659163602));
#61148=CARTESIAN_POINT('Ctrl Pts',(0.685282848986421,-5.16814338373953,
31.4507861704422));
#61149=CARTESIAN_POINT('Ctrl Pts',(2.45835985870677,-4.59736722735202,31.5037064245242));
#61150=CARTESIAN_POINT('Ctrl Pts',(3.5859801562746,-3.4123812139678,31.5566266786061));
#61151=CARTESIAN_POINT('Ctrl Pts',(4.71360045384243,-2.22739520058358,31.6095469326881));
#61152=CARTESIAN_POINT('Ctrl Pts',(5.19576403925773,-0.428199330202661,
31.6624671867701));
#61153=CARTESIAN_POINT('Ctrl Pts',(4.81182549189739,1.16186688830996,31.715387440852));
#61154=CARTESIAN_POINT('Ctrl Pts',(4.42788694453706,2.75193310682255,31.768307694934));
#61155=CARTESIAN_POINT('Ctrl Pts',(3.17784626440109,4.13286967346687,31.8212279490159));
#61156=CARTESIAN_POINT('Ctrl Pts',(1.63374115821347,4.67273892471915,31.8741482030979));
#61157=CARTESIAN_POINT('Ctrl Pts',(0.0896360520258116,5.21260817597145,
31.9270684571799));
#61158=CARTESIAN_POINT('Ctrl Pts',(-1.74853348021352,4.91141011183171,31.9799887112618));
#61159=CARTESIAN_POINT('Ctrl Pts',(-3.0395929867415,3.90697756655707,32.0329089653438));
#61160=CARTESIAN_POINT('Ctrl Pts',(-4.21688283424399,2.99105678050979,32.0811658253436));
#61161=CARTESIAN_POINT('Ctrl Pts',(-4.93923809973741,1.49038033345358,32.1294226853434));
#61162=CARTESIAN_POINT('Ctrl Pts',(-4.94851874366221,-0.00251525819571033,
32.1776795453432));
#61163=CARTESIAN_POINT('Origin',(0.,0.,16.));
#61164=CARTESIAN_POINT('',(-4.94391378591308,0.00432614989180041,33.3223204546569));
#61165=CARTESIAN_POINT('',(-4.943114998001,0.00443591996608837,33.1776795453432));
#61166=CARTESIAN_POINT('',(-4.942,-6.05220448138622E-16,16.));
#61167=CARTESIAN_POINT('Ctrl Pts',(-4.94391378591308,0.00432614989180041,
33.3223204546569));
#61168=CARTESIAN_POINT('Ctrl Pts',(-4.94684012248784,0.323678273041629,
33.3120226145595));
#61169=CARTESIAN_POINT('Ctrl Pts',(-4.91854579890533,0.642514059921896,
33.3017247744621));
#61170=CARTESIAN_POINT('Ctrl Pts',(-4.8571468315969,0.954841972036427,33.2914269343646));
#61171=CARTESIAN_POINT('Ctrl Pts',(-4.54161960262542,2.55988461298029,33.2385066802827));
#61172=CARTESIAN_POINT('Ctrl Pts',(-3.3518326489115,3.99306094874791,33.1855864262007));
#61173=CARTESIAN_POINT('Ctrl Pts',(-1.83225065173251,4.59852759962142,33.1326661721187));
#61174=CARTESIAN_POINT('Ctrl Pts',(-0.312668654553525,5.20399425049493,
33.0797459180367));
#61175=CARTESIAN_POINT('Ctrl Pts',(1.53670838609054,4.98175121647435,33.0268256639548));
#61176=CARTESIAN_POINT('Ctrl Pts',(2.86957729142234,4.03350030417842,32.9739054098728));
#61177=CARTESIAN_POINT('Ctrl Pts',(4.20244619675414,3.0852493918825,32.9209851557909));
#61178=CARTESIAN_POINT('Ctrl Pts',(5.01880696677368,1.41099060131123,32.8680649017089));
#61179=CARTESIAN_POINT('Ctrl Pts',(4.94508044508782,-0.223109674519649,
32.8151446476269));
#61180=CARTESIAN_POINT('Ctrl Pts',(4.87135392340196,-1.85720995035054,32.762224393545));
#61181=CARTESIAN_POINT('Ctrl Pts',(3.90754011001068,-3.45115171144104,32.709304139463));
#61182=CARTESIAN_POINT('Ctrl Pts',(2.49469492595997,-4.27552286412362,32.6563838853811));
#61183=CARTESIAN_POINT('Ctrl Pts',(1.08184974190924,-5.0998940168062,32.6034636312991));
#61184=CARTESIAN_POINT('Ctrl Pts',(-0.780026812800927,-5.15469456108083,
32.5505433772171));
#61185=CARTESIAN_POINT('Ctrl Pts',(-2.2389115908552,-4.41484693093525,32.4976231231352));
#61186=CARTESIAN_POINT('Ctrl Pts',(-3.69779636890945,-3.67499930078968,
32.4447028690532));
#61187=CARTESIAN_POINT('Ctrl Pts',(-4.75368937030783,-2.14050349622394,
32.3917826149712));
#61188=CARTESIAN_POINT('Ctrl Pts',(-4.92339783127462,-0.513568233299591,
32.3388623608893));
#61189=CARTESIAN_POINT('Ctrl Pts',(-4.94108042115667,-0.344051469933491,
32.3333483921451));
#61190=CARTESIAN_POINT('Ctrl Pts',(-4.94914226106849,-0.173531149322059,
32.327834423401));
#61191=CARTESIAN_POINT('Ctrl Pts',(-4.94795422753399,-0.0028972882267797,
32.3223204546569));
#61192=CARTESIAN_POINT('Ctrl Pts',(-4.94851874366221,-0.00251525819571033,
32.1776795453432));
#61193=CARTESIAN_POINT('Ctrl Pts',(-4.94941559646112,-0.146784082719192,
32.1823429394254));
#61194=CARTESIAN_POINT('Ctrl Pts',(-4.9436532640282,-0.290980244219974,
32.1870063335075));
#61195=CARTESIAN_POINT('Ctrl Pts',(-4.93099878465363,-0.434569000702025,
32.1916697275897));
#61196=CARTESIAN_POINT('Ctrl Pts',(-4.78739559522113,-2.06401599627693,
32.2445899816717));
#61197=CARTESIAN_POINT('Ctrl Pts',(-3.75623973553951,-3.61524296101718,
32.2975102357536));
#61198=CARTESIAN_POINT('Ctrl Pts',(-2.30940387553184,-4.3783847444355,32.3504304898356));
#61199=CARTESIAN_POINT('Ctrl Pts',(-0.862568015524189,-5.14152652785381,
32.4033507439175));
#61200=CARTESIAN_POINT('Ctrl Pts',(0.999947844809495,-5.11658312995021,
32.4562709979995));
#61201=CARTESIAN_POINT('Ctrl Pts',(2.4258280021366,-4.3149690305583,32.5091912520815));
#61202=CARTESIAN_POINT('Ctrl Pts',(3.85170815946372,-3.51335493116639,32.5621115061634));
#61203=CARTESIAN_POINT('Ctrl Pts',(4.84095261378425,-1.93507013028614,32.6150317602454));
#61204=CARTESIAN_POINT('Ctrl Pts',(4.9408679943685,-0.30236185746891,32.6679520143274));
#61205=CARTESIAN_POINT('Ctrl Pts',(5.04078337495275,1.33034641534833,32.7208722684093));
#61206=CARTESIAN_POINT('Ctrl Pts',(4.25136968180072,3.01747816010256,32.7737925224913));
#61207=CARTESIAN_POINT('Ctrl Pts',(2.93387467737636,3.9869761233392,32.8267127765732));
#61208=CARTESIAN_POINT('Ctrl Pts',(1.616379672952,4.95647408657584,32.8796330306552));
#61209=CARTESIAN_POINT('Ctrl Pts',(-0.229196642744684,5.20833826829488,
32.9325532847372));
#61210=CARTESIAN_POINT('Ctrl Pts',(-1.75829036071957,4.62731177229585,32.9854735388191));
#61211=CARTESIAN_POINT('Ctrl Pts',(-3.28738407869442,4.04628527629685,33.0383937929011));
#61212=CARTESIAN_POINT('Ctrl Pts',(-4.49999519894748,2.63236810257984,33.091314046983));
#61213=CARTESIAN_POINT('Ctrl Pts',(-4.8412143530065,1.03259034416892,33.144234301065));
#61214=CARTESIAN_POINT('Ctrl Pts',(-4.91309708900794,0.695574086725974,
33.1553827158244));
#61215=CARTESIAN_POINT('Ctrl Pts',(-4.94630788623483,0.350309429675576,
33.1665311305838));
#61216=CARTESIAN_POINT('Ctrl Pts',(-4.943114998001,0.00443591996608837,
33.1776795453432));
#61217=CARTESIAN_POINT('Origin',(0.,0.,16.));
#61218=CARTESIAN_POINT('',(-4.93390856647989,0.000179243442527399,34.3223204546569));
#61219=CARTESIAN_POINT('',(-4.93391474235666,-0.000255694835337854,34.1776795453433));
#61220=CARTESIAN_POINT('',(-4.942,-6.05220448138622E-16,16.));
#61221=CARTESIAN_POINT('Ctrl Pts',(-4.93390856647989,0.000179243442527399,
34.3223204546569));
#61222=CARTESIAN_POINT('Ctrl Pts',(-4.93417188922503,0.81404442559312,34.2962108057179));
#61223=CARTESIAN_POINT('Ctrl Pts',(-4.7439659144325,1.62779374632659,34.2701011567789));
#61224=CARTESIAN_POINT('Ctrl Pts',(-4.36261434797766,2.33905848282458,34.24399150784));
#61225=CARTESIAN_POINT('Ctrl Pts',(-3.58967320891792,3.780683020289,34.191071253758));
#61226=CARTESIAN_POINT('Ctrl Pts',(-2.03148547319181,4.80128989115793,34.138150999676));
#61227=CARTESIAN_POINT('Ctrl Pts',(-0.401101646399658,4.93383380390034,
34.0852307455941));
#61228=CARTESIAN_POINT('Ctrl Pts',(1.22928218039249,5.06637771664275,34.0323104915121));
#61229=CARTESIAN_POINT('Ctrl Pts',(2.93186209825069,4.31085867125863,33.9793902374301));
#61230=CARTESIAN_POINT('Ctrl Pts',(3.92751153377263,3.01301372173064,33.9264699833482));
#61231=CARTESIAN_POINT('Ctrl Pts',(4.92316096929458,1.71516877220265,33.8735497292662));
#61232=CARTESIAN_POINT('Ctrl Pts',(5.21187992248028,-0.125002081469193,
33.8206294751842));
#61233=CARTESIAN_POINT('Ctrl Pts',(4.66154619083434,-1.6654085522694,33.7677092211023));
#61234=CARTESIAN_POINT('Ctrl Pts',(4.1112124591884,-3.2058150230696,33.7147889670203));
#61235=CARTESIAN_POINT('Ctrl Pts',(2.72182604271081,-4.44645711099814,33.6618687129384));
#61236=CARTESIAN_POINT('Ctrl Pts',(1.12919138526205,-4.8195980486659,33.6089484588564));
#61237=CARTESIAN_POINT('Ctrl Pts',(-0.463443272186686,-5.19273898633366,
33.5560282047744));
#61238=CARTESIAN_POINT('Ctrl Pts',(-2.25932617060659,-4.69837877374066,
33.5031079506925));
#61239=CARTESIAN_POINT('Ctrl Pts',(-3.43663386770201,-3.56274419438412,
33.4501876966105));
#61240=CARTESIAN_POINT('Ctrl Pts',(-4.384847305511,-2.64809463314952,33.407565282626));
#61241=CARTESIAN_POINT('Ctrl Pts',(-4.93180177720373,-1.3174615522823,33.3649428686414));
#61242=CARTESIAN_POINT('Ctrl Pts',(-4.94391378591308,0.00432614989180041,
33.3223204546569));
#61243=CARTESIAN_POINT('Ctrl Pts',(-4.943114998001,0.00443591996608837,
33.1776795453432));
#61244=CARTESIAN_POINT('Ctrl Pts',(-4.93115160973848,-1.2915126956278,33.2194513846658));
#61245=CARTESIAN_POINT('Ctrl Pts',(-4.40811124636647,-2.59600908794704,
33.2612232239884));
#61246=CARTESIAN_POINT('Ctrl Pts',(-3.49331109260409,-3.50718930782419,
33.3029950633109));
#61247=CARTESIAN_POINT('Ctrl Pts',(-2.33436149027767,-4.6615528583015,33.3559153173929));
#61248=CARTESIAN_POINT('Ctrl Pts',(-0.54663509775989,-5.18464161615124,
33.4088355714748));
#61249=CARTESIAN_POINT('Ctrl Pts',(1.0517771843263,-4.83708217680429,33.4617558255568));
#61250=CARTESIAN_POINT('Ctrl Pts',(2.65018946641248,-4.48952273745735,33.5146760796387));
#61251=CARTESIAN_POINT('Ctrl Pts',(4.05928763806706,-3.27131510091373,33.5675963337207));
#61252=CARTESIAN_POINT('Ctrl Pts',(4.63424685520885,-1.73992968697417,33.6205165878027));
#61253=CARTESIAN_POINT('Ctrl Pts',(5.20920607235062,-0.208544273034641,
33.6734368418847));
#61254=CARTESIAN_POINT('Ctrl Pts',(4.95002633497964,1.63601891830083,33.7263570959666));
#61255=CARTESIAN_POINT('Ctrl Pts',(3.97531224929094,2.94965959921896,33.7792773500486));
#61256=CARTESIAN_POINT('Ctrl Pts',(3.00059816360222,4.26330028013712,33.8321976041305));
#61257=CARTESIAN_POINT('Ctrl Pts',(1.31034972959575,5.04601845063795,33.8851178582125));
#61258=CARTESIAN_POINT('Ctrl Pts',(-0.321949554671762,4.93963032168135,
33.9380381122945));
#61259=CARTESIAN_POINT('Ctrl Pts',(-1.95424883893928,4.83324219272475,33.9909583663764));
#61260=CARTESIAN_POINT('Ctrl Pts',(-3.52859897346783,3.83774776431073,34.0438786204584));
#61261=CARTESIAN_POINT('Ctrl Pts',(-4.32455329212167,2.40870049076816,34.0967988745404));
#61262=CARTESIAN_POINT('Ctrl Pts',(-4.73005222214988,1.68067235297088,34.1237590981413));
#61263=CARTESIAN_POINT('Ctrl Pts',(-4.93352684267558,0.840120210825594,
34.1507193217423));
#61264=CARTESIAN_POINT('Ctrl Pts',(-4.93391474235666,-0.000255694835337854,
34.1776795453433));
#61265=CARTESIAN_POINT('Origin',(0.,0.,16.));
#61266=CARTESIAN_POINT('',(-4.94325592752636,-0.00441992691212867,35.3223204546569));
#61267=CARTESIAN_POINT('',(-4.94405342481732,-0.00430212276008984,35.1776795453432));
#61268=CARTESIAN_POINT('',(-4.942,-6.05220448138622E-16,16.));
#61269=CARTESIAN_POINT('Ctrl Pts',(-4.94325592752636,-0.00441992691212867,
35.3223204546569));
#61270=CARTESIAN_POINT('Ctrl Pts',(-4.93125773853651,1.29607520943411,35.2803989968764));
#61271=CARTESIAN_POINT('Ctrl Pts',(-4.40405811483643,2.60517623543917,35.2384775390958));
#61272=CARTESIAN_POINT('Ctrl Pts',(-3.48340604301779,3.51702727807467,35.1965560813153));
#61273=CARTESIAN_POINT('Ctrl Pts',(-2.32120548652017,4.66811770803537,35.1436358272333));
#61274=CARTESIAN_POINT('Ctrl Pts',(-0.53201099429802,5.18616256481328,35.0907155731514));
#61275=CARTESIAN_POINT('Ctrl Pts',(1.06541470817911,4.83409661000376,35.0377953190694));
#61276=CARTESIAN_POINT('Ctrl Pts',(2.66284041065621,4.48203065519423,34.9848750649874));
#61277=CARTESIAN_POINT('Ctrl Pts',(4.0684973233883,3.25985388879729,34.9319548109055));
#61278=CARTESIAN_POINT('Ctrl Pts',(4.63913537493446,1.72685306505386,34.8790345568235));
#61279=CARTESIAN_POINT('Ctrl Pts',(5.20977342648062,0.193852241310417,34.8261143027416));
#61280=CARTESIAN_POINT('Ctrl Pts',(4.94539261684082,-1.64997263977952,34.7731940486596));
#61281=CARTESIAN_POINT('Ctrl Pts',(3.96697764231472,-2.96085915244703,34.7202737945776));
#61282=CARTESIAN_POINT('Ctrl Pts',(2.98856266778862,-4.27174566511454,34.6673535404957));
#61283=CARTESIAN_POINT('Ctrl Pts',(1.29611352837622,-5.04969380935962,34.6144332864137));
#61284=CARTESIAN_POINT('Ctrl Pts',(-0.335879201461312,-4.93870263300798,
34.5615130323317));
#61285=CARTESIAN_POINT('Ctrl Pts',(-1.96787193129885,-4.82771145665634,
34.5085927782498));
#61286=CARTESIAN_POINT('Ctrl Pts',(-3.53940825156152,-3.82778095970798,
34.4556725241678));
#61287=CARTESIAN_POINT('Ctrl Pts',(-4.33132914049615,-2.39649460920384,
34.4027522700858));
#61288=CARTESIAN_POINT('Ctrl Pts',(-4.73253428635246,-1.67137236904084,
34.3759416649429));
#61289=CARTESIAN_POINT('Ctrl Pts',(-4.93363817440523,-0.835535479848384,
34.3491310597999));
#61290=CARTESIAN_POINT('Ctrl Pts',(-4.93390856647989,0.000179243442527399,
34.3223204546569));
#61291=CARTESIAN_POINT('Ctrl Pts',(-4.93391474235666,-0.000255694835337854,
34.1776795453433));
#61292=CARTESIAN_POINT('Ctrl Pts',(-4.93428825140812,-0.80945462617062,
34.2036395758242));
#61293=CARTESIAN_POINT('Ctrl Pts',(-4.7463640914517,-1.61849015480256,34.2295996063052));
#61294=CARTESIAN_POINT('Ctrl Pts',(-4.36919376142154,-2.32674560401052,
34.2555596367863));
#61295=CARTESIAN_POINT('Ctrl Pts',(-3.60032140928848,-3.77054430657554,
34.3084798908682));
#61296=CARTESIAN_POINT('Ctrl Pts',(-2.04501820224325,-4.79554159303451,
34.3614001449502));
#61297=CARTESIAN_POINT('Ctrl Pts',(-0.415014641507274,-4.93268305062891,
34.4143203990321));
#61298=CARTESIAN_POINT('Ctrl Pts',(1.21498891922872,-5.0698245082233,34.4672406531141));
#61299=CARTESIAN_POINT('Ctrl Pts',(2.91969283365546,-4.31911013695313,34.5201609071961));
#61300=CARTESIAN_POINT('Ctrl Pts',(3.91899855510175,-3.02407829854611,34.573081161278));
#61301=CARTESIAN_POINT('Ctrl Pts',(4.91830427654803,-1.72904646013911,34.62600141536));
#61302=CARTESIAN_POINT('Ctrl Pts',(5.21221180501386,0.110302845404735,34.678921669442));
#61303=CARTESIAN_POINT('Ctrl Pts',(4.66622456671209,1.65225528404048,34.7318419235239));
#61304=CARTESIAN_POINT('Ctrl Pts',(4.12023732841032,3.19420772267622,34.7847621776059));
#61305=CARTESIAN_POINT('Ctrl Pts',(2.73435532334095,4.43876329440389,34.8376824316879));
#61306=CARTESIAN_POINT('Ctrl Pts',(1.14277932318225,4.81639436187842,34.8906026857698));
#61307=CARTESIAN_POINT('Ctrl Pts',(-0.448796676976434,5.19402542935295,
34.9435229398518));
#61308=CARTESIAN_POINT('Ctrl Pts',(-2.24606667222443,4.70473199257438,34.9964431939337));
#61309=CARTESIAN_POINT('Ctrl Pts',(-3.42657246357288,3.57242220104389,35.0493634480157));
#61310=CARTESIAN_POINT('Ctrl Pts',(-4.38069925079363,2.65724913586347,35.0921354804582));
#61311=CARTESIAN_POINT('Ctrl Pts',(-4.93192805452064,1.32202900724285,35.1349075129007));
#61312=CARTESIAN_POINT('Ctrl Pts',(-4.94405342481732,-0.00430212276008983,
35.1776795453432));
#61313=CARTESIAN_POINT('Origin',(0.,0.,16.));
#61314=CARTESIAN_POINT('',(-4.94842418382236,0.0025848059749288,36.3223204546569));
#61315=CARTESIAN_POINT('',(-4.9478484900732,0.00296101277178129,36.1776795453433));
#61316=CARTESIAN_POINT('',(-4.942,-6.05220448138622E-16,16.));
#61317=CARTESIAN_POINT('Ctrl Pts',(-4.94842418382236,0.0025848059749288,
36.3223204546569));
#61318=CARTESIAN_POINT('Ctrl Pts',(-4.94937063025513,0.151489796715591,
36.3175074421168));
#61319=CARTESIAN_POINT('Ctrl Pts',(-4.94323189211144,0.300315679824302,
36.3126944295766));
#61320=CARTESIAN_POINT('Ctrl Pts',(-4.92975351682066,0.448473855033485,
36.3078814170365));
#61321=CARTESIAN_POINT('Ctrl Pts',(-4.78155547265312,2.07750935224505,36.2549611629546));
#61322=CARTESIAN_POINT('Ctrl Pts',(-3.74602889959972,3.62582202129232,36.2020409088726));
#61323=CARTESIAN_POINT('Ctrl Pts',(-2.2970465727752,4.38488033790615,36.1491206547906));
#61324=CARTESIAN_POINT('Ctrl Pts',(-0.848064245950652,5.14393865451998,
36.0962004007087));
#61325=CARTESIAN_POINT('Ctrl Pts',(1.01437383464502,5.11374261870034,36.0432801466267));
#61326=CARTESIAN_POINT('Ctrl Pts',(2.43798755887529,4.30811039761326,35.9903598925447));
#61327=CARTESIAN_POINT('Ctrl Pts',(3.86160128310556,3.50247817652618,35.9374396384628));
#61328=CARTESIAN_POINT('Ctrl Pts',(4.84639065097043,1.92140977017166,35.8845193843808));
#61329=CARTESIAN_POINT('Ctrl Pts',(4.94170100734347,0.28842622847917,35.8315991302989));
#61330=CARTESIAN_POINT('Ctrl Pts',(5.03701136371651,-1.34455731321331,35.7786788762169));
#61331=CARTESIAN_POINT('Ctrl Pts',(4.24284270859772,-3.02945599024377,35.7257586221349));
#61332=CARTESIAN_POINT('Ctrl Pts',(2.92261874766819,-3.99523443505293,35.6728383680529));
#61333=CARTESIAN_POINT('Ctrl Pts',(1.60239478673866,-4.96101287986208,35.619918113971));
#61334=CARTESIAN_POINT('Ctrl Pts',(-0.243884480001596,-5.20767109244996,
35.566997859889));
#61335=CARTESIAN_POINT('Ctrl Pts',(-1.77133346242501,-4.62233450759977,
35.5140776058071));
#61336=CARTESIAN_POINT('Ctrl Pts',(-3.29878244484848,-4.03699792274956,
35.4611573517251));
#61337=CARTESIAN_POINT('Ctrl Pts',(-4.50740114295507,-2.61966654046123,
35.4082370976431));
#61338=CARTESIAN_POINT('Ctrl Pts',(-4.84410718162179,-1.01893284774532,
35.3553168435612));
#61339=CARTESIAN_POINT('Ctrl Pts',(-4.91408721473011,-0.686240873293583,
35.3443180472597));
#61340=CARTESIAN_POINT('Ctrl Pts',(-4.94640385328257,-0.345626598935659,
35.3333192509583));
#61341=CARTESIAN_POINT('Ctrl Pts',(-4.94325592752636,-0.00441992691212867,
35.3223204546569));
#61342=CARTESIAN_POINT('Ctrl Pts',(-4.94405342481732,-0.00430212276008983,
35.1776795453432));
#61343=CARTESIAN_POINT('Ctrl Pts',(-4.94693032680687,-0.318991453753773,
35.1878277669827));
#61344=CARTESIAN_POINT('Ctrl Pts',(-4.91945907962359,-0.633180389759553,
35.1979759886221));
#61345=CARTESIAN_POINT('Ctrl Pts',(-4.85982046564743,-0.941139879242983,
35.2081242102616));
#61346=CARTESIAN_POINT('Ctrl Pts',(-4.54882108892463,-2.5470660217169,35.2610444643436));
#61347=CARTESIAN_POINT('Ctrl Pts',(-3.36308074803015,-3.98359216038229,
35.3139647184255));
#61348=CARTESIAN_POINT('Ctrl Pts',(-1.84521233241245,-4.59334199455474,
35.3668849725075));
#61349=CARTESIAN_POINT('Ctrl Pts',(-0.327343916794751,-5.2030918287272,
35.4198052265894));
#61350=CARTESIAN_POINT('Ctrl Pts',(1.52265257354617,-4.98606535840671,35.4727254806714));
#61351=CARTESIAN_POINT('Ctrl Pts',(2.858190490191,-4.04157721099188,35.5256457347534));
#61352=CARTESIAN_POINT('Ctrl Pts',(4.19372840683581,-3.09708906357705,35.5785659888353));
#61353=CARTESIAN_POINT('Ctrl Pts',(5.01480774978454,-1.42513923906789,35.6314862429173));
#61354=CARTESIAN_POINT('Ctrl Pts',(4.94569007160633,0.20916248765404,35.6844064969993));
#61355=CARTESIAN_POINT('Ctrl Pts',(4.87657239342812,1.843464214376,35.7373267510812));
#61356=CARTESIAN_POINT('Ctrl Pts',(3.91725769412294,3.44011784331073,35.7902470051632));
#61357=CARTESIAN_POINT('Ctrl Pts',(2.50674303141734,4.26847028864764,35.8431672592451));
#61358=CARTESIAN_POINT('Ctrl Pts',(1.09622836871175,5.09682273398456,35.8960875133271));
#61359=CARTESIAN_POINT('Ctrl Pts',(-0.765486257394255,5.15687399572365,
35.9490077674091));
#61360=CARTESIAN_POINT('Ctrl Pts',(-2.2264518005877,4.42114369934827,36.001928021491));
#61361=CARTESIAN_POINT('Ctrl Pts',(-3.68741734378115,3.68541340297289,36.054848275573));
#61362=CARTESIAN_POINT('Ctrl Pts',(-4.74763380406204,2.15390154848305,36.107768529655));
#61363=CARTESIAN_POINT('Ctrl Pts',(-4.92192993683911,0.527451350812649,
36.1606887837369));
#61364=CARTESIAN_POINT('Ctrl Pts',(-4.94058331188609,0.353386757129483,
36.166352370939));
#61365=CARTESIAN_POINT('Ctrl Pts',(-4.94908977224877,0.178234784323597,
36.1720159581411));
#61366=CARTESIAN_POINT('Ctrl Pts',(-4.9478484900732,0.00296101277178129,
36.1776795453433));
#61367=CARTESIAN_POINT('Origin',(0.,0.,16.));
#61368=CARTESIAN_POINT('',(-4.93549302535697,0.00277814199197368,37.3223204546569));
#61369=CARTESIAN_POINT('',(-4.9350718820976,0.00242042316235142,37.1776795453432));
#61370=CARTESIAN_POINT('',(-4.942,-6.05220448138622E-16,16.));
#61371=CARTESIAN_POINT('Ctrl Pts',(-4.93549302535697,0.00277814199197368,
37.3223204546569));
#61372=CARTESIAN_POINT('Ctrl Pts',(-4.93877741300468,0.645159704289348,
37.3016956332752));
#61373=CARTESIAN_POINT('Ctrl Pts',(-4.82236482292357,1.2863972760676,37.2810708118936));
#61374=CARTESIAN_POINT('Ctrl Pts',(-4.5807162353096,1.87633613908203,37.2604459905119));
#61375=CARTESIAN_POINT('Ctrl Pts',(-3.96068154902433,3.39003237653315,37.2075257364299));
#61376=CARTESIAN_POINT('Ctrl Pts',(-2.51614312549289,4.56599842518147,37.1546054823479));
#61377=CARTESIAN_POINT('Ctrl Pts',(-0.908143809323614,4.86609426099016,
37.101685228266));
#61378=CARTESIAN_POINT('Ctrl Pts',(0.699855506845637,5.16619009679885,37.048764974184));
#61379=CARTESIAN_POINT('Ctrl Pts',(2.47131571565271,4.59041571976794,36.995844720102));
#61380=CARTESIAN_POINT('Ctrl Pts',(3.59558957056917,3.40225427845545,36.9429244660201));
#61381=CARTESIAN_POINT('Ctrl Pts',(4.71986342548563,2.21409283714297,36.8900042119381));
#61382=CARTESIAN_POINT('Ctrl Pts',(5.19695092651147,0.413544331548897,36.8370839578562));
#61383=CARTESIAN_POINT('Ctrl Pts',(4.80852954676355,-1.17543274293179,36.7841637037742));
#61384=CARTESIAN_POINT('Ctrl Pts',(4.42010816701563,-2.76440981741246,36.7312434496922));
#61385=CARTESIAN_POINT('Ctrl Pts',(3.16617790649396,-4.14181546077975,36.6783231956103));
#61386=CARTESIAN_POINT('Ctrl Pts',(1.6205564033125,-4.67732781392721,36.6254029415283));
#61387=CARTESIAN_POINT('Ctrl Pts',(0.0749349001310295,-5.21284016707467,
36.5724826874463));
#61388=CARTESIAN_POINT('Ctrl Pts',(-1.76237784571023,-4.90645923000227,
36.5195624333644));
#61389=CARTESIAN_POINT('Ctrl Pts',(-3.05059946099004,-3.89838959877812,
36.4666421792824));
#61390=CARTESIAN_POINT('Ctrl Pts',(-4.22165937898849,-2.98200228957926,
36.4185349377406));
#61391=CARTESIAN_POINT('Ctrl Pts',(-4.93896421945116,-1.48575712054711,
36.3704276961987));
#61392=CARTESIAN_POINT('Ctrl Pts',(-4.94842418382236,0.0025848059749288,
36.3223204546569));
#61393=CARTESIAN_POINT('Ctrl Pts',(-4.9478484900732,0.00296101277178129,
36.1776795453433));
#61394=CARTESIAN_POINT('Ctrl Pts',(-4.93749129838862,-1.4595139062905,36.2249362122231));
#61395=CARTESIAN_POINT('Ctrl Pts',(-4.24848225306339,-2.93046862920176,
36.2721928791029));
#61396=CARTESIAN_POINT('Ctrl Pts',(-3.11270745258791,-3.84898058519796,
36.3194495459828));
#61397=CARTESIAN_POINT('Ctrl Pts',(-1.84081303028634,-4.87757378268728,
36.3723698000648));
#61398=CARTESIAN_POINT('Ctrl Pts',(-0.00864838040995825,-5.21337163681495,
36.4252900541467));
#61399=CARTESIAN_POINT('Ctrl Pts',(1.54535997115889,-4.70270792099264,36.4782103082287));
#61400=CARTESIAN_POINT('Ctrl Pts',(3.09936832272773,-4.19204420517033,36.5311305623107));
#61401=CARTESIAN_POINT('Ctrl Pts',(4.37522037598902,-2.83491891939801,36.5840508163926));
#61402=CARTESIAN_POINT('Ctrl Pts',(4.78906674566614,-1.25237332141095,36.6369710704746));
#61403=CARTESIAN_POINT('Ctrl Pts',(5.20291311534324,0.330172276576089,36.6898913245566));
#61404=CARTESIAN_POINT('Ctrl Pts',(4.75475380143625,2.13813818677785,36.7428115786385));
#61405=CARTESIAN_POINT('Ctrl Pts',(3.64967335059123,3.34417159616718,36.7957318327205));
#61406=CARTESIAN_POINT('Ctrl Pts',(2.54459289974621,4.55020500555648,36.8486520868024));
#61407=CARTESIAN_POINT('Ctrl Pts',(0.782591311963154,5.15430591413334,36.9015723408844));
#61408=CARTESIAN_POINT('Ctrl Pts',(-0.830012575668756,4.88002851988171,
36.9544925949664));
#61409=CARTESIAN_POINT('Ctrl Pts',(-2.44261646330071,4.60575112563006,37.0074128490484));
#61410=CARTESIAN_POINT('Ctrl Pts',(-3.9058226507815,3.45309542854993,37.0603331031303));
#61411=CARTESIAN_POINT('Ctrl Pts',(-4.5500456396125,1.94953427978849,37.1132533572123));
#61412=CARTESIAN_POINT('Ctrl Pts',(-4.81147567364344,1.33937902438292,37.1347287532559));
#61413=CARTESIAN_POINT('Ctrl Pts',(-4.93803628002896,0.671436970049187,
37.1562041492996));
#61414=CARTESIAN_POINT('Ctrl Pts',(-4.9350718820976,0.00242042316235142,
37.1776795453432));
#61415=CARTESIAN_POINT('Origin',(0.,0.,16.));
#61416=CARTESIAN_POINT('',(-4.93830712716952,-0.00410043205665789,38.3223204546569));
#61417=CARTESIAN_POINT('',(-4.93901314208066,-0.00426717980477184,38.1776795453432));
#61418=CARTESIAN_POINT('',(-4.942,-6.05220448138622E-16,16.));
#61419=CARTESIAN_POINT('Ctrl Pts',(-4.93830712716952,-0.00410043205665789,
38.3223204546569));
#61420=CARTESIAN_POINT('Ctrl Pts',(-4.92941979674321,1.12913042651997,38.2858838244337));
#61421=CARTESIAN_POINT('Ctrl Pts',(-4.54190399082784,2.26785272885638,38.2494471942104));
#61422=CARTESIAN_POINT('Ctrl Pts',(-3.8277718834972,3.13875149433059,38.2130105639872));
#61423=CARTESIAN_POINT('Ctrl Pts',(-2.79057244061549,4.40363750783395,38.1600903099052));
#61424=CARTESIAN_POINT('Ctrl Pts',(-1.06439510407127,5.10356550944081,38.1071700558233));
#61425=CARTESIAN_POINT('Ctrl Pts',(0.560835013546147,4.91823775582626,38.0542498017413));
#61426=CARTESIAN_POINT('Ctrl Pts',(2.18606513116352,4.73291000221171,38.0013295476593));
#61427=CARTESIAN_POINT('Ctrl Pts',(3.71034802985413,3.66232649337579,37.9484092935774));
#61428=CARTESIAN_POINT('Ctrl Pts',(4.43614857526344,2.19640259366137,37.8954890394954));
#61429=CARTESIAN_POINT('Ctrl Pts',(5.16194912067276,0.730478693946923,37.8425687854135));
#61430=CARTESIAN_POINT('Ctrl Pts',(5.08926731280079,-1.13078559664599,37.7896485313315));
#61431=CARTESIAN_POINT('Ctrl Pts',(4.25136345697712,-2.53564731221314,37.7367282772495));
#61432=CARTESIAN_POINT('Ctrl Pts',(3.41345960115345,-3.94050902778028,37.6838080231676));
#61433=CARTESIAN_POINT('Ctrl Pts',(1.81033369737808,-4.88896816832161,37.6308877690856));
#61434=CARTESIAN_POINT('Ctrl Pts',(0.175600643277768,-4.9469953455946,37.5779675150036));
#61435=CARTESIAN_POINT('Ctrl Pts',(-1.45913241082256,-5.00502252286759,
37.5250472609217));
#61436=CARTESIAN_POINT('Ctrl Pts',(-3.12547261524786,-4.17261773687219,
37.4721270068397));
#61437=CARTESIAN_POINT('Ctrl Pts',(-4.06087724294093,-2.83070213074755,
37.4192067527577));
#61438=CARTESIAN_POINT('Ctrl Pts',(-4.63172289977408,-2.01177663806308,
37.3869113200575));
#61439=CARTESIAN_POINT('Ctrl Pts',(-4.93035015801884,-1.00309677586341,
37.3546158873572));
#61440=CARTESIAN_POINT('Ctrl Pts',(-4.93549302535697,0.00277814199197368,
37.3223204546569));
#61441=CARTESIAN_POINT('Ctrl Pts',(-4.9350718820976,0.00242042316235142,
37.1776795453432));
#61442=CARTESIAN_POINT('Ctrl Pts',(-4.93073133015009,-0.977171771522589,
37.2091244033815));
#61443=CARTESIAN_POINT('Ctrl Pts',(-4.64869419974499,-1.95906763650772,
37.2405692614198));
#61444=CARTESIAN_POINT('Ctrl Pts',(-4.10573795122914,-2.76523328246712,
37.2720141194581));
#61445=CARTESIAN_POINT('Ctrl Pts',(-3.19196748383364,-4.12197309551857,
37.3249343735401));
#61446=CARTESIAN_POINT('Ctrl Pts',(-1.53918675886144,-4.9809861211788,37.3778546276221));
#61447=CARTESIAN_POINT('Ctrl Pts',(0.0962665215178138,-4.94917487945839,
37.4307748817041));
#61448=CARTESIAN_POINT('Ctrl Pts',(1.73171980189707,-4.91736363773799,37.483695135786));
#61449=CARTESIAN_POINT('Ctrl Pts',(3.34984563768341,-3.99472812863699,37.536615389868));
#61450=CARTESIAN_POINT('Ctrl Pts',(4.21016493327244,-2.60348045225429,37.5895356439499));
#61451=CARTESIAN_POINT('Ctrl Pts',(5.07048422886148,-1.21223277587156,37.6424558980319));
#61452=CARTESIAN_POINT('Ctrl Pts',(5.17299698425316,0.64762706779285,37.6953761521139));
#61453=CARTESIAN_POINT('Ctrl Pts',(4.47079179693381,2.12499880919883,37.7482964061958));
#61454=CARTESIAN_POINT('Ctrl Pts',(3.76858660961448,3.60237055060479,37.8012166602778));
#61455=CARTESIAN_POINT('Ctrl Pts',(2.26166347958414,4.69725418975229,37.8541369143597));
#61456=CARTESIAN_POINT('Ctrl Pts',(0.639613445927835,4.90861425153937,37.9070571684417));
#61457=CARTESIAN_POINT('Ctrl Pts',(-0.982436587728495,5.11997431332645,
37.9599774225237));
#61458=CARTESIAN_POINT('Ctrl Pts',(-2.71961352501084,4.44781079775303,38.0128976766056));
#61459=CARTESIAN_POINT('Ctrl Pts',(-3.77695866803847,3.19971599529649,38.0658179306876));
#61460=CARTESIAN_POINT('Ctrl Pts',(-4.52195594113156,2.32031797609409,38.1031051355728));
#61461=CARTESIAN_POINT('Ctrl Pts',(-4.92945048540112,1.15499867080211,38.140392340458));
#61462=CARTESIAN_POINT('Ctrl Pts',(-4.93901314208066,-0.00426717980477184,
38.1776795453432));
#61463=CARTESIAN_POINT('Origin',(0.,0.,16.));
#61464=CARTESIAN_POINT('',(-4.95007301157197,-0.000387401246429997,39.3223204546569));
#61465=CARTESIAN_POINT('',(-4.95010830192917,0.000103228088722096,39.1776795453432));
#61466=CARTESIAN_POINT('',(-4.942,-6.05220448138622E-16,16.));
#61467=CARTESIAN_POINT('Ctrl Pts',(-4.95007301157197,-0.000387401246429997,
39.3223204546569));
#61468=CARTESIAN_POINT('Ctrl Pts',(-4.94825412650634,1.61464285750734,39.2700720155921));
#61469=CARTESIAN_POINT('Ctrl Pts',(-4.08291838964434,3.23134503628798,39.2178235765273));
#61470=CARTESIAN_POINT('Ctrl Pts',(-2.73731172677047,4.12440578092639,39.1655751374625));
#61471=CARTESIAN_POINT('Ctrl Pts',(-1.37440313527419,5.0289495790347,39.1126548833806));
#61472=CARTESIAN_POINT('Ctrl Pts',(0.481206517102607,5.19112301285789,39.0597346292986));
#61473=CARTESIAN_POINT('Ctrl Pts',(1.98036191326499,4.53671304225247,39.0068143752166));
#61474=CARTESIAN_POINT('Ctrl Pts',(3.47951730942733,3.88230307164706,38.9538941211347));
#61475=CARTESIAN_POINT('Ctrl Pts',(4.62221844937522,2.41130969661302,38.9009738670527));
#61476=CARTESIAN_POINT('Ctrl Pts',(4.88554783933805,0.796881951604831,38.8480536129708));
#61477=CARTESIAN_POINT('Ctrl Pts',(5.14887722930088,-0.817545793403355,
38.7951333588888));
#61478=CARTESIAN_POINT('Ctrl Pts',(4.53283486927871,-2.57540790838573,38.7422131048068));
#61479=CARTESIAN_POINT('Ctrl Pts',(3.31933115184711,-3.67227984222765,38.6892928507249));
#61480=CARTESIAN_POINT('Ctrl Pts',(2.10582743441549,-4.76915177606959,38.6363725966429));
#61481=CARTESIAN_POINT('Ctrl Pts',(0.294862359574459,-5.20503352877106,
38.5834523425609));
#61482=CARTESIAN_POINT('Ctrl Pts',(-1.28483879610452,-4.78045895320511,
38.530532088479));
#61483=CARTESIAN_POINT('Ctrl Pts',(-2.86453995178352,-4.35588437763916,
38.477611834397));
#61484=CARTESIAN_POINT('Ctrl Pts',(-4.21297718830044,-3.07085347380577,
38.424691580315));
#61485=CARTESIAN_POINT('Ctrl Pts',(-4.71308503194927,-1.51341600918913,
38.3717713262331));
#61486=CARTESIAN_POINT('Ctrl Pts',(-4.86885884155228,-1.02830470737132,
38.3552877023743));
#61487=CARTESIAN_POINT('Ctrl Pts',(-4.94232768041382,-0.516764503992941,
38.3388040785156));
#61488=CARTESIAN_POINT('Ctrl Pts',(-4.93830712716952,-0.00410043205665789,
38.3223204546569));
#61489=CARTESIAN_POINT('Ctrl Pts',(-4.93901314208066,-0.00426717980477184,
38.1776795453432));
#61490=CARTESIAN_POINT('Ctrl Pts',(-4.94302238554053,-0.490301467717737,
38.19331259454));
#61491=CARTESIAN_POINT('Ctrl Pts',(-4.87708344029753,-0.975271683602742,
38.2089456437367));
#61492=CARTESIAN_POINT('Ctrl Pts',(-4.7367428403112,-1.43766007643938,38.2245786929335));
#61493=CARTESIAN_POINT('Ctrl Pts',(-4.26166852078334,-3.00291525637914,
38.2774989470154));
#61494=CARTESIAN_POINT('Ctrl Pts',(-2.9340065329546,-4.30939952691902,38.3304192010974));
#61495=CARTESIAN_POINT('Ctrl Pts',(-1.36131527943717,-4.75924573231914,
38.3833394551794));
#61496=CARTESIAN_POINT('Ctrl Pts',(0.211375974080253,-5.20909193771926,
38.4362597092614));
#61497=CARTESIAN_POINT('Ctrl Pts',(2.0290964932864,-4.80230007797962,38.4891799633433));
#61498=CARTESIAN_POINT('Ctrl Pts',(3.2600296070944,-3.72502432092665,38.5421002174252));
#61499=CARTESIAN_POINT('Ctrl Pts',(4.4909627209024,-2.64774856387368,38.5950204715072));
#61500=CARTESIAN_POINT('Ctrl Pts',(5.13510842931226,-0.899988909507443,
38.6479407255892));
#61501=CARTESIAN_POINT('Ctrl Pts',(4.89769581831224,0.718453131327276,38.7008609796712));
#61502=CARTESIAN_POINT('Ctrl Pts',(4.66028320731222,2.33689517216197,38.7537812337531));
#61503=CARTESIAN_POINT('Ctrl Pts',(3.54131227690224,3.82601959946517,38.8067014878351));
#61504=CARTESIAN_POINT('Ctrl Pts',(2.05284121454405,4.50438033235388,38.859621741917));
#61505=CARTESIAN_POINT('Ctrl Pts',(0.564370152185806,5.18274106524261,38.912541995999));
#61506=CARTESIAN_POINT('Ctrl Pts',(-1.29360104212064,5.05033810371689,38.965462250081));
#61507=CARTESIAN_POINT('Ctrl Pts',(-2.67083637362622,4.16776106512145,39.0183825041629));
#61508=CARTESIAN_POINT('Ctrl Pts',(-4.04807170513178,3.28518402652602,39.0713027582449));
#61509=CARTESIAN_POINT('Ctrl Pts',(-4.94457117383642,1.65243291086087,39.1242230123269));
#61510=CARTESIAN_POINT('Ctrl Pts',(-4.95008293089447,0.0166795651704946,
39.1771432664088));
#61511=CARTESIAN_POINT('Ctrl Pts',(-4.95010154909182,0.0111541440981086,
39.1773220260536));
#61512=CARTESIAN_POINT('Ctrl Pts',(-4.95011000089745,0.00562868876953041,
39.1775007856984));
#61513=CARTESIAN_POINT('Ctrl Pts',(-4.95010830192917,0.000103228088722096,
39.1776795453432));
#61514=CARTESIAN_POINT('Origin',(0.,0.,16.));
#61515=CARTESIAN_POINT('',(-4.93943724668283,0.00434520414469897,40.3223204546569));
#61516=CARTESIAN_POINT('',(-4.9387122051873,0.0042019715207839,40.1776795453432));
#61517=CARTESIAN_POINT('',(-4.942,-6.05220448138622E-16,16.));
#61518=CARTESIAN_POINT('Ctrl Pts',(-4.93943724668283,0.00434520414469897,
40.3223204546569));
#61519=CARTESIAN_POINT('Ctrl Pts',(-4.94341650816428,0.474947915493244,
40.3071804608325));
#61520=CARTESIAN_POINT('Ctrl Pts',(-4.88164614501736,0.944527111103383,
40.2920404670082));
#61521=CARTESIAN_POINT('Ctrl Pts',(-4.74989944410437,1.39357590613184,40.2769004731838));
#61522=CARTESIAN_POINT('Ctrl Pts',(-4.28939272477215,2.96317868165193,40.2239802191018));
#61523=CARTESIAN_POINT('Ctrl Pts',(-2.97393022079225,4.28194545604953,40.1710599650198));
#61524=CARTESIAN_POINT('Ctrl Pts',(-1.40548766464857,4.74638841223249,40.1181397109379));
#61525=CARTESIAN_POINT('Ctrl Pts',(0.162954891495088,5.21083136841545,40.0652194568559));
#61526=CARTESIAN_POINT('Ctrl Pts',(1.98437749980252,4.82095050638379,40.012299202774));
#61527=CARTESIAN_POINT('Ctrl Pts',(3.22526935667327,3.75516126313619,39.959378948692));
#61528=CARTESIAN_POINT('Ctrl Pts',(4.46616121354403,2.68937201988858,39.90645869461));
#61529=CARTESIAN_POINT('Ctrl Pts',(5.1265223189781,0.947674395425016,39.8535384405281));
#61530=CARTESIAN_POINT('Ctrl Pts',(4.90416134563252,-0.672904176876648,
39.8006181864461));
#61531=CARTESIAN_POINT('Ctrl Pts',(4.68180037228695,-2.29348274917834,39.7476979323641));
#61532=CARTESIAN_POINT('Ctrl Pts',(3.57671732016171,-3.79294226931812,39.6947776782822));
#61533=CARTESIAN_POINT('Ctrl Pts',(2.09461507151,-4.4851071600863,39.6418574242002));
#61534=CARTESIAN_POINT('Ctrl Pts',(0.612512822858338,-5.17727205085446,
39.5889371701182));
#61535=CARTESIAN_POINT('Ctrl Pts',(-1.24660862231976,-5.06214231225107,
39.5360169160363));
#61536=CARTESIAN_POINT('Ctrl Pts',(-2.63198689690885,-4.19240307100288,
39.4830966619543));
#61537=CARTESIAN_POINT('Ctrl Pts',(-4.01736517149795,-3.32266382975467,
39.4301764078723));
#61538=CARTESIAN_POINT('Ctrl Pts',(-4.92900027549801,-1.69831508586162,
39.3772561537904));
#61539=CARTESIAN_POINT('Ctrl Pts',(-4.9497140621902,-0.0626836327184169,
39.3243358997084));
#61540=CARTESIAN_POINT('Ctrl Pts',(-4.94997702073422,-0.0419195265770804,
39.3236640846913));
#61541=CARTESIAN_POINT('Ctrl Pts',(-4.95009639895585,-0.0211536021213772,
39.3229922696741));
#61542=CARTESIAN_POINT('Ctrl Pts',(-4.95007301157197,-0.000387401246429997,
39.3223204546569));
#61543=CARTESIAN_POINT('Ctrl Pts',(-4.95010830192917,0.000103228088722096,
39.1776795453432));
#61544=CARTESIAN_POINT('Ctrl Pts',(-4.94960703596349,-1.6301363826534,39.2304210397804));
#61545=CARTESIAN_POINT('Ctrl Pts',(-4.06548675829959,-3.26084190194751,
39.2831625342175));
#61546=CARTESIAN_POINT('Ctrl Pts',(-2.6988623875562,-4.14966758230844,39.3359040286547));
#61547=CARTESIAN_POINT('Ctrl Pts',(-1.32760604174843,-5.04150580838138,
39.3888242827367));
#61548=CARTESIAN_POINT('Ctrl Pts',(0.529430695278565,-5.18642668481171,
39.4417445368187));
#61549=CARTESIAN_POINT('Ctrl Pts',(2.02243945069843,-4.51811220521201,39.4946647909006));
#61550=CARTESIAN_POINT('Ctrl Pts',(3.51544820611836,-3.84979772561229,39.5475850449826));
#61551=CARTESIAN_POINT('Ctrl Pts',(4.6444289799311,-2.36824788998248,39.6005052990645));
#61552=CARTESIAN_POINT('Ctrl Pts',(4.89274292745657,-0.751442530371268,
39.6534255531465));
#61553=CARTESIAN_POINT('Ctrl Pts',(5.14105687498204,0.865362829239897,39.7063458072285));
#61554=CARTESIAN_POINT('Ctrl Pts',(4.50870399622024,2.61742371283248,39.7592660613104));
#61555=CARTESIAN_POINT('Ctrl Pts',(3.2850586262277,3.70297030137619,39.8121863153924));
#61556=CARTESIAN_POINT('Ctrl Pts',(2.06141325623513,4.78851688991993,39.8651065694743));
#61557=CARTESIAN_POINT('Ctrl Pts',(0.246475395011777,5.2075491834148,39.9180268235563));
#61558=CARTESIAN_POINT('Ctrl Pts',(-1.32921167314713,4.76831160460351,39.9709470776383));
#61559=CARTESIAN_POINT('Ctrl Pts',(-2.90489874130597,4.32907402579225,40.0238673317202));
#61560=CARTESIAN_POINT('Ctrl Pts',(-4.24133501640037,3.03156657467491,40.0767875858022));
#61561=CARTESIAN_POINT('Ctrl Pts',(-4.72694684795839,1.46954847732333,40.1297078398842));
#61562=CARTESIAN_POINT('Ctrl Pts',(-4.87368101212714,0.997563642860038,
40.1456984083705));
#61563=CARTESIAN_POINT('Ctrl Pts',(-4.94273254556439,0.501428253000672,
40.1616889768569));
#61564=CARTESIAN_POINT('Ctrl Pts',(-4.9387122051873,0.0042019715207839,
40.1776795453432));
#61565=CARTESIAN_POINT('Origin',(0.,0.,16.));
#61566=CARTESIAN_POINT('',(-4.93485552516168,-0.00220275864159403,41.3223204546569));
#61567=CARTESIAN_POINT('',(-4.93524162710697,-0.00257366327817901,41.1776795453432));
#61568=CARTESIAN_POINT('',(-4.942,-6.05220448138622E-16,16.));
#61569=CARTESIAN_POINT('Ctrl Pts',(-4.93485552516168,-0.00220275864159403,
41.3223204546569));
#61570=CARTESIAN_POINT('Ctrl Pts',(-4.93097721826847,0.962135133190097,
41.291368651991));
#61571=CARTESIAN_POINT('Ctrl Pts',(-4.65830472720369,1.92849849558568,41.2604168493251));
#61572=CARTESIAN_POINT('Ctrl Pts',(-4.13125993704044,2.72695615437044,41.2294650466591));
#61573=CARTESIAN_POINT('Ctrl Pts',(-3.23013813457067,4.09212969959618,41.1765447925771));
#61574=CARTESIAN_POINT('Ctrl Pts',(-1.58541225739997,4.96646613003761,41.1236245384952));
#61575=CARTESIAN_POINT('Ctrl Pts',(0.0502660136753988,4.94985574164777,
41.0707042844132));
#61576=CARTESIAN_POINT('Ctrl Pts',(1.68594428475072,4.93324535325794,41.0177840303312));
#61577=CARTESIAN_POINT('Ctrl Pts',(3.31257494973071,4.0256881460368,40.9648637762493));
#61578=CARTESIAN_POINT('Ctrl Pts',(4.18578697328013,2.64249615885673,40.9119435221673));
#61579=CARTESIAN_POINT('Ctrl Pts',(5.05899899682956,1.25930417167664,40.8590232680854));
#61580=CARTESIAN_POINT('Ctrl Pts',(5.17879237894847,-0.599522595462416,
40.8061030140034));
#61581=CARTESIAN_POINT('Ctrl Pts',(4.49034783841098,-2.08335662461616,40.7531827599214));
#61582=CARTESIAN_POINT('Ctrl Pts',(3.8019032978735,-3.56719065376989,40.7002625058395));
#61583=CARTESIAN_POINT('Ctrl Pts',(2.30522083467963,-4.67603194493831,40.6473422517575));
#61584=CARTESIAN_POINT('Ctrl Pts',(0.685205202367444,-4.90245778828362,
40.5944219976755));
#61585=CARTESIAN_POINT('Ctrl Pts',(-0.93481042994472,-5.12888363162893,
40.5415017435936));
#61586=CARTESIAN_POINT('Ctrl Pts',(-2.6781592313752,-4.47289402715115,40.4885814895116));
#61587=CARTESIAN_POINT('Ctrl Pts',(-3.74705816474816,-3.23467983659099,
40.4356612354296));
#61588=CARTESIAN_POINT('Ctrl Pts',(-4.51015502798955,-2.35070724073872,
40.397880975172));
#61589=CARTESIAN_POINT('Ctrl Pts',(-4.92950741869571,-1.16999430476845,
40.3601007149145));
#61590=CARTESIAN_POINT('Ctrl Pts',(-4.93943724668283,0.00434520414469897,
40.3223204546569));
#61591=CARTESIAN_POINT('Ctrl Pts',(-4.9387122051873,0.0042019715207839,
40.1776795453432));
#61592=CARTESIAN_POINT('Ctrl Pts',(-4.92942736292292,-1.14412557296836,
40.2146092309388));
#61593=CARTESIAN_POINT('Ctrl Pts',(-4.53040370843391,-2.2982715368062,40.2515389165345));
#61594=CARTESIAN_POINT('Ctrl Pts',(-3.79843588104676,-3.17419030434592,
40.2884686021301));
#61595=CARTESIAN_POINT('Ctrl Pts',(-2.74952569455548,-4.42938224507769,
40.341388856212));
#61596=CARTESIAN_POINT('Ctrl Pts',(-1.01691793355136,-5.11323738295533,
40.394309110294));
#61597=CARTESIAN_POINT('Ctrl Pts',(0.606519628933596,-4.91281316257247,
40.4472293643759));
#61598=CARTESIAN_POINT('Ctrl Pts',(2.22995719141853,-4.71238894218962,40.5001496184579));
#61599=CARTESIAN_POINT('Ctrl Pts',(3.74422455538428,-3.62768536354625,40.5530698725399));
#61600=CARTESIAN_POINT('Ctrl Pts',(4.45636984813063,-2.15507935058069,40.6059901266218));
#61601=CARTESIAN_POINT('Ctrl Pts',(5.16851514087698,-0.682473337615157,
40.6589103807038));
#61602=CARTESIAN_POINT('Ctrl Pts',(5.07853836240398,1.17803510967258,40.7118306347858));
#61603=CARTESIAN_POINT('Ctrl Pts',(4.22761426072911,2.57504891081838,40.7647508888677));
#61604=CARTESIAN_POINT('Ctrl Pts',(3.37669015905424,3.97206271196421,40.8176711429497));
#61605=CARTESIAN_POINT('Ctrl Pts',(1.76481873417747,4.90558186696812,40.8705913970317));
#61606=CARTESIAN_POINT('Ctrl Pts',(0.12961696774931,4.94841375314338,40.9235116511136));
#61607=CARTESIAN_POINT('Ctrl Pts',(-1.50558479867887,4.99124563931864,40.9764319051956));
#61608=CARTESIAN_POINT('Ctrl Pts',(-3.16411690665841,4.14339025666527,41.0293521592775));
#61609=CARTESIAN_POINT('Ctrl Pts',(-4.0870097333165,2.79283917732535,41.0822724133595));
#61610=CARTESIAN_POINT('Ctrl Pts',(-4.6416213166461,1.98122676595515,41.1140747906874));
#61611=CARTESIAN_POINT('Ctrl Pts',(-4.93056429073029,0.988070940573039,
41.1458771680153));
#61612=CARTESIAN_POINT('Ctrl Pts',(-4.93524162710697,-0.00257366327817901,
41.1776795453432));
#61613=CARTESIAN_POINT('Origin',(0.,0.,16.));
#61614=CARTESIAN_POINT('',(-4.94748713622925,-0.00316321289392352,42.3223204546569));
#61615=CARTESIAN_POINT('',(-4.94809820533655,-0.00280696805152256,42.1776795453432));
#61616=CARTESIAN_POINT('',(-4.942,-6.05220448138622E-16,16.));
#61617=CARTESIAN_POINT('Ctrl Pts',(-4.94748713622925,-0.00316321289392352,
42.3223204546569));
#61618=CARTESIAN_POINT('Ctrl Pts',(-4.93670139323051,1.44433029491444,42.2755568431494));
#61619=CARTESIAN_POINT('Ctrl Pts',(-4.26377312667576,2.9005508041267,42.2287932316419));
#61620=CARTESIAN_POINT('Ctrl Pts',(-3.14834440585587,3.81988560527279,42.1820296201344));
#61621=CARTESIAN_POINT('Ctrl Pts',(-1.88606441050834,4.8602550227471,42.1291093660525));
#61622=CARTESIAN_POINT('Ctrl Pts',(-0.0570997319322858,5.21306603328002,
42.0761891119705));
#61623=CARTESIAN_POINT('Ctrl Pts',(1.50158745972911,4.71686693007535,42.0232688578886));
#61624=CARTESIAN_POINT('Ctrl Pts',(3.06027465139055,4.22066782687068,41.9703486038066));
#61625=CARTESIAN_POINT('Ctrl Pts',(4.34868435613734,2.87545860992836,41.9174283497246));
#61626=CARTESIAN_POINT('Ctrl Pts',(4.77722061558389,1.29682756189652,41.8645080956427));
#61627=CARTESIAN_POINT('Ctrl Pts',(5.20575687503042,-0.281803486135251,
41.8115878415607));
#61628=CARTESIAN_POINT('Ctrl Pts',(4.77441968917683,-2.09385636525649,41.7586675874787));
#61629=CARTESIAN_POINT('Ctrl Pts',(3.68059554195264,-3.31010800304349,41.7057473333968));
#61630=CARTESIAN_POINT('Ctrl Pts',(2.58677139472839,-4.52635964083055,41.6528270793148));
#61631=CARTESIAN_POINT('Ctrl Pts',(0.830460286133465,-5.14681003728328,
41.5999068252328));
#61632=CARTESIAN_POINT('Ctrl Pts',(-0.78462299692839,-4.88753161503282,
41.5469865711509));
#61633=CARTESIAN_POINT('Ctrl Pts',(-2.39970627999022,-4.62825319278237,
41.4940663170689));
#61634=CARTESIAN_POINT('Ctrl Pts',(-3.87356173751901,-3.48924595182876,
41.4411460629869));
#61635=CARTESIAN_POINT('Ctrl Pts',(-4.531730602399,-1.99173700134697,41.388225808905));
#61636=CARTESIAN_POINT('Ctrl Pts',(-4.80495209353668,-1.37008555249385,
41.366257357489));
#61637=CARTESIAN_POINT('Ctrl Pts',(-4.93760820478682,-0.686654334984092,
41.3442889060729));
#61638=CARTESIAN_POINT('Ctrl Pts',(-4.93485552516168,-0.00220275864159403,
41.3223204546569));
#61639=CARTESIAN_POINT('Ctrl Pts',(-4.93524162710697,-0.00257366327817901,
41.1776795453432));
#61640=CARTESIAN_POINT('Ctrl Pts',(-4.93834753998013,-0.660395889443513,
41.1987974220973));
#61641=CARTESIAN_POINT('Ctrl Pts',(-4.81610883381463,-1.31711081291602,
41.2199152988513));
#61642=CARTESIAN_POINT('Ctrl Pts',(-4.56308028711322,-1.91882712196431,
41.2410331756054));
#61643=CARTESIAN_POINT('Ctrl Pts',(-3.92900446891528,-3.42669556588764,
41.2939534296874));
#61644=CARTESIAN_POINT('Ctrl Pts',(-2.47359928718284,-4.58918567770784,
41.3468736837693));
#61645=CARTESIAN_POINT('Ctrl Pts',(-0.862880381041693,-4.87432422789462,
41.3997939378513));
#61646=CARTESIAN_POINT('Ctrl Pts',(0.74783852509941,-5.15946277808138,41.4527141919333));
#61647=CARTESIAN_POINT('Ctrl Pts',(2.51387115564923,-4.56724976663472,41.5056344460152));
#61648=CARTESIAN_POINT('Ctrl Pts',(3.62705400678358,-3.36869091228363,41.5585547000972));
#61649=CARTESIAN_POINT('Ctrl Pts',(4.74023685791794,-2.17013205793252,41.6114749541791));
#61650=CARTESIAN_POINT('Ctrl Pts',(5.20056992963686,-0.36522736067698,41.6643952082611));
#61651=CARTESIAN_POINT('Ctrl Pts',(4.79739777779339,1.22007122425299,41.7173154623431));
#61652=CARTESIAN_POINT('Ctrl Pts',(4.3942256259499,2.80536980918301,41.770235716425));
#61653=CARTESIAN_POINT('Ctrl Pts',(3.12754825054399,4.17106228178741,41.823155970507));
#61654=CARTESIAN_POINT('Ctrl Pts',(1.57701656414349,4.69218690879255,41.8760762245889));
#61655=CARTESIAN_POINT('Ctrl Pts',(0.0264848777430365,5.21331153579767,
41.9289964786709));
#61656=CARTESIAN_POINT('Ctrl Pts',(-1.80790111965202,4.88986831720356,41.9819167327529));
#61657=CARTESIAN_POINT('Ctrl Pts',(-3.08669837960869,3.86986980968975,42.0348369868349));
#61658=CARTESIAN_POINT('Ctrl Pts',(-4.2372765819408,2.95214181174547,42.0824511730043));
#61659=CARTESIAN_POINT('Ctrl Pts',(-4.93809323584742,1.47053667915491,42.1300653591738));
#61660=CARTESIAN_POINT('Ctrl Pts',(-4.94809820533655,-0.00280696805152256,
42.1776795453432));
#61661=CARTESIAN_POINT('Origin',(0.,0.,16.));
#61662=CARTESIAN_POINT('',(-4.94451025515232,0.00421302333877771,43.3223204546569));
#61663=CARTESIAN_POINT('',(-4.94371934458518,0.00435719887056521,43.1776795453432));
#61664=CARTESIAN_POINT('',(-4.942,-6.05220448138622E-16,16.));
#61665=CARTESIAN_POINT('Ctrl Pts',(-4.94451025515232,0.00421302333877771,
43.3223204546569));
#61666=CARTESIAN_POINT('Ctrl Pts',(-4.94721961825891,0.30354166338666,43.3126652883898));
#61667=CARTESIAN_POINT('Ctrl Pts',(-4.9223727794906,0.602421473877891,43.3030101221227));
#61668=CARTESIAN_POINT('Ctrl Pts',(-4.8683572221906,0.895933308008362,43.2933549558557));
#61669=CARTESIAN_POINT('Ctrl Pts',(-4.57229634269635,2.50468041899365,43.2404347017737));
#61670=CARTESIAN_POINT('Ctrl Pts',(-3.39995792978838,3.95216446044364,43.1875144476917));
#61671=CARTESIAN_POINT('Ctrl Pts',(-1.88782194598489,4.57599462800297,43.1345941936098));
#61672=CARTESIAN_POINT('Ctrl Pts',(-0.375685962181428,5.19982479556229,
43.0816739395278));
#61673=CARTESIAN_POINT('Ctrl Pts',(1.47624759251752,5.00000108923096,43.0287536854458));
#61674=CARTESIAN_POINT('Ctrl Pts',(2.82050563945827,4.06796588887349,42.9758334313639));
#61675=CARTESIAN_POINT('Ctrl Pts',(4.16476368639908,3.13593068851599,42.9229131772819));
#61676=CARTESIAN_POINT('Ctrl Pts',(5.00134622558163,1.47168399413228,42.8699929231999));
#61677=CARTESIAN_POINT('Ctrl Pts',(4.9474203102028,-0.163189489389038,42.817072669118));
#61678=CARTESIAN_POINT('Ctrl Pts',(4.89349439482397,-1.79806297291028,42.764152415036));
#61679=CARTESIAN_POINT('Ctrl Pts',(3.94906002488378,-3.40356324556919,42.7112321609541));
#61680=CARTESIAN_POINT('Ctrl Pts',(2.54630479212863,-4.24498886227479,42.6583119068721));
#61681=CARTESIAN_POINT('Ctrl Pts',(1.14354955937346,-5.0864144789804,42.6053916527901));
#61682=CARTESIAN_POINT('Ctrl Pts',(-0.717526536196703,-5.16376543973274,
42.5524713987082));
#61683=CARTESIAN_POINT('Ctrl Pts',(-2.18526664959422,-4.44164476353361,
42.4995511446262));
#61684=CARTESIAN_POINT('Ctrl Pts',(-3.65300676299177,-3.71952408733446,
42.4466308905442));
#61685=CARTESIAN_POINT('Ctrl Pts',(-4.72741089421663,-2.19793177418379,
42.3937106364623));
#61686=CARTESIAN_POINT('Ctrl Pts',(-4.91681530376954,-0.573171705400564,
42.3407903823803));
#61687=CARTESIAN_POINT('Ctrl Pts',(-4.93885025563959,-0.38415018261489,
42.3346337398059));
#61688=CARTESIAN_POINT('Ctrl Pts',(-4.94890712844976,-0.19373232997381,
42.3284770972314));
#61689=CARTESIAN_POINT('Ctrl Pts',(-4.94748713622925,-0.00316321289392352,
42.3223204546569));
#61690=CARTESIAN_POINT('Ctrl Pts',(-4.94809820533655,-0.00280696805152256,
42.1776795453432));
#61691=CARTESIAN_POINT('Ctrl Pts',(-4.94921314716046,-0.166994620502292,
42.1829856132557));
#61692=CARTESIAN_POINT('Ctrl Pts',(-4.94174917029318,-0.331079676814377,
42.1882916811682));
#61693=CARTESIAN_POINT('Ctrl Pts',(-4.92537268191333,-0.494270345953525,
42.1935977490807));
#61694=CARTESIAN_POINT('Ctrl Pts',(-4.76204120174297,-2.12185819764955,
42.2465180031627));
#61695=CARTESIAN_POINT('Ctrl Pts',(-3.71216971888389,-3.6604801046081,42.2994382572447));
#61696=CARTESIAN_POINT('Ctrl Pts',(-2.25619545826342,-4.40603918329588,
42.3523585113266));
#61697=CARTESIAN_POINT('Ctrl Pts',(-0.800221197642949,-5.15159826198366,
42.4052787654086));
#61698=CARTESIAN_POINT('Ctrl Pts',(1.06185584073894,-5.10409451240069,42.4581990194906));
#61699=CARTESIAN_POINT('Ctrl Pts',(2.4779207651768,-4.28526637586659,42.5111192735725));
#61700=CARTESIAN_POINT('Ctrl Pts',(3.89398568961467,-3.46643823933247,42.5640395276545));
#61701=CARTESIAN_POINT('Ctrl Pts',(4.8640385001085,-1.87628571584728,42.6169597817364));
#61702=CARTESIAN_POINT('Ctrl Pts',(4.9441682152519,-0.242486886078373,42.6698800358184));
#61703=CARTESIAN_POINT('Ctrl Pts',(5.02429793039529,1.39131194369048,42.7228002899004));
#61704=CARTESIAN_POINT('Ctrl Pts',(4.21450455018825,3.06875707974299,42.7757205439823));
#61705=CARTESIAN_POINT('Ctrl Pts',(2.88536189314395,4.02222400870711,42.8286407980643));
#61706=CARTESIAN_POINT('Ctrl Pts',(1.55621923609964,4.97569093767124,42.8815610521463));
#61707=CARTESIAN_POINT('Ctrl Pts',(-0.292272697781964,5.20517965954696,
42.9344813062282));
#61708=CARTESIAN_POINT('Ctrl Pts',(-1.81421576809595,4.60567263029181,42.9874015603102));
#61709=CARTESIAN_POINT('Ctrl Pts',(-3.33615883840994,4.00616560103666,43.0403218143921));
#61710=CARTESIAN_POINT('Ctrl Pts',(-4.53155304515633,2.57766282065063,43.0932420684741));
#61711=CARTESIAN_POINT('Ctrl Pts',(-4.85336774243223,0.97386897853116,43.1461623225561));
#61712=CARTESIAN_POINT('Ctrl Pts',(-4.91725446964838,0.655483458634976,
43.1566680634851));
#61713=CARTESIAN_POINT('Ctrl Pts',(-4.94671318283581,0.330189668722103,
43.1671738044142));
#61714=CARTESIAN_POINT('Ctrl Pts',(-4.94371934458518,0.00435719887056521,
43.1776795453432));
#61715=CARTESIAN_POINT('Origin',(0.,0.,16.));
#61716=CARTESIAN_POINT('',(-4.93394997286128,0.000507016503537849,44.3223204546569));
#61717=CARTESIAN_POINT('',(-4.93390371744476,7.29331094537614E-5,44.1776795453432));
#61718=CARTESIAN_POINT('',(-4.942,-6.05220448138622E-16,16.));
#61719=CARTESIAN_POINT('Ctrl Pts',(-4.93394997286128,0.000507016503537849,
44.3223204546569));
#61720=CARTESIAN_POINT('Ctrl Pts',(-4.93467682586532,0.794322762801275,
44.2968534795483));
#61721=CARTESIAN_POINT('Ctrl Pts',(-4.75416264908751,1.58782655048687,44.2713865044396));
#61722=CARTESIAN_POINT('Ctrl Pts',(-4.39062917456631,2.28603892939324,44.245919529331));
#61723=CARTESIAN_POINT('Ctrl Pts',(-3.63520833024163,3.73692095748179,44.192999275249));
#61724=CARTESIAN_POINT('Ctrl Pts',(-2.08949837449215,4.77632854708712,44.1400790211671));
#61725=CARTESIAN_POINT('Ctrl Pts',(-0.460839790231528,4.92861291064672,
44.0871587670851));
#61726=CARTESIAN_POINT('Ctrl Pts',(1.16781879402907,5.08089727420631,44.0342385130031));
#61727=CARTESIAN_POINT('Ctrl Pts',(2.8794260068008,4.3460584117202,43.9813182589212));
#61728=CARTESIAN_POINT('Ctrl Pts',(3.8907242466578,3.06036980963467,43.9283980048392));
#61729=CARTESIAN_POINT('Ctrl Pts',(4.90202248651478,1.77468120754915,43.8754777507573));
#61730=CARTESIAN_POINT('Ctrl Pts',(5.21301175345704,-0.0618571341358118,
43.8225574966753));
#61731=CARTESIAN_POINT('Ctrl Pts',(4.68137860928635,-1.60881722136807,43.7696372425933));
#61732=CARTESIAN_POINT('Ctrl Pts',(4.14974546511566,-3.15577730860032,43.7167169885114));
#61733=CARTESIAN_POINT('Ctrl Pts',(2.77548990983206,-4.41315914137991,43.6637967344294));
#61734=CARTESIAN_POINT('Ctrl Pts',(1.18749227412456,-4.80556558941283,43.6108764803475));
#61735=CARTESIAN_POINT('Ctrl Pts',(-0.400505361582988,-5.19797203744577,
43.5579562262655));
#61736=CARTESIAN_POINT('Ctrl Pts',(-2.20224507771443,-4.72540310073197,
43.5050359721835));
#61737=CARTESIAN_POINT('Ctrl Pts',(-3.3932232627399,-3.60411354211475,43.4521157181016));
#61738=CARTESIAN_POINT('Ctrl Pts',(-4.36691049562677,-2.68740042232609,
43.4088506302867));
#61739=CARTESIAN_POINT('Ctrl Pts',(-4.93236951831919,-1.33708753420181,
43.3655855424718));
#61740=CARTESIAN_POINT('Ctrl Pts',(-4.94451025515232,0.00421302333877771,
43.3223204546569));
#61741=CARTESIAN_POINT('Ctrl Pts',(-4.94371934458518,0.00435719887056521,
43.1776795453432));
#61742=CARTESIAN_POINT('Ctrl Pts',(-4.93163241109647,-1.31111647133373,
43.2200940584961));
#61743=CARTESIAN_POINT('Ctrl Pts',(-4.39058351177215,-2.63537038181765,
43.262508571649));
#61744=CARTESIAN_POINT('Ctrl Pts',(-3.45056931084653,-3.5492493095965,43.3049230848019));
#61745=CARTESIAN_POINT('Ctrl Pts',(-2.27772099417954,-4.68948885175174,
43.3578433388839));
#61746=CARTESIAN_POINT('Ctrl Pts',(-0.483789173040172,-5.19088303220938,
43.4107635929659));
#61747=CARTESIAN_POINT('Ctrl Pts',(1.11029555303778,-4.82398621634968,43.4636838470478));
#61748=CARTESIAN_POINT('Ctrl Pts',(2.70438027911579,-4.45708940048996,43.5166041011298));
#61749=CARTESIAN_POINT('Ctrl Pts',(4.09861791013234,-3.22190158831284,43.5695243552118));
#61750=CARTESIAN_POINT('Ctrl Pts',(4.65498401236277,-1.68366358732205,43.6224446092938));
#61751=CARTESIAN_POINT('Ctrl Pts',(5.21135011459319,-0.145425586331283,
43.6753648633757));
#61752=CARTESIAN_POINT('Ctrl Pts',(4.92984468803749,1.69586260347318,43.7282851174576));
#61753=CARTESIAN_POINT('Ctrl Pts',(3.93928891523517,2.99759938499667,43.7812053715396));
#61754=CARTESIAN_POINT('Ctrl Pts',(2.94873314243287,4.29933616652015,43.8341256256216));
#61755=CARTESIAN_POINT('Ctrl Pts',(1.24912702338399,5.06152153976273,43.8870458797035));
#61756=CARTESIAN_POINT('Ctrl Pts',(-0.381763724262289,4.93536783730094,
43.9399661337855));
#61757=CARTESIAN_POINT('Ctrl Pts',(-2.01265447190855,4.80921413483915,43.9928863878675));
#61758=CARTESIAN_POINT('Ctrl Pts',(-3.57482984815219,3.79472135667302,44.0458066419495));
#61759=CARTESIAN_POINT('Ctrl Pts',(-4.35341454219008,2.35613689213404,44.0987268960314));
#61760=CARTESIAN_POINT('Ctrl Pts',(-4.74060923336151,1.6407204811301,44.125044445802));
#61761=CARTESIAN_POINT('Ctrl Pts',(-4.93401170909488,0.820420654182907,
44.1513619955726));
#61762=CARTESIAN_POINT('Ctrl Pts',(-4.93390371744476,7.29331094537614E-5,
44.1776795453432));
#61763=CARTESIAN_POINT('Origin',(0.,0.,16.));
#61764=CARTESIAN_POINT('',(-4.94264971735337,-0.00447858357024544,45.3223204546569));
#61765=CARTESIAN_POINT('',(-4.94345166054126,-0.00439535110808767,45.1776795453432));
#61766=CARTESIAN_POINT('',(-4.942,-6.05220448138622E-16,16.));
#61767=CARTESIAN_POINT('Ctrl Pts',(-4.94264971735337,-0.00447858357024544,
45.3223204546569));
#61768=CARTESIAN_POINT('Ctrl Pts',(-4.93082575729553,1.27648252745284,45.2810416707067));
#61769=CARTESIAN_POINT('Ctrl Pts',(-4.42134998955586,2.56578412734584,45.2397628867565));
#61770=CARTESIAN_POINT('Ctrl Pts',(-3.52575508348954,3.47457186233093,45.1984841028063));
#61771=CARTESIAN_POINT('Ctrl Pts',(-2.37758390575486,4.63965651937944,45.1455638487244));
#61772=CARTESIAN_POINT('Ctrl Pts',(-0.594796197848898,5.17933734465609,
45.0926435946425));
#61773=CARTESIAN_POINT('Ctrl Pts',(1.00677715711088,4.84664815013159,45.0397233405605));
#61774=CARTESIAN_POINT('Ctrl Pts',(2.60835051207067,4.51395895560708,44.9868030864785));
#61775=CARTESIAN_POINT('Ctrl Pts',(4.02870951408424,3.30889974128137,44.9338828323965));
#61776=CARTESIAN_POINT('Ctrl Pts',(4.61787619111481,1.78292400813641,44.8809625783145));
#61777=CARTESIAN_POINT('Ctrl Pts',(5.20704286814536,0.25694827499149,44.8280423242326));
#61778=CARTESIAN_POINT('Ctrl Pts',(4.96501722019298,-1.58994397697268,44.7751220701506));
#61779=CARTESIAN_POINT('Ctrl Pts',(4.00255388014552,-2.91258664622809,44.7222018160687));
#61780=CARTESIAN_POINT('Ctrl Pts',(3.04009054009802,-4.23522931548356,44.6692815619867));
#61781=CARTESIAN_POINT('Ctrl Pts',(1.35718950795542,-5.03362240203022,44.6163613079047));
#61782=CARTESIAN_POINT('Ctrl Pts',(-0.276028001533181,-4.94240903584718,
44.5634410538228));
#61783=CARTESIAN_POINT('Ctrl Pts',(-1.90924551102172,-4.85119566966413,
44.5105207997408));
#61784=CARTESIAN_POINT('Ctrl Pts',(-3.49277949785625,-3.8703758507514,44.4576005456588));
#61785=CARTESIAN_POINT('Ctrl Pts',(-4.30198062482356,-2.4487877080092,44.4046802915769));
#61786=CARTESIAN_POINT('Ctrl Pts',(-4.72176742799645,-1.71131475847591,
44.3772270126036));
#61787=CARTESIAN_POINT('Ctrl Pts',(-4.93316642875337,-0.85522261151742,
44.3497737336302));
#61788=CARTESIAN_POINT('Ctrl Pts',(-4.93394997286128,0.000507016503537849,
44.3223204546569));
#61789=CARTESIAN_POINT('Ctrl Pts',(-4.93390371744476,7.29331094537614E-5,
44.1776795453432));
#61790=CARTESIAN_POINT('Ctrl Pts',(-4.93379455568915,-0.829163376745596,
44.2042822496546));
#61791=CARTESIAN_POINT('Ctrl Pts',(-4.73595877931974,-1.65844862422957,
44.2308849539659));
#61792=CARTESIAN_POINT('Ctrl Pts',(-4.34068739432695,-2.37950250585247,
44.2574876582773));
#61793=CARTESIAN_POINT('Ctrl Pts',(-3.55438154059382,-3.813881288388,44.3104079123592));
#61794=CARTESIAN_POINT('Ctrl Pts',(-1.98677582129545,-4.81996270254719,
44.3633281664412));
#61795=CARTESIAN_POINT('Ctrl Pts',(-0.355230555152893,-4.9373485276323,
44.4162484205232));
#61796=CARTESIAN_POINT('Ctrl Pts',(1.27631471098969,-5.05473435271742,44.4691686746052));
#61797=CARTESIAN_POINT('Ctrl Pts',(2.97179952397649,-4.28342458872844,44.5220889286871));
#61798=CARTESIAN_POINT('Ctrl Pts',(3.95534413875573,-2.9763823636485,44.5750091827691));
#61799=CARTESIAN_POINT('Ctrl Pts',(4.93888875353493,-1.66934013856861,44.627929436851));
#61800=CARTESIAN_POINT('Ctrl Pts',(5.21049317010665,0.173434547602146,44.680849690933));
#61801=CARTESIAN_POINT('Ctrl Pts',(4.64586705931524,1.70865985432931,44.733769945015));
#61802=CARTESIAN_POINT('Ctrl Pts',(4.08124094852381,3.24388516105654,44.7866901990969));
#61803=CARTESIAN_POINT('Ctrl Pts',(2.68038431036912,4.47156108834011,44.8396104531789));
#61804=CARTESIAN_POINT('Ctrl Pts',(1.08435053733238,4.82988438193028,44.8925307072609));
#61805=CARTESIAN_POINT('Ctrl Pts',(-0.511683235704347,5.18820767552046,
44.9454509613428));
#61806=CARTESIAN_POINT('Ctrl Pts',(-2.30289414362315,4.67717833541725,44.9983712154248));
#61807=CARTESIAN_POINT('Ctrl Pts',(-3.46959671833554,3.53065119244912,45.0512914695067));
#61808=CARTESIAN_POINT('Ctrl Pts',(-4.39839859233384,2.61791080594467,45.0934208281189));
#61809=CARTESIAN_POINT('Ctrl Pts',(-4.93141112790613,1.30241637823199,45.1355501867311));
#61810=CARTESIAN_POINT('Ctrl Pts',(-4.94345166054126,-0.00439535110808767,
45.1776795453432));
#61811=CARTESIAN_POINT('Origin',(0.,0.,16.));
#61812=CARTESIAN_POINT('',(-4.94881445934699,0.00227942523971326,46.3223204546569));
#61813=CARTESIAN_POINT('',(-4.94828946219151,0.00267981890309541,46.1776795453432));
#61814=CARTESIAN_POINT('',(-4.942,-6.05220448138622E-16,16.));
#61815=CARTESIAN_POINT('Ctrl Pts',(-4.94881445934699,0.00227942523971326,
46.3223204546569));
#61816=CARTESIAN_POINT('Ctrl Pts',(-4.94955378308614,0.131274482234953,
46.3181501159471));
#61817=CARTESIAN_POINT('Ctrl Pts',(-4.94494719039334,0.260215895992481,
46.3139797772374));
#61818=CARTESIAN_POINT('Ctrl Pts',(-4.93482452766902,0.388722801454193,
46.3098094385276));
#61819=CARTESIAN_POINT('Ctrl Pts',(-4.80637120034064,2.01943401260374,46.2568891844456));
#61820=CARTESIAN_POINT('Ctrl Pts',(-3.78967659005442,3.58017725671765,46.2039689303636));
#61821=CARTESIAN_POINT('Ctrl Pts',(-2.34999567814797,4.35673258852779,46.1510486762817));
#61822=CARTESIAN_POINT('Ctrl Pts',(-0.910314766241556,5.13328792033792,
46.0981284221997));
#61823=CARTESIAN_POINT('Ctrl Pts',(0.952352447285067,5.12565533984434,46.0452081681177));
#61824=CARTESIAN_POINT('Ctrl Pts',(2.38562099756669,4.33732763245101,45.9922879140358));
#61825=CARTESIAN_POINT('Ctrl Pts',(3.81888954784836,3.54899992505766,45.9393676599538));
#61826=CARTESIAN_POINT('Ctrl Pts',(4.82275943488501,1.97997709076453,45.8864474058719));
#61827=CARTESIAN_POINT('Ctrl Pts',(4.93784446656618,0.348267941757418,45.8335271517899));
#61828=CARTESIAN_POINT('Ctrl Pts',(5.05292949824735,-1.28344120724965,45.7806068977079));
#61829=CARTESIAN_POINT('Ctrl Pts',(4.27922967457309,-2.97783667097068,45.727686643626));
#61830=CARTESIAN_POINT('Ctrl Pts',(2.97080185134115,-3.95953720721528,45.674766389544));
#61831=CARTESIAN_POINT('Ctrl Pts',(1.66237402810921,-4.94123774345989,45.621846135462));
#61832=CARTESIAN_POINT('Ctrl Pts',(-0.18078179468041,-5.21024335222807,
45.5689258813801));
#61833=CARTESIAN_POINT('Ctrl Pts',(-1.71520936255536,-4.64345295850584,
45.5160056272981));
#61834=CARTESIAN_POINT('Ctrl Pts',(-3.24963693043034,-4.0766625647836,45.4630853732162));
#61835=CARTESIAN_POINT('Ctrl Pts',(-4.47533624339064,-2.67407616857091,
45.4101651191342));
#61836=CARTESIAN_POINT('Ctrl Pts',(-4.8314085760891,-1.07753872605438,45.3572448650522));
#61837=CARTESIAN_POINT('Ctrl Pts',(-4.90973785658425,-0.726330228027688,
45.3456033949204));
#61838=CARTESIAN_POINT('Ctrl Pts',(-4.94598431844091,-0.365736088925451,
45.3339619247887));
#61839=CARTESIAN_POINT('Ctrl Pts',(-4.94264971735337,-0.00447858357024544,
45.3223204546569));
#61840=CARTESIAN_POINT('Ctrl Pts',(-4.94345166054126,-0.00439535110808767,
45.1776795453432));
#61841=CARTESIAN_POINT('Ctrl Pts',(-4.94653568871891,-0.339118433408757,
45.188470440813));
#61842=CARTESIAN_POINT('Ctrl Pts',(-4.91544069255685,-0.673271876348126,
45.1992613362828));
#61843=CARTESIAN_POINT('Ctrl Pts',(-4.848063077171,-0.999941813506336,45.2100522317526));
#61844=CARTESIAN_POINT('Ctrl Pts',(-4.51763261978812,-2.60198273066066,
45.2629724858346));
#61845=CARTESIAN_POINT('Ctrl Pts',(-3.31457746351644,-4.02403961913634,
45.3158927399166));
#61846=CARTESIAN_POINT('Ctrl Pts',(-1.78943402176491,-4.61535752812037,
45.3688129939985));
#61847=CARTESIAN_POINT('Ctrl Pts',(-0.264290580013278,-5.20667543710444,
45.4217332480805));
#61848=CARTESIAN_POINT('Ctrl Pts',(1.58294114721826,-4.96725436659668,45.4746535021624));
#61849=CARTESIAN_POINT('Ctrl Pts',(2.90693970933454,-4.00665705506737,45.5275737562444));
#61850=CARTESIAN_POINT('Ctrl Pts',(4.23093827145077,-3.0460597435381,45.5804940103263));
#61851=CARTESIAN_POINT('Ctrl Pts',(5.0317036684518,-1.36428619098739,45.6334142644083));
#61852=CARTESIAN_POINT('Ctrl Pts',(4.94279342482124,0.2690583397166,45.6863345184903));
#61853=CARTESIAN_POINT('Ctrl Pts',(4.85388318119067,1.90240287042061,45.7392547725723));
#61854=CARTESIAN_POINT('Ctrl Pts',(3.87529729692844,3.4873183792779,45.7921750266543));
#61855=CARTESIAN_POINT('Ctrl Pts',(2.45485161832049,4.29852332349801,45.8450952807362));
#61856=CARTESIAN_POINT('Ctrl Pts',(1.03440593971258,5.1097282677181,45.8980155348182));
#61857=CARTESIAN_POINT('Ctrl Pts',(-0.827899533241065,5.1472226473011,45.9509357889001));
#61858=CARTESIAN_POINT('Ctrl Pts',(-2.27984537368615,4.39384846150945,46.0038560429821));
#61859=CARTESIAN_POINT('Ctrl Pts',(-3.73179121413126,3.64047427571779,46.056776297064));
#61860=CARTESIAN_POINT('Ctrl Pts',(-4.77337742206781,2.0962315245515,46.109696551146));
#61861=CARTESIAN_POINT('Ctrl Pts',(-4.92795824091158,0.46778927569873,46.162616805228));
#61862=CARTESIAN_POINT('Ctrl Pts',(-4.94262440066108,0.31328760891278,46.1676377185997));
#61863=CARTESIAN_POINT('Ctrl Pts',(-4.94930605767903,0.158028008604056,
46.1726586319715));
#61864=CARTESIAN_POINT('Ctrl Pts',(-4.94828946219151,0.00267981890309541,
46.1776795453432));
#61865=CARTESIAN_POINT('Origin',(0.,0.,16.));
#61866=CARTESIAN_POINT('',(-4.9358501160701,0.00303175399314515,47.3223204546569));
#61867=CARTESIAN_POINT('',(-4.93538463697233,0.00269292579073279,47.1776795453432));
#61868=CARTESIAN_POINT('',(-4.942,-6.05220448138622E-16,16.));
#61869=CARTESIAN_POINT('Ctrl Pts',(-4.9358501160701,0.00303175399314515,
47.3223204546569));
#61870=CARTESIAN_POINT('Ctrl Pts',(-4.93933793021421,0.625283723714611,
47.3023383071056));
#61871=CARTESIAN_POINT('Ctrl Pts',(-4.83028758168748,1.24635811395051,47.2823561595543));
#61872=CARTESIAN_POINT('Ctrl Pts',(-4.60310972348256,1.82070849089976,47.2623740120029));
#61873=CARTESIAN_POINT('Ctrl Pts',(-4.00145717602152,3.34180464946569,47.2094537579209));
#61874=CARTESIAN_POINT('Ctrl Pts',(-2.57127018656423,4.53518329005682,47.156533503839));
#61875=CARTESIAN_POINT('Ctrl Pts',(-0.967024164301558,4.85473612062603,
47.103613249757));
#61876=CARTESIAN_POINT('Ctrl Pts',(0.637221857961163,5.17428895119525,47.050692995675));
#61877=CARTESIAN_POINT('Ctrl Pts',(2.41552691302929,4.62001597174252,46.9977727415931));
#61878=CARTESIAN_POINT('Ctrl Pts',(3.55411144818602,3.44556096290971,46.9448524875111));
#61879=CARTESIAN_POINT('Ctrl Pts',(4.69269598334273,2.27110595407693,46.8919322334292));
#61880=CARTESIAN_POINT('Ctrl Pts',(5.19155999858808,0.476468915864107,46.8390119793472));
#61881=CARTESIAN_POINT('Ctrl Pts',(4.82241570154595,-1.11709683409153,46.7860917252652));
#61882=CARTESIAN_POINT('Ctrl Pts',(4.45327140450381,-2.71066258404717,46.7331714711833));
#61883=CARTESIAN_POINT('Ctrl Pts',(3.21611879517418,-4.10315704574563,46.6802512171013));
#61884=CARTESIAN_POINT('Ctrl Pts',(1.67709780224552,-4.65735348636513,46.6273309630194));
#61885=CARTESIAN_POINT('Ctrl Pts',(0.138076809316829,-5.21154992698464,
46.5744107089374));
#61886=CARTESIAN_POINT('Ctrl Pts',(-1.7028125672109,-4.92744834652514,46.5214904548554));
#61887=CARTESIAN_POINT('Ctrl Pts',(-3.00315123328947,-3.93505796720279,
46.4685702007734));
#61888=CARTESIAN_POINT('Ctrl Pts',(-4.2010177406636,-3.02087212574391,46.4198202854013));
#61889=CARTESIAN_POINT('Ctrl Pts',(-4.94017200312835,-1.50563121453851,
46.3710703700291));
#61890=CARTESIAN_POINT('Ctrl Pts',(-4.94881445934699,0.00227942523971326,
46.3223204546569));
#61891=CARTESIAN_POINT('Ctrl Pts',(-4.94828946219151,0.00267981890309541,
46.1776795453432));
#61892=CARTESIAN_POINT('Ctrl Pts',(-4.93859117623925,-1.47933656262951,
46.2255788860534));
#61893=CARTESIAN_POINT('Ctrl Pts',(-4.22826766932132,-2.96941554830109,
46.2734782267636));
#61894=CARTESIAN_POINT('Ctrl Pts',(-3.06585319961028,-3.88640494404102,
46.3213775674738));
#61895=CARTESIAN_POINT('Ctrl Pts',(-1.78159190971431,-4.89951516838867,
46.3742978215558));
#61896=CARTESIAN_POINT('Ctrl Pts',(0.0545060998286173,-5.21309387054478,
46.4272180756378));
#61897=CARTESIAN_POINT('Ctrl Pts',(1.60221433767964,-4.68364264720964,46.4801383297198));
#61898=CARTESIAN_POINT('Ctrl Pts',(3.14992257553069,-4.15419142387448,46.5330585838017));
#61899=CARTESIAN_POINT('Ctrl Pts',(4.40924104168984,-2.78171027504809,46.5859788378836));
#61900=CARTESIAN_POINT('Ctrl Pts',(4.80388637285101,-1.19426753592463,46.6388990919656));
#61901=CARTESIAN_POINT('Ctrl Pts',(5.19853170401218,0.393175203198827,46.6918193460476));
#61902=CARTESIAN_POINT('Ctrl Pts',(4.72850390017529,2.19557953261941,46.7447396001296));
#61903=CARTESIAN_POINT('Ctrl Pts',(3.60889486296925,3.38813770361555,46.7976598542115));
#61904=CARTESIAN_POINT('Ctrl Pts',(2.48928582576321,4.58069587461169,46.8505801082935));
#61905=CARTESIAN_POINT('Ctrl Pts',(0.720095555188062,5.16340788718348,46.9035003623755));
#61906=CARTESIAN_POINT('Ctrl Pts',(-0.889067460630859,4.86961582479301,
46.9564206164574));
#61907=CARTESIAN_POINT('Ctrl Pts',(-2.49823047644978,4.57582376240254,47.0093408705394));
#61908=CARTESIAN_POINT('Ctrl Pts',(-3.9473662375124,3.40552762504981,47.0622611246213));
#61909=CARTESIAN_POINT('Ctrl Pts',(-4.57332808734244,1.89427279876787,47.1151813787033));
#61910=CARTESIAN_POINT('Ctrl Pts',(-4.81974582587867,1.29934836887573,47.1360141009166));
#61911=CARTESIAN_POINT('Ctrl Pts',(-4.93859613551441,0.651585501425685,
47.1568468231299));
#61912=CARTESIAN_POINT('Ctrl Pts',(-4.93538463697233,0.00269292579073279,
47.1776795453432));
#61913=CARTESIAN_POINT('Origin',(0.,0.,16.));
#61914=CARTESIAN_POINT('',(-4.93779824682792,-0.00394849367342132,48.3223204546569));
#61915=CARTESIAN_POINT('',(-4.93847649956811,-0.00414486738929824,48.1776795453433));
#61916=CARTESIAN_POINT('',(-4.942,-6.05220448138622E-16,16.));
#61917=CARTESIAN_POINT('Ctrl Pts',(-4.93779824682792,-0.00394849367342132,
48.3223204546569));
#61918=CARTESIAN_POINT('Ctrl Pts',(-4.92945107906705,1.10958389040538,48.286526498264));
#61919=CARTESIAN_POINT('Ctrl Pts',(-4.55663414200584,2.22817899674935,48.2507325418711));
#61920=CARTESIAN_POINT('Ctrl Pts',(-3.86551329136296,3.09215224876629,48.2149385854782));
#61921=CARTESIAN_POINT('Ctrl Pts',(-2.8437125545035,4.36950989861378,48.1620183313963));
#61922=CARTESIAN_POINT('Ctrl Pts',(-1.12614067807074,5.09029714456033,48.1090980773143));
#61923=CARTESIAN_POINT('Ctrl Pts',(0.50121521532169,4.92467073449426,48.0561778232323));
#61924=CARTESIAN_POINT('Ctrl Pts',(2.12857110871417,4.75904432442819,48.0032575691504));
#61925=CARTESIAN_POINT('Ctrl Pts',(3.66571101906626,3.70700425834946,47.9503373150684));
#61926=CARTESIAN_POINT('Ctrl Pts',(4.40921624712591,2.2499801379868,47.8974170609865));
#61927=CARTESIAN_POINT('Ctrl Pts',(5.15272147518552,0.792956017624232,47.8444968069045));
#61928=CARTESIAN_POINT('Ctrl Pts',(5.10259202095273,-1.06905215702231,47.7915765528226));
#61929=CARTESIAN_POINT('Ctrl Pts',(4.28176788829653,-2.4839610073443,47.7386562987406));
#61930=CARTESIAN_POINT('Ctrl Pts',(3.46094375564028,-3.89886985766637,47.6857360446586));
#61931=CARTESIAN_POINT('Ctrl Pts',(1.86942494456057,-4.86667938366393,47.6328157905766));
#61932=CARTESIAN_POINT('Ctrl Pts',(0.235514769794999,-4.94450516517706,
47.5798955364947));
#61933=CARTESIAN_POINT('Ctrl Pts',(-1.39839540497048,-5.02233094669018,
47.5269752824127));
#61934=CARTESIAN_POINT('Ctrl Pts',(-3.07469694342178,-4.21017298371899,
47.4740550283308));
#61935=CARTESIAN_POINT('Ctrl Pts',(-4.02628865991507,-2.87968716396305,
47.4211347742488));
#61936=CARTESIAN_POINT('Ctrl Pts',(-4.61856906134665,-2.05157920362054,
47.3881966677182));
#61937=CARTESIAN_POINT('Ctrl Pts',(-4.93010088448512,-1.0226738972605,47.3552585611876));
#61938=CARTESIAN_POINT('Ctrl Pts',(-4.9358501160701,0.00303175399314515,
47.3223204546569));
#61939=CARTESIAN_POINT('Ctrl Pts',(-4.93538463697233,0.00269292579073279,
47.1776795453432));
#61940=CARTESIAN_POINT('Ctrl Pts',(-4.93043813690577,-0.996761729574154,
47.2097670772119));
#61941=CARTESIAN_POINT('Ctrl Pts',(-4.63591709407219,-1.99889645937005,
47.2418546090805));
#61942=CARTESIAN_POINT('Ctrl Pts',(-4.07193915439288,-2.81476655400573,
47.2739421409492));
#61943=CARTESIAN_POINT('Ctrl Pts',(-3.1418004330159,-4.16033756528617,47.3268623950311));
#61944=CARTESIAN_POINT('Ctrl Pts',(-1.47873505166457,-4.99926607263594,
47.3797826491131));
#61945=CARTESIAN_POINT('Ctrl Pts',(0.156212871657996,-4.94764557838933,
47.4327029031951));
#61946=CARTESIAN_POINT('Ctrl Pts',(1.79116079498061,-4.89602508414272,47.4856231572771));
#61947=CARTESIAN_POINT('Ctrl Pts',(3.39799126027446,-3.95385558829969,47.538543411359));
#61948=CARTESIAN_POINT('Ctrl Pts',(4.24139410598325,-2.552288241629,47.591463665441));
#61949=CARTESIAN_POINT('Ctrl Pts',(5.08479695169201,-1.15072089495835,47.6443839195229));
#61950=CARTESIAN_POINT('Ctrl Pts',(5.16477217781576,0.710244302539926,47.6973041736049));
#61951=CARTESIAN_POINT('Ctrl Pts',(4.44472189944271,2.17900125452958,47.7502244276869));
#61952=CARTESIAN_POINT('Ctrl Pts',(3.72467162106964,3.64775820651928,47.8031446817689));
#61953=CARTESIAN_POINT('Ctrl Pts',(2.20459583819974,4.72430691300034,47.8560649358508));
#61954=CARTESIAN_POINT('Ctrl Pts',(0.580104444733958,4.91600224408279,47.9089851899327));
#61955=CARTESIAN_POINT('Ctrl Pts',(-1.04438694873177,5.10769757516524,47.9619054440147));
#61956=CARTESIAN_POINT('Ctrl Pts',(-2.77329395279337,4.41453953084916,48.0148256980967));
#61957=CARTESIAN_POINT('Ctrl Pts',(-3.81544231731622,3.15372781860764,48.0677459521787));
#61958=CARTESIAN_POINT('Ctrl Pts',(-4.53707600502276,2.28068110435693,48.1043904832335));
#61959=CARTESIAN_POINT('Ctrl Pts',(-4.92941962837742,1.13545330336185,48.1410350142884));
#61960=CARTESIAN_POINT('Ctrl Pts',(-4.93847649956811,-0.00414486738929824,
48.1776795453433));
#61961=CARTESIAN_POINT('Origin',(0.,0.,16.));
#61962=CARTESIAN_POINT('',(-4.94996872029631,-0.000754789231165454,49.3223204546569));
#61963=CARTESIAN_POINT('',(-4.95009281286112,-0.000267728824007536,49.1776795453432));
#61964=CARTESIAN_POINT('',(-4.942,-6.05220448138622E-16,16.));
#61965=CARTESIAN_POINT('Ctrl Pts',(-4.94996872029631,-0.000754789231165454,
49.3223204546569));
#61966=CARTESIAN_POINT('Ctrl Pts',(-4.94657205241788,1.59450047399929,49.2707146894224));
#61967=CARTESIAN_POINT('Ctrl Pts',(-4.10534559557285,3.19283284813315,49.219108924188));
#61968=CARTESIAN_POINT('Ctrl Pts',(-2.78707318578254,4.09094385103807,49.1675031589536));
#61969=CARTESIAN_POINT('Ctrl Pts',(-1.4352220784804,5.01193130760659,49.1145829048716));
#61970=CARTESIAN_POINT('Ctrl Pts',(0.418286878732396,5.19657136329379,49.0616626507896));
#61971=CARTESIAN_POINT('Ctrl Pts',(1.92525967895112,4.56036990866522,49.0087423967077));
#61972=CARTESIAN_POINT('Ctrl Pts',(3.4322324791698,3.92416845403667,48.9558221426257));
#61973=CARTESIAN_POINT('Ctrl Pts',(4.59266912239443,2.4671254890924,48.9029018885438));
#61974=CARTESIAN_POINT('Ctrl Pts',(4.87553607768602,0.856006127569342,48.8499816344618));
#61975=CARTESIAN_POINT('Ctrl Pts',(5.15840303297761,-0.755113233953766,
48.7970613803799));
#61976=CARTESIAN_POINT('Ctrl Pts',(4.56370030033613,-2.52030899205568,48.7441411262979));
#61977=CARTESIAN_POINT('Ctrl Pts',(3.36357293293406,-3.63180060852569,48.6912208722159));
#61978=CARTESIAN_POINT('Ctrl Pts',(2.16344556553202,-4.74329222499568,48.6383006181339));
#61979=CARTESIAN_POINT('Ctrl Pts',(0.357893563369426,-5.20107969983381,
48.585380364052));
#61980=CARTESIAN_POINT('Ctrl Pts',(-1.22683490171212,-4.79567249290391,
48.53246010997));
#61981=CARTESIAN_POINT('Ctrl Pts',(-2.81156336679367,-4.39026528597401,
48.4795398558881));
#61982=CARTESIAN_POINT('Ctrl Pts',(-4.17546829479417,-3.12166339727609,
48.4266196018061));
#61983=CARTESIAN_POINT('Ctrl Pts',(-4.69440596015137,-1.57039842605291,
48.3736993477241));
#61984=CARTESIAN_POINT('Ctrl Pts',(-4.86234697051046,-1.0683708724689,48.356573050035));
#61985=CARTESIAN_POINT('Ctrl Pts',(-4.94179210764521,-0.536739194059861,
48.339446752346));
#61986=CARTESIAN_POINT('Ctrl Pts',(-4.93779824682792,-0.00394849367342132,
48.3223204546569));
#61987=CARTESIAN_POINT('Ctrl Pts',(-4.93847649956811,-0.00414486738929824,
48.1776795453433));
#61988=CARTESIAN_POINT('Ctrl Pts',(-4.942499122392,-0.510299091646249,48.1939552683704));
#61989=CARTESIAN_POINT('Ctrl Pts',(-4.87091055869885,-1.01534275567644,
48.2102309913974));
#61990=CARTESIAN_POINT('Ctrl Pts',(-4.7189797263556,-1.49493463832769,48.2265067144245));
#61991=CARTESIAN_POINT('Ctrl Pts',(-4.224979045888,-3.05432000285457,48.2794269685065));
#61992=CARTESIAN_POINT('Ctrl Pts',(-2.88158795996869,-4.34462535174135,
48.3323472225885));
#61993=CARTESIAN_POINT('Ctrl Pts',(-1.30356274672183,-4.77538725089245,
48.3852674766704));
#61994=CARTESIAN_POINT('Ctrl Pts',(0.274462466525034,-5.20614915004355,
48.4381877307524));
#61995=CARTESIAN_POINT('Ctrl Pts',(2.08712180709941,-4.77736759945896,48.4911079848343));
#61996=CARTESIAN_POINT('Ctrl Pts',(3.30491467655429,-3.68525958533767,48.5440282389163));
#61997=CARTESIAN_POINT('Ctrl Pts',(4.5227075460092,-2.59315157121635,48.5969484929983));
#61998=CARTESIAN_POINT('Ctrl Pts',(5.14563394434455,-0.837717093558183,
48.6498687470803));
#61999=CARTESIAN_POINT('Ctrl Pts',(4.88863323791471,0.7777302204381,48.7027890011622));
#62000=CARTESIAN_POINT('Ctrl Pts',(4.63163253148487,2.39317753443434,48.7557092552442));
#62001=CARTESIAN_POINT('Ctrl Pts',(3.49470472029,3.86863768476876,48.8086295093261));
#62002=CARTESIAN_POINT('Ctrl Pts',(1.99812533468889,4.52891757238984,48.8615497634081));
#62003=CARTESIAN_POINT('Ctrl Pts',(0.501545949087793,5.18919746001092,48.91447001749));
#62004=CARTESIAN_POINT('Ctrl Pts',(-1.35468501091949,5.03429708491863,48.967390271572));
#62005=CARTESIAN_POINT('Ctrl Pts',(-2.7211279083772,4.13510122450199,49.020310525654));
#62006=CARTESIAN_POINT('Ctrl Pts',(-4.07559217393182,3.24378797391906,49.0727668655504));
#62007=CARTESIAN_POINT('Ctrl Pts',(-4.94881798417885,1.62117145762289,49.1252232054468));
#62008=CARTESIAN_POINT('Ctrl Pts',(-4.95009281286112,-0.000267728824007536,
49.1776795453432));
#62009=CARTESIAN_POINT('Origin',(0.,0.,16.));
#62010=CARTESIAN_POINT('',(-4.94000433004934,0.00442567287284368,50.3223204546569));
#62011=CARTESIAN_POINT('',(-4.93925722597112,0.00431400617654748,50.1776795453432));
#62012=CARTESIAN_POINT('',(-4.942,-6.05220448138622E-16,16.));
#62013=CARTESIAN_POINT('Ctrl Pts',(-4.94000433004934,0.00442567287284368,
50.3223204546569));
#62014=CARTESIAN_POINT('Ctrl Pts',(-4.94391985550658,0.454920647205931,
50.3078231346629));
#62015=CARTESIAN_POINT('Ctrl Pts',(-4.88736862134446,0.904450331901516,
50.2933258146688));
#62016=CARTESIAN_POINT('Ctrl Pts',(-4.76643244788693,1.33593422554585,50.2788284946748));
#62017=CARTESIAN_POINT('Ctrl Pts',(-4.3249734037525,2.91100032695947,50.2259082405929));
#62018=CARTESIAN_POINT('Ctrl Pts',(-3.02558272518919,4.24560561283798,50.1729879865109));
#62019=CARTESIAN_POINT('Ctrl Pts',(-1.46288143191014,4.72901432133872,50.120067732429));
#62020=CARTESIAN_POINT('Ctrl Pts',(0.0998198613689605,5.21242302983948,
50.067147478347));
#62021=CARTESIAN_POINT('Ctrl Pts',(1.92583176936386,4.84463516096244,50.014227224265));
#62022=CARTESIAN_POINT('Ctrl Pts',(3.17954335484605,3.79395606061911,49.961306970183));
#62023=CARTESIAN_POINT('Ctrl Pts',(4.43325494032821,2.74327696027582,49.9083867161011));
#62024=CARTESIAN_POINT('Ctrl Pts',(5.11466620329769,1.00970662846638,49.8554664620191));
#62025=CARTESIAN_POINT('Ctrl Pts',(4.91195294283073,-0.613446674675755,
49.8025462079371));
#62026=CARTESIAN_POINT('Ctrl Pts',(4.70923968236377,-2.23659997781789,49.7496259538552));
#62027=CARTESIAN_POINT('Ctrl Pts',(3.62240189846027,-3.74933625229266,49.6967056997732));
#62028=CARTESIAN_POINT('Ctrl Pts',(2.14879315998069,-4.45940427533482,49.6437854456913));
#62029=CARTESIAN_POINT('Ctrl Pts',(0.675184421501018,-5.16947229837701,
49.5908651916093));
#62030=CARTESIAN_POINT('Ctrl Pts',(-1.18519527155483,-5.0768720699865,49.5379449375273));
#62031=CARTESIAN_POINT('Ctrl Pts',(-2.58100775862557,-4.22397886893019,
49.4850246834454));
#62032=CARTESIAN_POINT('Ctrl Pts',(-3.97682024569624,-3.37108566787394,
49.4321044293634));
#62033=CARTESIAN_POINT('Ctrl Pts',(-4.9080655267819,-1.75789949415196,49.3791841752814));
#62034=CARTESIAN_POINT('Ctrl Pts',(-4.94859153862899,-0.12263897856609,
49.3262639211994));
#62035=CARTESIAN_POINT('Ctrl Pts',(-4.94959816627151,-0.0820206605359307,
49.3249494323519));
#62036=CARTESIAN_POINT('Ctrl Pts',(-4.9500552393514,-0.0413887231133244,
49.3236349435044));
#62037=CARTESIAN_POINT('Ctrl Pts',(-4.94996872029631,-0.000754789231165454,
49.3223204546569));
#62038=CARTESIAN_POINT('Ctrl Pts',(-4.95009281286112,-0.000267728824007536,
49.1776795453432));
#62039=CARTESIAN_POINT('Ctrl Pts',(-4.95010408721063,-0.0146074376385199,
49.1781434595288));
#62040=CARTESIAN_POINT('Ctrl Pts',(-4.95004716359657,-0.02894705437045,
49.1786073737143));
#62041=CARTESIAN_POINT('Ctrl Pts',(-4.94992177176232,-0.0432860723615371,
49.1790712878999));
#62042=CARTESIAN_POINT('Ctrl Pts',(-4.93561790278161,-1.6789861630675,49.2319915419818));
#62043=CARTESIAN_POINT('Ctrl Pts',(-4.03035532991194,-3.30689499873837,
49.2849117960638));
#62044=CARTESIAN_POINT('Ctrl Pts',(-2.6483960323012,-4.18205663360964,49.3378320501458));
#62045=CARTESIAN_POINT('Ctrl Pts',(-1.26643673469055,-5.05721826848085,
49.3907523042277));
#62046=CARTESIAN_POINT('Ctrl Pts',(0.592219287661027,-5.17963270255261,
49.4436725583097));
#62047=CARTESIAN_POINT('Ctrl Pts',(2.07702265223193,-4.49328122119488,49.4965928123917));
#62048=CARTESIAN_POINT('Ctrl Pts',(3.56182601680279,-3.80692973983718,49.5495130664736));
#62049=CARTESIAN_POINT('Ctrl Pts',(4.67277672359291,-2.31181234304998,49.6024333205556));
#62050=CARTESIAN_POINT('Ctrl Pts',(4.90148676195955,-0.692117586080884,
49.6553535746375));
#62051=CARTESIAN_POINT('Ctrl Pts',(5.13019680032621,0.927577170888348,49.7082738287195));
#62052=CARTESIAN_POINT('Ctrl Pts',(4.47666617026921,2.67184928803957,49.7611940828015));
#62053=CARTESIAN_POINT('Ctrl Pts',(3.23996046927922,3.7424932048215,49.8141143368834));
#62054=CARTESIAN_POINT('Ctrl Pts',(2.00325476828929,4.81313712160337,49.8670345909654));
#62055=CARTESIAN_POINT('Ctrl Pts',(0.183373996366374,5.21015283801606,49.9199548450474));
#62056=CARTESIAN_POINT('Ctrl Pts',(-1.38687661076657,4.75185989872763,49.9728750991293));
#62057=CARTESIAN_POINT('Ctrl Pts',(-2.95712721789961,4.29356695943917,50.0257953532113));
#62058=CARTESIAN_POINT('Ctrl Pts',(-4.27774766024261,2.97996536444961,50.0787156072932));
#62059=CARTESIAN_POINT('Ctrl Pts',(-4.74440185394119,1.41217926586765,50.1316358613752));
#62060=CARTESIAN_POINT('Ctrl Pts',(-4.87974057311241,0.957491050521679,
50.1469837560312));
#62061=CARTESIAN_POINT('Ctrl Pts',(-4.94325117479429,0.481423074070403,
50.1623316506872));
#62062=CARTESIAN_POINT('Ctrl Pts',(-4.93925722597112,0.00431400617654748,
50.1776795453432));
#62063=CARTESIAN_POINT('Origin',(0.,0.,16.));
#62064=CARTESIAN_POINT('',(-4.9346053643787,-0.00190906406864477,51.3223204546569));
#62065=CARTESIAN_POINT('',(-4.93494424898874,-0.00229539766483815,51.1776795453432));
#62066=CARTESIAN_POINT('',(-4.942,-6.05220448138622E-16,16.));
#62067=CARTESIAN_POINT('Ctrl Pts',(-4.9346053643787,-0.00190906406864477,
51.3223204546569));
#62068=CARTESIAN_POINT('Ctrl Pts',(-4.93132359046474,0.942525285964724,
51.2920113258213));
#62069=CARTESIAN_POINT('Ctrl Pts',(-4.67058264693544,1.88863740917005,51.2617021969857));
#62070=CARTESIAN_POINT('Ctrl Pts',(-4.16399066183724,2.67671072463696,51.2313930681501));
#62071=CARTESIAN_POINT('Ctrl Pts',(-3.27947244580022,4.05270012756452,51.1784728140682));
#62072=CARTESIAN_POINT('Ctrl Pts',(-1.64545880455478,4.94689631680689,51.1255525599862));
#62073=CARTESIAN_POINT('Ctrl Pts',(-0.00969933613304136,4.95010145937766,
51.0726323059043));
#62074=CARTESIAN_POINT('Ctrl Pts',(1.62606013228874,4.95330660194842,51.0197120518223));
#62075=CARTESIAN_POINT('Ctrl Pts',(3.26356542788682,4.06552069784751,50.9667917977403));
#62076=CARTESIAN_POINT('Ctrl Pts',(4.15346911827026,2.69300813567829,50.9138715436584));
#62077=CARTESIAN_POINT('Ctrl Pts',(5.04337280865373,1.32049557350902,50.8609512895764));
#62078=CARTESIAN_POINT('Ctrl Pts',(5.18567489382252,-0.536743646728604,
50.8080310354945));
#62079=CARTESIAN_POINT('Ctrl Pts',(4.5152557662665,-2.0288084927985,50.7551107814125));
#62080=CARTESIAN_POINT('Ctrl Pts',(3.8448366387105,-3.52087333886836,50.7021905273305));
#62081=CARTESIAN_POINT('Ctrl Pts',(2.36169629842972,-4.64776381077051,50.6492702732485));
#62082=CARTESIAN_POINT('Ctrl Pts',(0.74454241669244,-4.89379761790371,50.5963500191666));
#62083=CARTESIAN_POINT('Ctrl Pts',(-0.872611465044887,-5.13983142503691,
50.5434297650846));
#62084=CARTESIAN_POINT('Ctrl Pts',(-2.62377888823873,-4.50500856740112,
50.4905095110027));
#62085=CARTESIAN_POINT('Ctrl Pts',(-3.70759889498285,-3.27983368010881,
50.4375892569207));
#62086=CARTESIAN_POINT('Ctrl Pts',(-4.49451017129344,-2.39029120233235,
50.3991663228328));
#62087=CARTESIAN_POINT('Ctrl Pts',(-4.92962682740573,-1.18954250282331,
50.3607433887448));
#62088=CARTESIAN_POINT('Ctrl Pts',(-4.94000433004934,0.00442567287284368,
50.3223204546569));
#62089=CARTESIAN_POINT('Ctrl Pts',(-4.93925722597112,0.00431400617654748,
50.1776795453432));
#62090=CARTESIAN_POINT('Ctrl Pts',(-4.92947985362941,-1.16367116612706,
50.2152519047692));
#62091=CARTESIAN_POINT('Ctrl Pts',(-4.51515233090316,-2.33789552818176,
50.2528242641951));
#62092=CARTESIAN_POINT('Ctrl Pts',(-3.75970560074729,-3.21997096669155,
50.2903966236211));
#62093=CARTESIAN_POINT('Ctrl Pts',(-2.69566720880064,-4.46236449849485,
50.3433168777031));
#62094=CARTESIAN_POINT('Ctrl Pts',(-0.95490247985317,-5.12518095992721,
50.396237131785));
#62095=CARTESIAN_POINT('Ctrl Pts',(0.665988059953313,-4.90510541524102,
50.449157385867));
#62096=CARTESIAN_POINT('Ctrl Pts',(2.28687859975984,-4.68502987055481,50.5020776399489));
#62097=CARTESIAN_POINT('Ctrl Pts',(3.78789495042532,-3.58206231974999,50.5549978940309));
#62098=CARTESIAN_POINT('Ctrl Pts',(4.48214910531455,-2.10093755936608,50.6079181481129));
#62099=CARTESIAN_POINT('Ctrl Pts',(5.17640326020376,-0.619812798982218,
50.6608384021949));
#62100=CARTESIAN_POINT('Ctrl Pts',(5.06389521931669,1.2394691709808,50.7137586562768));
#62101=CARTESIAN_POINT('Ctrl Pts',(4.19611038046471,2.62607252481409,50.7666789103588));
#62102=CARTESIAN_POINT('Ctrl Pts',(3.32832554161272,4.01267587864738,50.8195991644407));
#62103=CARTESIAN_POINT('Ctrl Pts',(1.70526390479588,4.92660061635104,50.8725194185227));
#62104=CARTESIAN_POINT('Ctrl Pts',(0.0696632635531223,4.94962081985461,
50.9254396726047));
#62105=CARTESIAN_POINT('Ctrl Pts',(-1.56593737768968,4.97264102335818,50.9783599266866));
#62106=CARTESIAN_POINT('Ctrl Pts',(-3.21407702335836,4.1047566926616,51.0312801807686));
#62107=CARTESIAN_POINT('Ctrl Pts',(-4.12054180005445,2.74312495242765,51.0842004348505));
#62108=CARTESIAN_POINT('Ctrl Pts',(-4.65427267801061,1.94138954819395,51.1153601383481));
#62109=CARTESIAN_POINT('Ctrl Pts',(-4.93087142137606,0.968476272531438,
51.1465198418457));
#62110=CARTESIAN_POINT('Ctrl Pts',(-4.93494424898874,-0.00229539766483815,
51.1776795453432));
#62111=CARTESIAN_POINT('Origin',(0.,0.,16.));
#62112=CARTESIAN_POINT('',(-4.94698954266231,-0.00340802453188072,52.3223204546568));
#62113=CARTESIAN_POINT('',(-4.94764183754834,-0.00307943510729547,52.1776795453432));
#62114=CARTESIAN_POINT('',(-4.942,-6.05220448138622E-16,16.));
#62115=CARTESIAN_POINT('Ctrl Pts',(-4.94698954266231,-0.00340802453188072,
52.3223204546568));
#62116=CARTESIAN_POINT('Ctrl Pts',(-4.93574079437759,1.42456851634609,52.2761995169797));
#62117=CARTESIAN_POINT('Ctrl Pts',(-4.28342182577614,2.86150661417242,52.2300785793026));
#62118=CARTESIAN_POINT('Ctrl Pts',(-3.19438680274345,3.78146684366169,52.1839576416255));
#62119=CARTESIAN_POINT('Ctrl Pts',(-1.94480227507184,4.83705095668842,52.1310373875436));
#62120=CARTESIAN_POINT('Ctrl Pts',(-0.120245685876333,5.21199182863453,
52.0781171334615));
#62121=CARTESIAN_POINT('Ctrl Pts',(1.44433800372382,4.73471079013843,52.0251968793796));
#62122=CARTESIAN_POINT('Ctrl Pts',(3.00892169332389,4.25742975164236,51.9722766252976));
#62123=CARTESIAN_POINT('Ctrl Pts',(4.31353248332859,2.92792680270421,51.9193563712157));
#62124=CARTESIAN_POINT('Ctrl Pts',(4.7611605513041,1.3546027978562,51.8664361171337));
#62125=CARTESIAN_POINT('Ctrl Pts',(5.20878861927959,-0.218721206991761,
51.8135158630518));
#62126=CARTESIAN_POINT('Ctrl Pts',(4.79943396522586,-2.03586626774964,51.7605956089698));
#62127=CARTESIAN_POINT('Ctrl Pts',(3.72042353078829,-3.26527905190521,51.7076753548878));
#62128=CARTESIAN_POINT('Ctrl Pts',(2.64141309635066,-4.49469183606084,51.6547551008059));
#62129=CARTESIAN_POINT('Ctrl Pts',(0.892746881529132,-5.1363723436142,51.6018348467239));
#62130=CARTESIAN_POINT('Ctrl Pts',(-0.725358746921474,-4.8966777741157,
51.5489145926419));
#62131=CARTESIAN_POINT('Ctrl Pts',(-2.34346437537199,-4.65698320461722,
51.49599433856));
#62132=CARTESIAN_POINT('Ctrl Pts',(-3.83100941745154,-3.535913558067,51.443074084478));
#62133=CARTESIAN_POINT('Ctrl Pts',(-4.50727054307715,-2.04648742648548,
51.3901538303961));
#62134=CARTESIAN_POINT('Ctrl Pts',(-4.79621520662888,-1.41010346743882,
51.3675427051497));
#62135=CARTESIAN_POINT('Ctrl Pts',(-4.93705362349566,-0.70647314083382,
51.3449315799033));
#62136=CARTESIAN_POINT('Ctrl Pts',(-4.9346053643787,-0.00190906406864477,
51.3223204546569));
#62137=CARTESIAN_POINT('Ctrl Pts',(-4.93494424898874,-0.00229539766483815,
51.1776795453432));
#62138=CARTESIAN_POINT('Ctrl Pts',(-4.9377885305877,-0.680239141156077,
51.1994400959276));
#62139=CARTESIAN_POINT('Ctrl Pts',(-4.80772180958983,-1.35713842276963,
51.221200646512));
#62140=CARTESIAN_POINT('Ctrl Pts',(-4.53950114466406,-1.9739626613036,51.2429611970964));
#62141=CARTESIAN_POINT('Ctrl Pts',(-3.88720580485411,-3.47403938502989,
51.2958814511784));
#62142=CARTESIAN_POINT('Ctrl Pts',(-2.41782521751062,-4.61881368271118,
51.3488017052603));
#62143=CARTESIAN_POINT('Ctrl Pts',(-0.803770380809228,-4.88441935193539,
51.4017219593423));
#62144=CARTESIAN_POINT('Ctrl Pts',(0.810284455892164,-5.1500250211596,51.4546422134243));
#62145=CARTESIAN_POINT('Ctrl Pts',(2.56901354195146,-4.53646206192671,51.5075624675063));
#62146=CARTESIAN_POINT('Ctrl Pts',(3.6675955870482,-3.32450625514402,51.5604827215882));
#62147=CARTESIAN_POINT('Ctrl Pts',(4.7661776321449,-2.11255044836137,51.6134029756702));
#62148=CARTESIAN_POINT('Ctrl Pts',(5.20461263627908,-0.302201794028944,
51.6663232297521));
#62149=CARTESIAN_POINT('Ctrl Pts',(4.78226604547315,1.27809651472091,51.7192434838341));
#62150=CARTESIAN_POINT('Ctrl Pts',(4.3599194546672,2.85839482347081,51.7721637379161));
#62151=CARTESIAN_POINT('Ctrl Pts',(3.07679126892111,4.20864278663813,51.825083991998));
#62152=CARTESIAN_POINT('Ctrl Pts',(1.52006054286266,4.71094631434696,51.87800424608));
#62153=CARTESIAN_POINT('Ctrl Pts',(-0.0366701831957017,5.21324984205576,
51.930924500162));
#62154=CARTESIAN_POINT('Ctrl Pts',(-1.86700344956638,4.86760893430616,51.9838447542439));
#62155=CARTESIAN_POINT('Ctrl Pts',(-3.13335079942941,3.83219414935389,52.0367650083259));
#62156=CARTESIAN_POINT('Ctrl Pts',(-4.25734861844162,2.9131698704424,52.083736520665));
#62157=CARTESIAN_POINT('Ctrl Pts',(-4.93702884968978,1.45073013335928,52.1307080330041));
#62158=CARTESIAN_POINT('Ctrl Pts',(-4.94764183754834,-0.00307943510729547,
52.1776795453432));
#62159=CARTESIAN_POINT('Origin',(0.,0.,16.));
#62160=CARTESIAN_POINT('',(-4.94509673752737,0.0040742516207555,53.3223204546569));
#62161=CARTESIAN_POINT('',(-4.94431829400652,0.00425244366110885,53.1776795453432));
#62162=CARTESIAN_POINT('',(-4.942,-6.05220448138622E-16,16.));
#62163=CARTESIAN_POINT('Ctrl Pts',(-4.94509673752737,0.0040742516207555,
53.3223204546569));
#62164=CARTESIAN_POINT('Ctrl Pts',(-4.94757864022345,0.283393084706415,
53.3133079622201));
#62165=CARTESIAN_POINT('Ctrl Pts',(-4.92595073565188,0.562327591030859,
53.3042954697834));
#62166=CARTESIAN_POINT('Ctrl Pts',(-4.87885318126865,0.836893165749963,
53.2952829773467));
#62167=CARTESIAN_POINT('Ctrl Pts',(-4.60230209819144,2.44910866310731,53.2423627232647));
#62168=CARTESIAN_POINT('Ctrl Pts',(-3.44758426677398,3.91068799192893,53.1894424691828));
#62169=CARTESIAN_POINT('Ctrl Pts',(-1.94311620233063,4.55279012908506,53.1365222151008));
#62170=CARTESIAN_POINT('Ctrl Pts',(-0.438648137887247,5.19489226624121,
53.0836019610189));
#62171=CARTESIAN_POINT('Ctrl Pts',(1.4155701595821,5.01751721173186,53.0306817069369));
#62172=CARTESIAN_POINT('Ctrl Pts',(2.77102007823768,4.10183449949628,52.9777614528549));
#62173=CARTESIAN_POINT('Ctrl Pts',(4.12646999689325,3.1861517872607,52.924841198773));
#62174=CARTESIAN_POINT('Ctrl Pts',(4.98315153673507,1.53216141729899,52.871920944691));
#62175=CARTESIAN_POINT('Ctrl Pts',(4.9490341412924,-0.10324535619766,52.8190006906091));
#62176=CARTESIAN_POINT('Ctrl Pts',(4.91491674584974,-1.73865212969422,52.7660804365271));
#62177=CARTESIAN_POINT('Ctrl Pts',(3.99000041512261,-3.35547530672568,52.7131601824451));
#62178=CARTESIAN_POINT('Ctrl Pts',(2.59754098802034,-4.21383190822896,52.6602399283632));
#62179=CARTESIAN_POINT('Ctrl Pts',(1.205081560918,-5.07218850973229,52.6073196742812));
#62180=CARTESIAN_POINT('Ctrl Pts',(-0.654920962559591,-5.17207853570735,
52.5543994201993));
#62181=CARTESIAN_POINT('Ctrl Pts',(-2.13130102041059,-4.4677907846777,52.5014791661173));
#62182=CARTESIAN_POINT('Ctrl Pts',(-3.6076810782616,-3.76350303364805,52.4485589120353));
#62183=CARTESIAN_POINT('Ctrl Pts',(-4.70043867048604,-2.25503750561363,
52.3956386579533));
#62184=CARTESIAN_POINT('Ctrl Pts',(-4.90951123352436,-0.632691064542821,
52.3427184038713));
#62185=CARTESIAN_POINT('Ctrl Pts',(-4.93637335904372,-0.424248248792036,
52.3359190874665));
#62186=CARTESIAN_POINT('Ctrl Pts',(-4.94864787405361,-0.213925520686765,
52.3291197710617));
#62187=CARTESIAN_POINT('Ctrl Pts',(-4.94698954266231,-0.00340802453188072,
52.3223204546568));
#62188=CARTESIAN_POINT('Ctrl Pts',(-4.94764183754834,-0.00307943510729547,
52.1776795453432));
#62189=CARTESIAN_POINT('Ctrl Pts',(-4.94898592720496,-0.187198217650565,
52.1836282870861));
#62190=CARTESIAN_POINT('Ctrl Pts',(-4.93959875206843,-0.371178579690442,
52.1895770288289));
#62191=CARTESIAN_POINT('Ctrl Pts',(-4.91902378063747,-0.553899157022463,
52.1955257705718));
#62192=CARTESIAN_POINT('Ctrl Pts',(-4.73598797862701,-2.17938901629118,
52.2484460246538));
#62193=CARTESIAN_POINT('Ctrl Pts',(-3.66755494125079,-3.70518007267354,
52.3013662787357));
#62194=CARTESIAN_POINT('Ctrl Pts',(-2.2026559442682,-4.43304703582165,52.3542865328177));
#62195=CARTESIAN_POINT('Ctrl Pts',(-0.737756947285612,-5.16091399896976,
52.4072067868996));
#62196=CARTESIAN_POINT('Ctrl Pts',(1.12360800930335,-5.09085686888362,52.4601270409816));
#62197=CARTESIAN_POINT('Ctrl Pts',(2.52964989329714,-4.2549348582521,52.5130472950635));
#62198=CARTESIAN_POINT('Ctrl Pts',(3.93569177729098,-3.41901284762056,52.5659675491455));
#62199=CARTESIAN_POINT('Ctrl Pts',(4.88641058868961,-1.81722595644361,52.6188878032275));
#62200=CARTESIAN_POINT('Ctrl Pts',(4.94674287935491,-0.182576329732651,
52.6718080573094));
#62201=CARTESIAN_POINT('Ctrl Pts',(5.0070751700202,1.45207329697826,52.7247283113914));
#62202=CARTESIAN_POINT('Ctrl Pts',(4.17702093995222,3.11958565922317,52.7776485654734));
#62203=CARTESIAN_POINT('Ctrl Pts',(2.83642568199835,4.05688163262466,52.8305688195553));
#62204=CARTESIAN_POINT('Ctrl Pts',(1.49583042404448,4.99417760602615,52.8834890736373));
#62205=CARTESIAN_POINT('Ctrl Pts',(-0.355305861795278,5.20125719058422,
52.9364093277193));
#62206=CARTESIAN_POINT('Ctrl Pts',(-1.86987493927361,4.58335760574097,52.9893295818012));
#62207=CARTESIAN_POINT('Ctrl Pts',(-3.384444016752,3.9654580208977,53.0422498358832));
#62208=CARTESIAN_POINT('Ctrl Pts',(-4.56244588586893,2.52257926665306,53.0951700899651));
#62209=CARTESIAN_POINT('Ctrl Pts',(-4.86480890004871,0.915004697602124,
53.1480903440471));
#62210=CARTESIAN_POINT('Ctrl Pts',(-4.92116211960056,0.615391324314909,
53.1579534111458));
#62211=CARTESIAN_POINT('Ctrl Pts',(-4.94709912492537,0.310057072885753,
53.1678164782445));
#62212=CARTESIAN_POINT('Ctrl Pts',(-4.94431829400652,0.00425244366110885,
53.1776795453432));
#62213=CARTESIAN_POINT('Origin',(0.,0.,16.));
#62214=CARTESIAN_POINT('',(-4.93403082595878,0.000832190755156725,54.3223204546569));
#62215=CARTESIAN_POINT('',(-4.93393232083006,0.000401187422265207,54.1776795453432));
#62216=CARTESIAN_POINT('',(-4.942,-6.05220448138622E-16,16.));
#62217=CARTESIAN_POINT('Ctrl Pts',(-4.93403082595878,0.000832190755156725,
54.3223204546569));
#62218=CARTESIAN_POINT('Ctrl Pts',(-4.93519480376781,0.77458390453562,54.2974961533786));
#62219=CARTESIAN_POINT('Ctrl Pts',(-4.76408859627892,1.54784860488958,54.2726718521003));
#62220=CARTESIAN_POINT('Ctrl Pts',(-4.41799967623941,2.23268389970517,54.2478475508221));
#62221=CARTESIAN_POINT('Ctrl Pts',(-3.6802099846732,3.69261050145239,54.1949272967401));
#62222=CARTESIAN_POINT('Ctrl Pts',(-2.14720464186602,4.75066627671043,54.1420070426582));
#62223=CARTESIAN_POINT('Ctrl Pts',(-0.52051030581542,4.92266874335397,54.0890867885762));
#62224=CARTESIAN_POINT('Ctrl Pts',(1.10618403023518,5.0946712099975,54.0361665344942));
#62225=CARTESIAN_POINT('Ctrl Pts',(2.82656735952921,4.38062036802653,53.9832462804122));
#62226=CARTESIAN_POINT('Ctrl Pts',(3.85336599568517,3.10727678821045,53.9303260263302));
#62227=CARTESIAN_POINT('Ctrl Pts',(4.8801646318411,1.83393320839441,53.8774057722483));
#62228=CARTESIAN_POINT('Ctrl Pts',(5.21337857485901,0.00129689073330608,
53.8244855181664));
#62229=CARTESIAN_POINT('Ctrl Pts',(4.70052403533771,-1.55198979650856,53.7715652640844));
#62230=CARTESIAN_POINT('Ctrl Pts',(4.18766949581641,-3.10527648375042,53.7186450100024));
#62231=CARTESIAN_POINT('Ctrl Pts',(2.82874647375599,-4.37921354057296,53.6657247559204));
#62232=CARTESIAN_POINT('Ctrl Pts',(1.24561889847324,-4.79082791331733,53.6128045018385));
#62233=CARTESIAN_POINT('Ctrl Pts',(-0.337508676809509,-5.2024422860617,
53.5598842477565));
#62234=CARTESIAN_POINT('Ctrl Pts',(-2.14484080531469,-4.75173397472772,
53.5069639936746));
#62235=CARTESIAN_POINT('Ctrl Pts',(-3.34931470219873,-3.64495398611418,
53.4540437395926));
#62236=CARTESIAN_POINT('Ctrl Pts',(-4.34866275314335,-2.72666225118592,
53.4101359779474));
#62237=CARTESIAN_POINT('Ctrl Pts',(-4.93300521093011,-1.35673296483636,
53.3662282163021));
#62238=CARTESIAN_POINT('Ctrl Pts',(-4.94509673752737,0.0040742516207555,
53.3223204546569));
#62239=CARTESIAN_POINT('Ctrl Pts',(-4.94431829400652,0.00425244366110885,
53.1776795453432));
#62240=CARTESIAN_POINT('Ctrl Pts',(-4.93217858577541,-1.33073665953657,
53.2207367323265));
#62241=CARTESIAN_POINT('Ctrl Pts',(-4.37274694612505,-2.67469001651735,
53.2637939193098));
#62242=CARTESIAN_POINT('Ctrl Pts',(-3.4073211579765,-3.59078845896452,53.306851106293));
#62243=CARTESIAN_POINT('Ctrl Pts',(-2.22074624248181,-4.71673666262315,
53.359771360375));
#62244=CARTESIAN_POINT('Ctrl Pts',(-0.42087225224974,-5.19636268608309,
53.4126916144569));
#62245=CARTESIAN_POINT('Ctrl Pts',(1.16865098585596,-4.81018233582522,53.4656118685389));
#62246=CARTESIAN_POINT('Ctrl Pts',(2.75817422396157,-4.42400198556738,53.5185321226208));
#62247=CARTESIAN_POINT('Ctrl Pts',(4.13734670994089,-3.17201526159183,53.5714523767028));
#62248=CARTESIAN_POINT('Ctrl Pts',(4.6750380505237,-1.62715041000601,53.6243726307848));
#62249=CARTESIAN_POINT('Ctrl Pts',(5.2127293911065,-0.0822855584201898,
53.6772928848668));
#62250=CARTESIAN_POINT('Ctrl Pts',(4.90893958629287,1.75545742077581,53.7302131389487));
#62251=CARTESIAN_POINT('Ctrl Pts',(3.9026874904557,3.045099273007,53.7831333930307));
#62252=CARTESIAN_POINT('Ctrl Pts',(2.89643539461849,4.33474112523822,53.8360536471126));
#62253=CARTESIAN_POINT('Ctrl Pts',(1.18772100775765,5.0762818505045,53.8889739011946));
#62254=CARTESIAN_POINT('Ctrl Pts',(-0.441521870018959,4.93038108759577,
53.9418941552766));
#62255=CARTESIAN_POINT('Ctrl Pts',(-2.07076474779552,4.78448032468705,53.9948144093585));
#62256=CARTESIAN_POINT('Ctrl Pts',(-3.62053611648792,3.75113807360336,54.0477346634405));
#62257=CARTESIAN_POINT('Ctrl Pts',(-4.38163692859106,2.30322753036564,54.1006549175225));
#62258=CARTESIAN_POINT('Ctrl Pts',(-4.75089382782116,1.60075691273335,54.1263297934627));
#62259=CARTESIAN_POINT('Ctrl Pts',(-4.9345120375631,0.800704467282281,54.152004669403));
#62260=CARTESIAN_POINT('Ctrl Pts',(-4.93393232083006,0.000401187422265207,
54.1776795453432));
#62261=CARTESIAN_POINT('Origin',(0.,0.,16.));
#62262=CARTESIAN_POINT('',(-4.94204396072975,-0.00451108372972908,55.3223204546568));
#62263=CARTESIAN_POINT('',(-4.94284599866247,-0.00446247280752122,55.1776795453432));
#62264=CARTESIAN_POINT('',(-4.942,-6.05220448138622E-16,16.));
#62265=CARTESIAN_POINT('Ctrl Pts',(-4.94204396072975,-0.00451108372972908,
55.3223204546568));
#62266=CARTESIAN_POINT('Ctrl Pts',(-4.93045565886636,1.25690241555476,55.281684344537));
#62267=CARTESIAN_POINT('Ctrl Pts',(-4.43833582829864,2.52635331123123,55.2410482344173));
#62268=CARTESIAN_POINT('Ctrl Pts',(-3.56758671933519,3.43160655309978,55.2004121242975));
#62269=CARTESIAN_POINT('Ctrl Pts',(-2.43361341450575,4.61051446104039,55.1474918702155));
#62270=CARTESIAN_POINT('Ctrl Pts',(-0.65749411504605,5.17175205664432,55.0945716161334));
#62271=CARTESIAN_POINT('Ctrl Pts',(0.947991861475882,4.85848844455039,55.0416513620514));
#62272=CARTESIAN_POINT('Ctrl Pts',(2.55347783799768,4.54522483245649,54.9887311079695));
#62273=CARTESIAN_POINT('Ctrl Pts',(3.98833049158174,3.35746001266491,54.9358108538876));
#62274=CARTESIAN_POINT('Ctrl Pts',(4.59593933387555,1.83873330708663,54.8828905998056));
#62275=CARTESIAN_POINT('Ctrl Pts',(5.2035481761694,0.320006601508274,54.8299703457237));
#62276=CARTESIAN_POINT('Ctrl Pts',(4.98391320717291,-1.52968198985681,54.7770500916417));
#62277=CARTESIAN_POINT('Ctrl Pts',(4.0375427431176,-2.86388671786309,54.7241298375597));
#62278=CARTESIAN_POINT('Ctrl Pts',(3.09117227906232,-4.19809144586933,54.6712095834777));
#62279=CARTESIAN_POINT('Ctrl Pts',(1.41806631994828,-5.0168123105168,54.6182893293958));
#62280=CARTESIAN_POINT('Ctrl Pts',(-0.216136294490469,-4.94539014006561,
54.5653690753138));
#62281=CARTESIAN_POINT('Ctrl Pts',(-1.85033890892918,-4.87396796961441,
54.5124488212319));
#62282=CARTESIAN_POINT('Ctrl Pts',(-3.4456381786926,-3.91240276406461,54.4595285671499));
#62283=CARTESIAN_POINT('Ctrl Pts',(-4.27200079341172,-2.50072144717157,
54.4066083130679));
#62284=CARTESIAN_POINT('Ctrl Pts',(-4.7107259171786,-1.75124409976784,54.3785123602642));
#62285=CARTESIAN_POINT('Ctrl Pts',(-4.93271344484821,-0.874894033659396,
54.3504164074605));
#62286=CARTESIAN_POINT('Ctrl Pts',(-4.93403082595878,0.000832190755156725,
54.3223204546569));
#62287=CARTESIAN_POINT('Ctrl Pts',(-4.93393232083006,0.000401187422265207,
54.1776795453432));
#62288=CARTESIAN_POINT('Ctrl Pts',(-4.93331714350093,-0.848855710199169,
54.2049249234849));
#62289=CARTESIAN_POINT('Ctrl Pts',(-4.72528049547278,-1.69839506725433,
54.2321703016266));
#62290=CARTESIAN_POINT('Ctrl Pts',(-4.31154403127411,-2.43191021565593,
54.2594156797684));
#62291=CARTESIAN_POINT('Ctrl Pts',(-3.50792006634005,-3.85665858304818,
54.3123359338503));
#62292=CARTESIAN_POINT('Ctrl Pts',(-1.92824188095795,-4.8436764824408,54.3652561879323));
#62293=CARTESIAN_POINT('Ctrl Pts',(-0.295394338707872,-4.9412894486446,
54.4181764420142));
#62294=CARTESIAN_POINT('Ctrl Pts',(1.33745320354216,-5.0389024148484,54.4710966960962));
#62295=CARTESIAN_POINT('Ctrl Pts',(3.02347010266025,-4.24711044786332,54.5240169501782));
#62296=CARTESIAN_POINT('Ctrl Pts',(3.99110927558139,-2.92824964458212,54.5769372042601));
#62297=CARTESIAN_POINT('Ctrl Pts',(4.95874844850256,-1.60938884130088,54.6298574583421));
#62298=CARTESIAN_POINT('Ctrl Pts',(5.20800989522687,0.236540798276539,54.6827777124241));
#62299=CARTESIAN_POINT('Ctrl Pts',(4.62482777083827,1.76481367875202,54.735697966506));
#62300=CARTESIAN_POINT('Ctrl Pts',(4.04164564644968,3.29308655922746,54.788618220588));
#62301=CARTESIAN_POINT('Ctrl Pts',(2.62601995094824,4.50370268060093,54.8415384746699));
#62302=CARTESIAN_POINT('Ctrl Pts',(1.02576262302031,4.84266561635652,54.8944587287519));
#62303=CARTESIAN_POINT('Ctrl Pts',(-0.574494704907621,5.1816285521121,54.9473789828339));
#62304=CARTESIAN_POINT('Ctrl Pts',(-2.35938366526199,4.64893830224978,55.0002992369159));
#62305=CARTESIAN_POINT('Ctrl Pts',(-3.51211180971311,3.48836206072432,55.0532194909978));
#62306=CARTESIAN_POINT('Ctrl Pts',(-4.4157898059278,2.57853157081683,55.0947061757796));
#62307=CARTESIAN_POINT('Ctrl Pts',(-4.93095870305679,1.2828191742603,55.1361928605614));
#62308=CARTESIAN_POINT('Ctrl Pts',(-4.94284599866247,-0.00446247280752122,
55.1776795453432));
#62309=CARTESIAN_POINT('Origin',(0.,0.,16.));
#62310=CARTESIAN_POINT('',(-4.94916162572937,0.00195780085970945,56.3223204546569));
#62311=CARTESIAN_POINT('',(-4.9486927940556,0.00238008058365034,56.1776795453432));
#62312=CARTESIAN_POINT('',(-4.942,-6.05220448138622E-16,16.));
#62313=CARTESIAN_POINT('Ctrl Pts',(-4.94916162572937,0.00195780085970945,
56.3223204546569));
#62314=CARTESIAN_POINT('Ctrl Pts',(-4.94971144692239,0.111053665337975,
56.3187927897774));
#62315=CARTESIAN_POINT('Ctrl Pts',(-4.94641661384693,0.220115719674017,
56.315265124898));
#62316=CARTESIAN_POINT('Ctrl Pts',(-4.93917135292333,0.328914702796541,
56.3117374600186));
#62317=CARTESIAN_POINT('Ctrl Pts',(-4.83048159296228,1.96106232098248,56.2588172059367));
#62318=CARTESIAN_POINT('Ctrl Pts',(-3.83276814539685,3.53400710106189,56.2058969518547));
#62319=CARTESIAN_POINT('Ctrl Pts',(-2.40259992160997,4.32794548855851,56.1529766977728));
#62320=CARTESIAN_POINT('Ctrl Pts',(-0.972431697823093,5.12188387605513,
56.1000564436908));
#62321=CARTESIAN_POINT('Ctrl Pts',(0.890191302185183,5.13681587096895,56.0471361896088));
#62322=CARTESIAN_POINT('Ctrl Pts',(2.33290434633096,4.36590836437554,55.9942159355269));
#62323=CARTESIAN_POINT('Ctrl Pts',(3.77561739047674,3.59500085778213,55.9412956814449));
#62324=CARTESIAN_POINT('Ctrl Pts',(4.79842047875997,2.03825384968152,55.8883754273629));
#62325=CARTESIAN_POINT('Ctrl Pts',(4.93326329701873,0.408058546708748,55.8354551732809));
#62326=CARTESIAN_POINT('Ctrl Pts',(5.0681061152775,-1.22213675626403,55.782534919199));
#62327=CARTESIAN_POINT('Ctrl Pts',(4.31498866351168,-2.92578035410902,55.729614665117));
#62328=CARTESIAN_POINT('Ctrl Pts',(3.01854898978546,-3.92325891721657,55.6766944110351));
#62329=CARTESIAN_POINT('Ctrl Pts',(1.72210931605921,-4.92073748032415,55.6237741569531));
#62330=CARTESIAN_POINT('Ctrl Pts',(-0.117652579627481,-5.21205100869435,
55.5708539028712));
#62331=CARTESIAN_POINT('Ctrl Pts',(-1.65883355567899,-4.66388998260118,
55.5179336487892));
#62332=CARTESIAN_POINT('Ctrl Pts',(-3.20001453173045,-4.11572895650802,
55.4650133947072));
#62333=CARTESIAN_POINT('Ctrl Pts',(-4.4426145881467,-2.72809337595155,55.4120931406252));
#62334=CARTESIAN_POINT('Ctrl Pts',(-4.81800096125524,-1.13598647553473,
55.3591728865432));
#62335=CARTESIAN_POINT('Ctrl Pts',(-4.90513773579808,-0.766417759225417,
55.3468887425811));
#62336=CARTESIAN_POINT('Ctrl Pts',(-4.94554706100059,-0.385831662281748,
55.334604598619));
#62337=CARTESIAN_POINT('Ctrl Pts',(-4.94204396072975,-0.00451108372972908,
55.3223204546568));
#62338=CARTESIAN_POINT('Ctrl Pts',(-4.94284599866247,-0.00446247280752122,
55.1776795453432));
#62339=CARTESIAN_POINT('Ctrl Pts',(-4.94612209119225,-0.359232298306442,
55.1891131146434));
#62340=CARTESIAN_POINT('Ctrl Pts',(-4.91117232521921,-0.713361781229651,
55.2005466839435));
#62341=CARTESIAN_POINT('Ctrl Pts',(-4.83559423534505,-1.05859700628939,
55.2119802532437));
#62342=CARTESIAN_POINT('Ctrl Pts',(-4.48578118797803,-2.6565175985889,55.2649005073256));
#62343=CARTESIAN_POINT('Ctrl Pts',(-3.26558776469621,-4.06389654999934,
55.3178207614076));
#62344=CARTESIAN_POINT('Ctrl Pts',(-1.73339311164005,-4.63669575788038,
55.3707410154896));
#62345=CARTESIAN_POINT('Ctrl Pts',(-0.201198458583838,-5.20949496576144,
55.4236612695715));
#62346=CARTESIAN_POINT('Ctrl Pts',(1.64299742424673,-4.94771443011306,55.4765815236535));
#62347=CARTESIAN_POINT('Ctrl Pts',(2.95526233502001,-3.97114892214321,55.5295017777355));
#62348=CARTESIAN_POINT('Ctrl Pts',(4.26752724579325,-2.9945834141734,55.5824220318174));
#62349=CARTESIAN_POINT('Ctrl Pts',(5.04786118450924,-1.30323293388218,55.6353422858994));
#62350=CARTESIAN_POINT('Ctrl Pts',(4.93917142300628,0.328914707462642,55.6882625399813));
#62351=CARTESIAN_POINT('Ctrl Pts',(4.83048166150332,1.96106234880747,55.7411827940633));
#62352=CARTESIAN_POINT('Ctrl Pts',(3.83276819978142,3.5340071512059,55.7941030481453));
#62353=CARTESIAN_POINT('Ctrl Pts',(2.40259995570176,4.32794554996814,55.8470233022272));
#62354=CARTESIAN_POINT('Ctrl Pts',(0.972431711622098,5.12188394873038,55.8999435563092));
#62355=CARTESIAN_POINT('Ctrl Pts',(-0.890191314815322,5.13681594385641,
55.9528638103912));
#62356=CARTESIAN_POINT('Ctrl Pts',(-2.33290437943218,4.36590842632473,56.0057840644731));
#62357=CARTESIAN_POINT('Ctrl Pts',(-3.77561744404904,3.59500090879304,56.0587043185551));
#62358=CARTESIAN_POINT('Ctrl Pts',(-4.79842054684533,2.03825387860361,56.1116245726371));
#62359=CARTESIAN_POINT('Ctrl Pts',(-4.93326336701772,0.408058552499706,
56.164544826719));
#62360=CARTESIAN_POINT('Ctrl Pts',(-4.94441928789138,0.273187967299986,
56.1689230662604));
#62361=CARTESIAN_POINT('Ctrl Pts',(-4.94949737612309,0.137814649647994,
56.1733013058018));
#62362=CARTESIAN_POINT('Ctrl Pts',(-4.9486927940556,0.00238008058365034,
56.1776795453432));
#62363=CARTESIAN_POINT('Origin',(0.,0.,16.));
#62364=CARTESIAN_POINT('',(-4.93623902664834,0.00326946414225537,57.3223204546569));
#62365=CARTESIAN_POINT('',(-4.93573111423024,0.00295138605979709,57.1776795453432));
#62366=CARTESIAN_POINT('',(-4.942,-6.05220448138622E-16,16.));
#62367=CARTESIAN_POINT('Ctrl Pts',(-4.93623902664834,0.00326946414225537,
57.3223204546569));
#62368=CARTESIAN_POINT('Ctrl Pts',(-4.93989713650663,0.605389273547052,
57.3029809809359));
#62369=CARTESIAN_POINT('Ctrl Pts',(-4.83794904041642,1.20631307007342,57.2836415072149));
#62370=CARTESIAN_POINT('Ctrl Pts',(-4.62482770521538,1.76481365371148,57.2643020334939));
#62371=CARTESIAN_POINT('Ctrl Pts',(-4.04164558910142,3.29308651250188,57.211381779412));
#62372=CARTESIAN_POINT('Ctrl Pts',(-2.6260199136863,4.50370261669748,57.15846152533));
#62373=CARTESIAN_POINT('Ctrl Pts',(-1.02576260846464,4.84266554764316,57.1055412712481));
#62374=CARTESIAN_POINT('Ctrl Pts',(0.574494696756969,5.18162847858883,57.0526210171661));
#62375=CARTESIAN_POINT('Ctrl Pts',(2.35938363178511,4.64893823628462,56.9997007630841));
#62376=CARTESIAN_POINT('Ctrl Pts',(3.51211175987971,3.48836201122659,56.9467805090022));
#62377=CARTESIAN_POINT('Ctrl Pts',(4.66483988797431,2.32778578616857,56.8938602549202));
#62378=CARTESIAN_POINT('Ctrl Pts',(5.18540720913538,0.539323578356728,56.8409400008383));
#62379=CARTESIAN_POINT('Ctrl Pts',(4.83559416673167,-1.05859699126952,56.7880197467563));
#62380=CARTESIAN_POINT('Ctrl Pts',(4.48578112432795,-2.65651756089581,56.7350994926743));
#62381=CARTESIAN_POINT('Ctrl Pts',(3.26558771835941,-4.0638964923365,56.6821792385924));
#62382=CARTESIAN_POINT('Ctrl Pts',(1.73339308704371,-4.63669569208971,56.6292589845104));
#62383=CARTESIAN_POINT('Ctrl Pts',(0.201198455728012,-5.20949489184292,
56.5763387304284));
#62384=CARTESIAN_POINT('Ctrl Pts',(-1.64299740093485,-4.94771435990864,
56.5234184763465));
#62385=CARTESIAN_POINT('Ctrl Pts',(-2.95526229308795,-3.97114886579523,
56.4704982222645));
#62386=CARTESIAN_POINT('Ctrl Pts',(-4.18005158912286,-3.0596812412178,56.4211056330619));
#62387=CARTESIAN_POINT('Ctrl Pts',(-4.94146330594845,-1.52554761761349,
56.3717130438594));
#62388=CARTESIAN_POINT('Ctrl Pts',(-4.94916162572937,0.00195780085970945,
56.3223204546569));
#62389=CARTESIAN_POINT('Ctrl Pts',(-4.9486927940556,0.00238008058365034,
56.1776795453432));
#62390=CARTESIAN_POINT('Ctrl Pts',(-4.93977230579782,-1.49919761032442,
56.2262215598838));
#62391=CARTESIAN_POINT('Ctrl Pts',(-4.20773066973569,-3.00830456759471,
56.2747635744243));
#62392=CARTESIAN_POINT('Ctrl Pts',(-3.018549032617,-3.92325897288391,56.3233055889649));
#62393=CARTESIAN_POINT('Ctrl Pts',(-1.72210934049551,-4.92073755014514,
56.3762258430469));
#62394=CARTESIAN_POINT('Ctrl Pts',(0.117652581295909,-5.2120510826492,56.4291460971289));
#62395=CARTESIAN_POINT('Ctrl Pts',(1.65883357921563,-4.66389004877836,56.4820663512108));
#62396=CARTESIAN_POINT('Ctrl Pts',(3.2000145771353,-4.11572901490753,56.5349866052928));
#62397=CARTESIAN_POINT('Ctrl Pts',(4.44261465118334,-2.72809341466183,56.5879068593747));
#62398=CARTESIAN_POINT('Ctrl Pts',(4.8180010296186,-1.13598649165438,56.6408271134567));
#62399=CARTESIAN_POINT('Ctrl Pts',(5.19338740805387,0.456120431353115,56.6937473675386));
#62400=CARTESIAN_POINT('Ctrl Pts',(4.70156009087639,2.25269867712231,56.7466676216206));
#62401=CARTESIAN_POINT('Ctrl Pts',(3.56758676995704,3.43160660179086,56.7995878757026));
#62402=CARTESIAN_POINT('Ctrl Pts',(2.43361344903769,4.61051452645941,56.8525081297845));
#62403=CARTESIAN_POINT('Ctrl Pts',(0.65749412437644,5.17175213002719,56.9054283838665));
#62404=CARTESIAN_POINT('Ctrl Pts',(-0.94799187492607,4.85848851348866,56.9583486379485));
#62405=CARTESIAN_POINT('Ctrl Pts',(-2.55347787422853,4.54522489695015,57.0112688920304));
#62406=CARTESIAN_POINT('Ctrl Pts',(-3.98833054817231,3.35746006030537,57.0641891461124));
#62407=CARTESIAN_POINT('Ctrl Pts',(-4.59593939908791,1.83873333317766,57.1171094001944));
#62408=CARTESIAN_POINT('Ctrl Pts',(-4.82775332951413,1.25931120769625,57.1372994485773));
#62409=CARTESIAN_POINT('Ctrl Pts',(-4.93915674573565,0.631715508347176,
57.1574894969603));
#62410=CARTESIAN_POINT('Ctrl Pts',(-4.93573111423024,0.00295138605979709,
57.1776795453432));
#62411=CARTESIAN_POINT('Origin',(0.,0.,16.));
#62412=CARTESIAN_POINT('',(-4.9373129524182,-0.00377529733612325,58.3223204546568));
#62413=CARTESIAN_POINT('',(-4.93796046055574,-0.00400002009900308,58.1776795453432));
#62414=CARTESIAN_POINT('',(-4.942,-6.05220448138622E-16,16.));
#62415=CARTESIAN_POINT('Ctrl Pts',(-4.9373129524182,-0.00377529733612325,
58.3223204546568));
#62416=CARTESIAN_POINT('Ctrl Pts',(-4.92952693668152,1.09003472006405,58.2871691720943));
#62417=CARTESIAN_POINT('Ctrl Pts',(-4.57107143779465,2.18847891881712,58.2520178895318));
#62418=CARTESIAN_POINT('Ctrl Pts',(-3.90268743507911,3.04509922980021,58.2168666069693));
#62419=CARTESIAN_POINT('Ctrl Pts',(-2.89643535351957,4.33474106373227,58.1639463528874));
#62420=CARTESIAN_POINT('Ctrl Pts',(-1.18772099090388,5.07628177847635,58.1110260988054));
#62421=CARTESIAN_POINT('Ctrl Pts',(0.441521863755048,4.93038101763753,58.0581058447234));
#62422=CARTESIAN_POINT('Ctrl Pts',(2.07076471841393,4.78448025679871,58.0051855906414));
#62423=CARTESIAN_POINT('Ctrl Pts',(3.62053606511612,3.75113802037702,57.9522653365595));
#62424=CARTESIAN_POINT('Ctrl Pts',(4.38163686641958,2.30322749768385,57.8993450824775));
#62425=CARTESIAN_POINT('Ctrl Pts',(5.14273766772306,0.855316974990642,57.8464248283956));
#62426=CARTESIAN_POINT('Ctrl Pts',(5.11516792362781,-1.00716183397399,57.7935045743136));
#62427=CARTESIAN_POINT('Ctrl Pts',(4.31154397009623,-2.43191018115001,57.7405843202316));
#62428=CARTESIAN_POINT('Ctrl Pts',(3.50792001656464,-3.85665852832602,57.6876640661497));
#62429=CARTESIAN_POINT('Ctrl Pts',(1.92824185359667,-4.84367641371333,57.6347438120677));
#62430=CARTESIAN_POINT('Ctrl Pts',(0.295394334515388,-4.94128937853172,
57.5818235579858));
#62431=CARTESIAN_POINT('Ctrl Pts',(-1.33745318456585,-5.03890234335011,
57.5289033039038));
#62432=CARTESIAN_POINT('Ctrl Pts',(-3.02347005976055,-4.24711038759957,
57.4759830498218));
#62433=CARTESIAN_POINT('Ctrl Pts',(-3.99110921895138,-2.92824960303174,
57.4230627957398));
#62434=CARTESIAN_POINT('Ctrl Pts',(-4.60512891022411,-2.09136068211493,
57.3894820153788));
#62435=CARTESIAN_POINT('Ctrl Pts',(-4.9298871379951,-1.04224259902719,57.3559012350179));
#62436=CARTESIAN_POINT('Ctrl Pts',(-4.93623902664834,0.00326946414225537,
57.3223204546569));
#62437=CARTESIAN_POINT('Ctrl Pts',(-4.93573111423024,0.00295138605979709,
57.1776795453432));
#62438=CARTESIAN_POINT('Ctrl Pts',(-4.93017780293081,-1.01634181563486,
57.2104097510422));
#62439=CARTESIAN_POINT('Ctrl Pts',(-4.62285556832308,-2.03870561435216,
57.2431399567412));
#62440=CARTESIAN_POINT('Ctrl Pts',(-4.03754280040764,-2.86388675849859,
57.2758701624402));
#62441=CARTESIAN_POINT('Ctrl Pts',(-3.09117232292437,-4.19809150543631,
57.3287904165222));
#62442=CARTESIAN_POINT('Ctrl Pts',(-1.41806634007047,-5.01681238170109,
57.3817106706042));
#62443=CARTESIAN_POINT('Ctrl Pts',(0.216136297556334,-4.94539021023678,
57.4346309246861));
#62444=CARTESIAN_POINT('Ctrl Pts',(1.85033893518309,-4.87396803877247,57.4875511787681));
#62445=CARTESIAN_POINT('Ctrl Pts',(3.4456382275827,-3.91240281957913,57.5404714328501));
#62446=CARTESIAN_POINT('Ctrl Pts',(4.27200085402752,-2.50072148265561,57.593391686932));
#62447=CARTESIAN_POINT('Ctrl Pts',(5.0983634804724,-1.08904014573198,57.646311941014));
#62448=CARTESIAN_POINT('Ctrl Pts',(5.15578944096228,0.772757308922017,57.699232195096));
#62449=CARTESIAN_POINT('Ctrl Pts',(4.41799973892759,2.23268393138458,57.7521524491779));
#62450=CARTESIAN_POINT('Ctrl Pts',(3.68021003689295,3.69261055384702,57.8050727032599));
#62451=CARTESIAN_POINT('Ctrl Pts',(2.14720467233395,4.75066634411819,57.8579929573418));
#62452=CARTESIAN_POINT('Ctrl Pts',(0.520510313201973,4.9226688132026,57.9109132114238));
#62453=CARTESIAN_POINT('Ctrl Pts',(-1.1061840459301,5.09467128228702,57.9638334655058));
#62454=CARTESIAN_POINT('Ctrl Pts',(-2.8265673996351,4.38062043018456,58.0167537195877));
#62455=CARTESIAN_POINT('Ctrl Pts',(-3.85336605036076,3.10727683230095,58.0696739736697));
#62456=CARTESIAN_POINT('Ctrl Pts',(-4.5519012154505,2.2410161688934,58.1056758308942));
#62457=CARTESIAN_POINT('Ctrl Pts',(-4.92943605312281,1.11590730173118,58.1416776881187));
#62458=CARTESIAN_POINT('Ctrl Pts',(-4.93796046055574,-0.00400002009900308,
58.1776795453432));
#62459=CARTESIAN_POINT('Origin',(0.,0.,16.));
#62460=CARTESIAN_POINT('',(-4.94980236868244,-0.00111614563719775,59.3223204546569));
#62461=CARTESIAN_POINT('',(-4.95000952859661,-0.000636468299896517,59.1776795453432));
#62462=CARTESIAN_POINT('',(-4.942,-6.05220448138622E-16,16.));
#62463=CARTESIAN_POINT('Ctrl Pts',(-4.94980236868244,-0.00111614563719775,
59.3223204546569));
#62464=CARTESIAN_POINT('Ctrl Pts',(-4.94498060556177,1.57441454729254,59.2713573632528));
#62465=CARTESIAN_POINT('Ctrl Pts',(-4.12744131963774,3.15424986030506,59.2203942718487));
#62466=CARTESIAN_POINT('Ctrl Pts',(-2.83642564175097,4.05688157506129,59.1694311804446));
#62467=CARTESIAN_POINT('Ctrl Pts',(-1.49583040281886,4.99417753516308,59.1165109263627));
#62468=CARTESIAN_POINT('Ctrl Pts',(0.355305856754859,5.20125711678249,59.0635906722807));
#62469=CARTESIAN_POINT('Ctrl Pts',(1.86987491274258,4.58335754070639,59.0106704181987));
#62470=CARTESIAN_POINT('Ctrl Pts',(3.38444396873026,3.96545796463031,58.9577501641168));
#62471=CARTESIAN_POINT('Ctrl Pts',(4.56244582113197,2.52257923085877,58.9048299100348));
#62472=CARTESIAN_POINT('Ctrl Pts',(4.86480883102114,0.915004684618019,58.8519096559529));
#62473=CARTESIAN_POINT('Ctrl Pts',(5.16717184091031,-0.692569861622737,
58.7989894018709));
#62474=CARTESIAN_POINT('Ctrl Pts',(4.59389600828695,-2.46484022033272,58.7460691477889));
#62475=CARTESIAN_POINT('Ctrl Pts',(3.40732110962866,-3.59078840801476,58.6931488937069));
#62476=CARTESIAN_POINT('Ctrl Pts',(2.22074621097036,-4.7167365956968,58.640228639625));
#62477=CARTESIAN_POINT('Ctrl Pts',(0.42087224627713,-5.1963626123509,58.5873083855431));
#62478=CARTESIAN_POINT('Ctrl Pts',(-1.16865096927437,-4.81018226757243,
58.5343881314611));
#62479=CARTESIAN_POINT('Ctrl Pts',(-2.75817418482588,-4.42400192279397,
58.4814678773791));
#62480=CARTESIAN_POINT('Ctrl Pts',(-4.13734665123566,-3.17201521658293,
58.4285476232971));
#62481=CARTESIAN_POINT('Ctrl Pts',(-4.67503798418886,-1.62715038691743,
58.3756273692152));
#62482=CARTESIAN_POINT('Ctrl Pts',(-4.85557797114165,-1.10843293863767,
58.3578583976957));
#62483=CARTESIAN_POINT('Ctrl Pts',(-4.94124878297087,-0.556696204625704,
58.3400894261763));
#62484=CARTESIAN_POINT('Ctrl Pts',(-4.9373129524182,-0.00377529733612325,
58.3223204546568));
#62485=CARTESIAN_POINT('Ctrl Pts',(-4.93796046055574,-0.00400002009900308,
58.1776795453432));
#62486=CARTESIAN_POINT('Ctrl Pts',(-4.94196634578065,-0.530279439411995,
58.1945979422007));
#62487=CARTESIAN_POINT('Ctrl Pts',(-4.86448168129051,-1.05541017361004,
58.2115163390581));
#62488=CARTESIAN_POINT('Ctrl Pts',(-4.70052410203468,-1.55198981852916,
58.2284347359156));
#62489=CARTESIAN_POINT('Ctrl Pts',(-4.18766955523667,-3.10527652781102,
58.2813549899975));
#62490=CARTESIAN_POINT('Ctrl Pts',(-2.82874651389436,-4.37921360271005,
58.3342752440795));
#62491=CARTESIAN_POINT('Ctrl Pts',(-1.24561891614835,-4.79082798129515,
58.3871954981615));
#62492=CARTESIAN_POINT('Ctrl Pts',(0.337508681597706,-5.20244235988026,
58.4401157522434));
#62493=CARTESIAN_POINT('Ctrl Pts',(2.14484083574746,-4.75173404215139,58.4930360063254));
#62494=CARTESIAN_POINT('Ctrl Pts',(3.34931474972224,-3.6449540378337,58.5459562604074));
#62495=CARTESIAN_POINT('Ctrl Pts',(4.55378866369698,-2.53817403351603,58.5988765144893));
#62496=CARTESIAN_POINT('Ctrl Pts',(5.15540433749678,-0.775322342609574,
58.6517967685713));
#62497=CARTESIAN_POINT('Ctrl Pts',(4.87885325049583,0.836893177623885,58.7047170226533));
#62498=CARTESIAN_POINT('Ctrl Pts',(4.60230216349487,2.44910869785739,58.7576372767352));
#62499=CARTESIAN_POINT('Ctrl Pts',(3.44758431569312,3.91068804741789,58.8105575308172));
#62500=CARTESIAN_POINT('Ctrl Pts',(1.94311622990263,4.5527901936852,58.8634777848992));
#62501=CARTESIAN_POINT('Ctrl Pts',(0.438648144112182,5.19489233995249,58.9163980389811));
#62502=CARTESIAN_POINT('Ctrl Pts',(-1.41557017966698,5.01751728292666,58.969318293063));
#62503=CARTESIAN_POINT('Ctrl Pts',(-2.77102011755545,4.10183455769855,59.022238547145));
#62504=CARTESIAN_POINT('Ctrl Pts',(-4.09812694403132,3.205299199536,59.0740522132111));
#62505=CARTESIAN_POINT('Ctrl Pts',(-4.94710627363632,1.60101008771938,59.1258658792772));
#62506=CARTESIAN_POINT('Ctrl Pts',(-4.95000952859661,-0.000636468299896517,
59.1776795453432));
#62507=CARTESIAN_POINT('Origin',(0.,0.,16.));
#62508=CARTESIAN_POINT('',(-4.9405850371911,0.0044815032353801,60.3223204546569));
#62509=CARTESIAN_POINT('',(-4.93981933179839,0.00440230787564107,60.1776795453432));
#62510=CARTESIAN_POINT('',(-4.942,-6.05220448138622E-16,16.));
#62511=CARTESIAN_POINT('Ctrl Pts',(-4.9405850371911,0.0044815032353801,
60.3223204546569));
#62512=CARTESIAN_POINT('Ctrl Pts',(-4.94441025446321,0.434877172261215,
60.3084658084932));
#62513=CARTESIAN_POINT('Ctrl Pts',(-4.89283730030809,0.864370712953886,
60.2946111623296));
#62514=CARTESIAN_POINT('Ctrl Pts',(-4.78226597761638,1.27809649658665,60.2807565161659));
#62515=CARTESIAN_POINT('Ctrl Pts',(-4.3599193928029,2.85839478291331,60.2278362620839));
#62516=CARTESIAN_POINT('Ctrl Pts',(-3.07679122526311,4.20864272692144,60.1749160080019));
#62517=CARTESIAN_POINT('Ctrl Pts',(-1.52006052129332,4.71094624750269,60.12199575392));
#62518=CARTESIAN_POINT('Ctrl Pts',(0.0366701826763779,5.21324976808391,
60.069075499838));
#62519=CARTESIAN_POINT('Ctrl Pts',(1.867003423076,4.86760886523835,60.016155245756));
#62520=CARTESIAN_POINT('Ctrl Pts',(3.1333507549704,3.83219409497753,59.9632349916741));
#62521=CARTESIAN_POINT('Ctrl Pts',(4.39969808686486,2.79677932471666,59.9103147375921));
#62522=CARTESIAN_POINT('Ctrl Pts',(5.102059510254,1.07159068704033,59.8573944835102));
#62523=CARTESIAN_POINT('Ctrl Pts',(4.91902371084035,-0.55389914916401,59.8044742294282));
#62524=CARTESIAN_POINT('Ctrl Pts',(4.73598791142671,-2.1793889853683,59.7515539753462));
#62525=CARTESIAN_POINT('Ctrl Pts',(3.66755488921043,-3.70518002010068,59.6986337212642));
#62526=CARTESIAN_POINT('Ctrl Pts',(2.20265591301344,-4.43304697292067,59.6457134671823));
#62527=CARTESIAN_POINT('Ctrl Pts',(0.737756936816448,-5.16091392574066,
59.5927932131003));
#62528=CARTESIAN_POINT('Ctrl Pts',(-1.12360799336121,-5.09085679664823,
59.5398729590184));
#62529=CARTESIAN_POINT('Ctrl Pts',(-2.52964985740424,-4.25493479787751,
59.4869527049364));
#62530=CARTESIAN_POINT('Ctrl Pts',(-3.93569172144728,-3.41901279910679,
59.4340324508545));
#62531=CARTESIAN_POINT('Ctrl Pts',(-4.88641051935565,-1.8172259306578,59.3811121967725));
#62532=CARTESIAN_POINT('Ctrl Pts',(-4.94674280916461,-0.182576327141242,
59.3281919426905));
#62533=CARTESIAN_POINT('Ctrl Pts',(-4.94897409296954,-0.122121681733242,
59.3262347800127));
#62534=CARTESIAN_POINT('Ctrl Pts',(-4.94998754141356,-0.0616220879792628,
59.3242776173348));
#62535=CARTESIAN_POINT('Ctrl Pts',(-4.94980236868244,-0.00111614563719775,
59.3223204546569));
#62536=CARTESIAN_POINT('Ctrl Pts',(-4.95000952859661,-0.000636468299896517,
59.1776795453432));
#62537=CARTESIAN_POINT('Ctrl Pts',(-4.95007153361169,-0.0348429435249772,
59.1787861333591));
#62538=CARTESIAN_POINT('Ctrl Pts',(-4.94974762270576,-0.0690482134159459,
59.179892721375));
#62539=CARTESIAN_POINT('Ctrl Pts',(-4.94903421151526,-0.103245357661693,
59.1809993093909));
#62540=CARTESIAN_POINT('Ctrl Pts',(-4.9149168155888,-1.73865215436347,59.2339195634729));
#62541=CARTESIAN_POINT('Ctrl Pts',(-3.99000047173805,-3.35547535433661,
59.2868398175548));
#62542=CARTESIAN_POINT('Ctrl Pts',(-2.59754102487793,-4.21383196801951,
59.3397600716368));
#62543=CARTESIAN_POINT('Ctrl Pts',(-1.20508157801781,-5.07218858170242,
59.3926803257188));
#62544=CARTESIAN_POINT('Ctrl Pts',(0.654920971851715,-5.17207860909511,
59.4456005798008));
#62545=CARTESIAN_POINT('Ctrl Pts',(2.13130105065146,-4.46779084807236,59.4985208338827));
#62546=CARTESIAN_POINT('Ctrl Pts',(3.60768112945116,-3.76350308704963,59.5514410879647));
#62547=CARTESIAN_POINT('Ctrl Pts',(4.70043873718116,-2.25503753761151,59.6043613420466));
#62548=CARTESIAN_POINT('Ctrl Pts',(4.90951130318629,-0.632691073520989,
59.6572815961286));
#62549=CARTESIAN_POINT('Ctrl Pts',(5.11858386919144,0.98965539056958,59.7102018502105));
#62550=CARTESIAN_POINT('Ctrl Pts',(4.44397139347178,2.7258827693125,59.7631221042925));
#62551=CARTESIAN_POINT('Ctrl Pts',(3.19438684806975,3.78146689731725,59.8160423583745));
#62552=CARTESIAN_POINT('Ctrl Pts',(1.94480230266778,4.83705102532194,59.8689626124565));
#62553=CARTESIAN_POINT('Ctrl Pts',(0.120245687583507,5.21199190258845,59.9218828665384));
#62554=CARTESIAN_POINT('Ctrl Pts',(-1.44433802421679,4.7347108573205,59.9748031206203));
#62555=CARTESIAN_POINT('Ctrl Pts',(-3.00892173601718,4.25742981205253,60.0277233747023));
#62556=CARTESIAN_POINT('Ctrl Pts',(-4.31353254453361,2.92792684424999,60.0806436287843));
#62557=CARTESIAN_POINT('Ctrl Pts',(-4.7611606188609,1.35460281707783,60.1335638828663));
#62558=CARTESIAN_POINT('Ctrl Pts',(-4.88554531419032,0.917415247758462,
60.1482691036919));
#62559=CARTESIAN_POINT('Ctrl Pts',(-4.94375845579816,0.461401140068047,
60.1629743245176));
#62560=CARTESIAN_POINT('Ctrl Pts',(-4.93981933179839,0.00440230787564107,
60.1776795453432));
#62561=CARTESIAN_POINT('Origin',(0.,0.,16.));
#62562=CARTESIAN_POINT('',(-4.93439206002794,-0.00160550854955477,61.3223204546568));
#62563=CARTESIAN_POINT('',(-4.93468237204831,-0.00200522711461992,61.1776795453432));
#62564=CARTESIAN_POINT('',(-4.942,-6.05220448138622E-16,16.));
#62565=CARTESIAN_POINT('Ctrl Pts',(-4.93439206002794,-0.00160550854955477,
61.3223204546568));
#62566=CARTESIAN_POINT('Ctrl Pts',(-4.93169731118072,0.922902919227787,
61.2926539996516));
#62567=CARTESIAN_POINT('Ctrl Pts',(-4.68258000927622,1.84875941269167,61.2629875446464));
#62568=CARTESIAN_POINT('Ctrl Pts',(-4.19611032092476,2.62607248755302,61.2333210896412));
#62569=CARTESIAN_POINT('Ctrl Pts',(-3.3283254943857,4.01267582171134,61.1804008355592));
#62570=CARTESIAN_POINT('Ctrl Pts',(-1.7052638805986,4.92660054644685,61.1274805814773));
#62571=CARTESIAN_POINT('Ctrl Pts',(-0.0696632625637214,4.94962074962347,
61.0745603273953));
#62572=CARTESIAN_POINT('Ctrl Pts',(1.56593735547125,4.97264095280009,61.0216400733134));
#62573=CARTESIAN_POINT('Ctrl Pts',(3.21407697775393,4.10475663441781,60.9687198192314));
#62574=CARTESIAN_POINT('Ctrl Pts',(4.12054174158777,2.74312491350412,60.9157995651494));
#62575=CARTESIAN_POINT('Ctrl Pts',(5.02700650542156,1.3814931925905,60.8628793110674));
#62576=CARTESIAN_POINT('Ctrl Pts',(5.19179641080646,-0.473885930854428,
60.8099590569854));
#62577=CARTESIAN_POINT('Ctrl Pts',(4.53950108025175,-1.97396263329564,60.7570388029035));
#62578=CARTESIAN_POINT('Ctrl Pts',(3.88720574969703,-3.47403933573684,60.7041185488216));
#62579=CARTESIAN_POINT('Ctrl Pts',(2.41782518320256,-4.61881361717445,60.6511982947396));
#62580=CARTESIAN_POINT('Ctrl Pts',(0.803770369403307,-4.88441928262956,
60.5982780406577));
#62581=CARTESIAN_POINT('Ctrl Pts',(-0.810284444395997,-5.15002494808468,
60.5453577865757));
#62582=CARTESIAN_POINT('Ctrl Pts',(-2.56901350550008,-4.53646199755745,
60.4924375324937));
#62583=CARTESIAN_POINT('Ctrl Pts',(-3.66759553500858,-3.32450620797124,
60.4395172784117));
#62584=CARTESIAN_POINT('Ctrl Pts',(-4.47856622242051,-2.42984327576097,
60.4004516704934));
#62585=CARTESIAN_POINT('Ctrl Pts',(-4.92979916533343,-1.20909466877745,
60.3613860625752));
#62586=CARTESIAN_POINT('Ctrl Pts',(-4.9405850371911,0.0044815032353801,
60.3223204546569));
#62587=CARTESIAN_POINT('Ctrl Pts',(-4.93981933179839,0.00440230787564107,
60.1776795453432));
#62588=CARTESIAN_POINT('Ctrl Pts',(-4.9295825759933,-1.18321845466868,60.2158945785995));
#62589=CARTESIAN_POINT('Ctrl Pts',(-4.49960389811683,-2.3774895002097,60.2541096118559));
#62590=CARTESIAN_POINT('Ctrl Pts',(-3.72042358357856,-3.26527909823641,
60.2923246451122));
#62591=CARTESIAN_POINT('Ctrl Pts',(-2.64141313383085,-4.49469189983651,
60.3452448991941));
#62592=CARTESIAN_POINT('Ctrl Pts',(-0.892746894197383,-5.13637241649503,
60.3981651532761));
#62593=CARTESIAN_POINT('Ctrl Pts',(0.72535875721281,-4.89667784359578,60.451085407358));
#62594=CARTESIAN_POINT('Ctrl Pts',(2.34346440862305,-4.65698327069652,60.50400566144));
#62595=CARTESIAN_POINT('Ctrl Pts',(3.83100947181002,-3.53591360823934,60.556925915522));
#62596=CARTESIAN_POINT('Ctrl Pts',(4.50727060703144,-2.0464874555241,60.6098461696039));
#62597=CARTESIAN_POINT('Ctrl Pts',(5.18353174225287,-0.557061302808867,
60.6627664236859));
#62598=CARTESIAN_POINT('Ctrl Pts',(5.04850894950886,1.30072134016443,60.7156866777678));
#62599=CARTESIAN_POINT('Ctrl Pts',(4.16399072092151,2.67671076261644,60.7686069318498));
#62600=CARTESIAN_POINT('Ctrl Pts',(3.27947249233419,4.0527001850684,60.8215271859318));
#62601=CARTESIAN_POINT('Ctrl Pts',(1.64545882790348,4.94689638699909,60.8744474400138));
#62602=CARTESIAN_POINT('Ctrl Pts',(0.00969933627160482,4.95010152961563,
60.9273676940957));
#62603=CARTESIAN_POINT('Ctrl Pts',(-1.62606015536036,4.95330667223218,60.9802879481777));
#62604=CARTESIAN_POINT('Ctrl Pts',(-3.26356547419351,4.06552075553457,61.0332082022597));
#62605=CARTESIAN_POINT('Ctrl Pts',(-4.15346917720423,2.69300817389058,61.0861284563416));
#62606=CARTESIAN_POINT('Ctrl Pts',(-4.66664165108668,1.90153413622322,61.1166454860088));
#62607=CARTESIAN_POINT('Ctrl Pts',(-4.93120852346023,0.948870286286938,
61.147162515676));
#62608=CARTESIAN_POINT('Ctrl Pts',(-4.93468237204831,-0.00200522711461992,
61.1776795453432));
#62609=CARTESIAN_POINT('Origin',(0.,0.,16.));
#62610=CARTESIAN_POINT('',(-4.94646539259968,-0.00363051697945815,62.3223204546568));
#62611=CARTESIAN_POINT('',(-4.94715367607242,-0.003331217148393,62.1776795453432));
#62612=CARTESIAN_POINT('',(-4.942,-6.05220448138622E-16,16.));
#62613=CARTESIAN_POINT('Ctrl Pts',(-4.94646539259968,-0.00363051697945815,
62.3223204546568));
#62614=CARTESIAN_POINT('Ctrl Pts',(-4.93485651568824,1.40483737949782,62.2768421908101));
#62615=CARTESIAN_POINT('Ctrl Pts',(-4.3027525120455,2.82241015727549,62.2313639269634));
#62616=CARTESIAN_POINT('Ctrl Pts',(-3.23996042330606,3.74249315171913,62.1858856631166));
#62617=CARTESIAN_POINT('Ctrl Pts',(-2.00325473986379,4.81313705330919,62.1329654090346));
#62618=CARTESIAN_POINT('Ctrl Pts',(-0.183373993763468,5.2101527640882,62.0800451549526));
#62619=CARTESIAN_POINT('Ctrl Pts',(1.3868765910888,4.75185983130228,62.0271249008706));
#62620=CARTESIAN_POINT('Ctrl Pts',(2.95712717594107,4.29356689851636,61.9742046467886));
#62621=CARTESIAN_POINT('Ctrl Pts',(4.2777475995453,2.97996532216552,61.9212843927068));
#62622=CARTESIAN_POINT('Ctrl Pts',(4.74440178662215,1.4121792458292,61.8683641386248));
#62623=CARTESIAN_POINT('Ctrl Pts',(5.21105597369902,-0.155606830507172,
61.8154438845429));
#62624=CARTESIAN_POINT('Ctrl Pts',(4.82374392424848,-1.97757740682905,61.7625236304608));
#62625=CARTESIAN_POINT('Ctrl Pts',(3.75970554739938,-3.21997092100356,61.7096033763788));
#62626=CARTESIAN_POINT('Ctrl Pts',(2.69566717055032,-4.46236443517805,61.6566831222968));
#62627=CARTESIAN_POINT('Ctrl Pts',(0.954902466302742,-5.12518088720521,
61.603762868215));
#62628=CARTESIAN_POINT('Ctrl Pts',(-0.665988050504544,-4.90510534564135,
61.550842614133));
#62629=CARTESIAN_POINT('Ctrl Pts',(-2.28687856731188,-4.68502980407749,
61.4979223600511));
#62630=CARTESIAN_POINT('Ctrl Pts',(-3.78789489667891,-3.58206226892256,
61.4450021059691));
#62631=CARTESIAN_POINT('Ctrl Pts',(-4.4821490417169,-2.10093752955449,61.3920818518871));
#62632=CARTESIAN_POINT('Ctrl Pts',(-4.78721270168923,-1.45011342271034,
61.3688280528103));
#62633=CARTESIAN_POINT('Ctrl Pts',(-4.9365043160506,-0.726273596479458,
61.3455742537336));
#62634=CARTESIAN_POINT('Ctrl Pts',(-4.93439206002794,-0.00160550854955477,
61.3223204546568));
#62635=CARTESIAN_POINT('Ctrl Pts',(-4.93468237204831,-0.00200522711461992,
61.1776795453432));
#62636=CARTESIAN_POINT('Ctrl Pts',(-4.93723260089922,-0.700063909415997,
61.200082769758));
#62637=CARTESIAN_POINT('Ctrl Pts',(-4.79907061241107,-1.39715879423438,
61.2224859941727));
#62638=CARTESIAN_POINT('Ctrl Pts',(-4.51525583033475,-2.02880852158482,
61.2448892185875));
#62639=CARTESIAN_POINT('Ctrl Pts',(-3.84483669326632,-3.520873388826,61.2978094726695));
#62640=CARTESIAN_POINT('Ctrl Pts',(-2.36169633194117,-4.64776387671811,
61.3507297267514));
#62641=CARTESIAN_POINT('Ctrl Pts',(-0.744542427257826,-4.89379768734264,
61.4036499808334));
#62642=CARTESIAN_POINT('Ctrl Pts',(0.872611477425563,-5.13983149796717,
61.4565702349153));
#62643=CARTESIAN_POINT('Ctrl Pts',(2.62377892546721,-4.50500863132408,61.5094904889973));
#62644=CARTESIAN_POINT('Ctrl Pts',(3.7075989475901,-3.27983372664773,61.5624107430792));
#62645=CARTESIAN_POINT('Ctrl Pts',(4.79141896971299,-2.05465882197138,61.6153309971612));
#62646=CARTESIAN_POINT('Ctrl Pts',(5.20789156591715,-0.23913187926188,61.6682512512432));
#62647=CARTESIAN_POINT('Ctrl Pts',(4.76643251551905,1.33593424450079,61.7211715053252));
#62648=CARTESIAN_POINT('Ctrl Pts',(4.32497346512095,2.91100036826346,61.7740917594072));
#62649=CARTESIAN_POINT('Ctrl Pts',(3.02558276812051,4.24560567307922,61.8270120134891));
#62650=CARTESIAN_POINT('Ctrl Pts',(1.46288145266801,4.72901438843942,61.879932267571));
#62651=CARTESIAN_POINT('Ctrl Pts',(-0.099819862784441,5.2124231037996,61.932852521653));
#62652=CARTESIAN_POINT('Ctrl Pts',(-1.92583179668899,4.84463522970427,61.985772775735));
#62653=CARTESIAN_POINT('Ctrl Pts',(-3.17954339996051,3.79395611445292,62.038693029817));
#62654=CARTESIAN_POINT('Ctrl Pts',(-4.27710053403159,2.87414301265627,62.0850218683257));
#62655=CARTESIAN_POINT('Ctrl Pts',(-4.93604317278978,1.43095786114934,62.1313507068344));
#62656=CARTESIAN_POINT('Ctrl Pts',(-4.94715367607242,-0.003331217148393,
62.1776795453432));
#62657=CARTESIAN_POINT('Origin',(0.,0.,16.));
#62658=CARTESIAN_POINT('',(-4.94566965389892,0.00391030538274315,63.3223204546568));
#62659=CARTESIAN_POINT('',(-4.94490839420487,0.00412192395711707,63.1776795453432));
#62660=CARTESIAN_POINT('',(-4.942,-6.05220448138622E-16,16.));
#62661=CARTESIAN_POINT('Ctrl Pts',(-4.94566965389892,0.00391030538274314,
63.3223204546568));
#62662=CARTESIAN_POINT('Ctrl Pts',(-4.94791640205867,0.263233220344943,
63.3139506360505));
#62663=CARTESIAN_POINT('Ctrl Pts',(-4.92928016281063,0.522232554885722,
63.3055808174441));
#62664=CARTESIAN_POINT('Ctrl Pts',(-4.88863316854879,0.777730209403516,
63.2972109988377));
#62665=CARTESIAN_POINT('Ctrl Pts',(-4.63163246576532,2.39317750047789,63.2442907447558));
#62666=CARTESIAN_POINT('Ctrl Pts',(-3.49470467070217,3.86863762987662,63.1913704906738));
#62667=CARTESIAN_POINT('Ctrl Pts',(-1.99812530633611,4.52891750812856,63.1384502365919));
#62668=CARTESIAN_POINT('Ctrl Pts',(-0.501545941970182,5.18919738638045,
63.0855299825099));
#62669=CARTESIAN_POINT('Ctrl Pts',(1.35468499169859,5.0342970134857,63.0326097284279));
#62670=CARTESIAN_POINT('Ctrl Pts',(2.72112786976736,4.1351011658277,62.979689474346));
#62671=CARTESIAN_POINT('Ctrl Pts',(4.08757074783617,3.23590531816966,62.926769220264));
#62672=CARTESIAN_POINT('Ctrl Pts',(4.96422557030495,1.59241399574832,62.8738489661821));
#62673=CARTESIAN_POINT('Ctrl Pts',(4.94992170152689,-0.0432860717482803,
62.8209287121001));
#62674=CARTESIAN_POINT('Ctrl Pts',(4.93561783274882,-1.67898613924493,62.7680084580182));
#62675=CARTESIAN_POINT('Ctrl Pts',(4.03035527272386,-3.30689495181684,62.7150882039362));
#62676=CARTESIAN_POINT('Ctrl Pts',(2.64839599472191,-4.18205657427003,62.6621679498542));
#62677=CARTESIAN_POINT('Ctrl Pts',(1.26643671671996,-5.05721819672321,62.6092476957723));
#62678=CARTESIAN_POINT('Ctrl Pts',(-0.592219279258987,-5.17963262905766,
62.5563274416903));
#62679=CARTESIAN_POINT('Ctrl Pts',(-2.07702262276162,-4.49328115743837,
62.5034071876083));
#62680=CARTESIAN_POINT('Ctrl Pts',(-3.56182596626416,-3.80692968581911,
62.4504869335263));
#62681=CARTESIAN_POINT('Ctrl Pts',(-4.67277665729038,-2.31181231024634,
62.3975666794443));
#62682=CARTESIAN_POINT('Ctrl Pts',(-4.9014866924115,-0.692117576259364,
62.3446464253624));
#62683=CARTESIAN_POINT('Ctrl Pts',(-4.93364938470368,-0.464345570938786,
62.3372044351272));
#62684=CARTESIAN_POINT('Ctrl Pts',(-4.94836505061889,-0.234109947053592,
62.329762444892));
#62685=CARTESIAN_POINT('Ctrl Pts',(-4.94646539259968,-0.00363051697945815,
62.3223204546568));
#62686=CARTESIAN_POINT('Ctrl Pts',(-4.94715367607242,-0.003331217148393,
62.1776795453432));
#62687=CARTESIAN_POINT('Ctrl Pts',(-4.94873441814843,-0.207394078888273,
62.1842709609164));
#62688=CARTESIAN_POINT('Ctrl Pts',(-4.93720170764577,-0.4112768658406,62.1908623764896));
#62689=CARTESIAN_POINT('Ctrl Pts',(-4.91195301252751,-0.613446683379284,
62.1974537920628));
#62690=CARTESIAN_POINT('Ctrl Pts',(-4.70923974918446,-2.23660000955276,
62.2503740461448));
#62691=CARTESIAN_POINT('Ctrl Pts',(-3.6224019498598,-3.74933630549224,62.3032943002267));
#62692=CARTESIAN_POINT('Ctrl Pts',(-2.14879319047093,-4.45940433860991,
62.3562145543087));
#62693=CARTESIAN_POINT('Ctrl Pts',(-0.675184431082104,-5.16947237172755,
62.4091348083907));
#62694=CARTESIAN_POINT('Ctrl Pts',(1.18519528837092,-5.07687214202343,62.4620550624727));
#62695=CARTESIAN_POINT('Ctrl Pts',(2.58100779524721,-4.22397892886556,62.5149753165546));
#62696=CARTESIAN_POINT('Ctrl Pts',(3.97682030212355,-3.37108571570767,62.5678955706366));
#62697=CARTESIAN_POINT('Ctrl Pts',(4.90806559642314,-1.75789951909599,62.6208158247185));
#62698=CARTESIAN_POINT('Ctrl Pts',(4.94859160884553,-0.122638980307035,
62.6737360788005));
#62699=CARTESIAN_POINT('Ctrl Pts',(4.98911762126792,1.51262155848192,62.7266563328825));
#62700=CARTESIAN_POINT('Ctrl Pts',(4.13892435181312,3.16995643944814,62.7795765869645));
#62701=CARTESIAN_POINT('Ctrl Pts',(2.78707322532942,4.09094390908492,62.8324968410464));
#62702=CARTESIAN_POINT('Ctrl Pts',(1.43522209884579,5.01193137872164,62.8854170951284));
#62703=CARTESIAN_POINT('Ctrl Pts',(-0.418286884666658,5.19657143702902,
62.9383373492103));
#62704=CARTESIAN_POINT('Ctrl Pts',(-1.92525970626815,4.56036997337358,62.9912576032922));
#62705=CARTESIAN_POINT('Ctrl Pts',(-3.43223252786973,3.92416850971811,63.0441778573742));
#62706=CARTESIAN_POINT('Ctrl Pts',(-4.59266918756032,2.46712552409973,63.0970981114562));
#62707=CARTESIAN_POINT('Ctrl Pts',(-4.87553614686583,0.856006139716171,
63.1500183655382));
#62708=CARTESIAN_POINT('Ctrl Pts',(-4.9248205778018,0.57529784411246,63.1592387588066));
#62709=CARTESIAN_POINT('Ctrl Pts',(-4.94746485856309,0.289912292218248,
63.1684591520749));
#62710=CARTESIAN_POINT('Ctrl Pts',(-4.94490839420487,0.00412192395711708,
63.1776795453432));
#62711=CARTESIAN_POINT('Origin',(0.,0.,16.));
#62712=CARTESIAN_POINT('',(-4.93415080838549,0.00115309545102804,64.3223204546568));
#62713=CARTESIAN_POINT('',(-4.9340004404197,0.000727385793248169,64.1776795453432));
#62714=CARTESIAN_POINT('',(-4.942,-6.05220448138622E-16,16.));
#62715=CARTESIAN_POINT('Ctrl Pts',(-4.93415080838549,0.00115309545102804,
64.3223204546568));
#62716=CARTESIAN_POINT('Ctrl Pts',(-4.93572402472308,0.754827492624239,
64.2981388272089));
#62717=CARTESIAN_POINT('Ctrl Pts',(-4.77374496051519,1.5078605887699,64.273957199761));
#62718=CARTESIAN_POINT('Ctrl Pts',(-4.44472183637519,2.17900122361227,64.2497755723131));
#62719=CARTESIAN_POINT('Ctrl Pts',(-3.72467156821878,3.64775815476123,64.1968553182311));
#62720=CARTESIAN_POINT('Ctrl Pts',(-2.20459580691742,4.72430684596657,64.1439350641492));
#62721=CARTESIAN_POINT('Ctrl Pts',(-0.580104436501948,4.91600217432875,
64.0910148100672));
#62722=CARTESIAN_POINT('Ctrl Pts',(1.04438693391362,5.10769750269094,64.0380945559853));
#62723=CARTESIAN_POINT('Ctrl Pts',(2.77329391344336,4.41453946820987,63.9851743019033));
#62724=CARTESIAN_POINT('Ctrl Pts',(3.81544226317875,3.15372777385805,63.9322540478213));
#62725=CARTESIAN_POINT('Ctrl Pts',(4.85759061291414,1.89291607950622,63.8793337937393));
#62726=CARTESIAN_POINT('Ctrl Pts',(5.2129803328552,0.0644507252837223,63.8264135396574));
#62727=CARTESIAN_POINT('Ctrl Pts',(4.71897965939677,-1.49493461711666,63.7734932855754));
#62728=CARTESIAN_POINT('Ctrl Pts',(4.22497898593836,-3.05431995951699,63.7205730314935));
#62729=CARTESIAN_POINT('Ctrl Pts',(2.88158791908043,-4.34462529009514,63.6676527774115));
#62730=CARTESIAN_POINT('Ctrl Pts',(1.30356272822442,-4.77538718313377,63.6147325233296));
#62731=CARTESIAN_POINT('Ctrl Pts',(-0.274462462631595,-5.2061490761724,
63.5618122692476));
#62732=CARTESIAN_POINT('Ctrl Pts',(-2.08712177748574,-4.77736753167153,
63.5088920151656));
#62733=CARTESIAN_POINT('Ctrl Pts',(-3.30491462966089,-3.68525953304616,
63.4559717610837));
#62734=CARTESIAN_POINT('Ctrl Pts',(-4.33010248683659,-2.76587832883282,
63.4114213256081));
#62735=CARTESIAN_POINT('Ctrl Pts',(-4.93371077956384,-1.37640022865803,
63.3668708901324));
#62736=CARTESIAN_POINT('Ctrl Pts',(-4.94566965389892,0.00391030538274314,
63.3223204546568));
#62737=CARTESIAN_POINT('Ctrl Pts',(-4.94490839420487,0.00412192395711708,
63.1776795453432));
#62738=CARTESIAN_POINT('Ctrl Pts',(-4.9327920849133,-1.35037554176026,63.2213794061568));
#62739=CARTESIAN_POINT('Ctrl Pts',(-4.35459996207,-2.71396626059995,63.2650792669704));
#62740=CARTESIAN_POINT('Ctrl Pts',(-3.36357298066115,-3.6318006600574,63.308779127784));
#62741=CARTESIAN_POINT('Ctrl Pts',(-2.16344559623047,-4.74329229229879,
63.361699381866));
#62742=CARTESIAN_POINT('Ctrl Pts',(-0.35789356844863,-5.2010797736329,63.4146196359481));
#62743=CARTESIAN_POINT('Ctrl Pts',(1.22683491911902,-4.7956725609509,63.46753989003));
#62744=CARTESIAN_POINT('Ctrl Pts',(2.81156340668672,-4.39026534826889,63.520460144112));
#62745=CARTESIAN_POINT('Ctrl Pts',(4.17546835404021,-3.12166344157071,63.5733803981938));
#62746=CARTESIAN_POINT('Ctrl Pts',(4.69440602676098,-1.57039844833637,63.6263006522758));
#62747=CARTESIAN_POINT('Ctrl Pts',(5.21334369948175,-0.0191334551020692,
63.6792209063577));
#62748=CARTESIAN_POINT('Ctrl Pts',(4.88731409756984,1.81479462466838,63.7321411604398));
#62749=CARTESIAN_POINT('Ctrl Pts',(3.86551334621209,3.09215229264073,63.7850614145218));
#62750=CARTESIAN_POINT('Ctrl Pts',(2.84371259485431,4.36950996061312,63.8379816686038));
#62751=CARTESIAN_POINT('Ctrl Pts',(1.12614069405063,5.09029721678739,63.8909019226856));
#62752=CARTESIAN_POINT('Ctrl Pts',(-0.501215222432739,4.92467080437148,
63.9438221767676));
#62753=CARTESIAN_POINT('Ctrl Pts',(-2.12857113891606,4.75904439195557,63.9967424308495));
#62754=CARTESIAN_POINT('Ctrl Pts',(-3.66571107107909,3.70700431094953,64.0496626849316));
#62755=CARTESIAN_POINT('Ctrl Pts',(-4.40921630968873,2.24998016991306,64.1025829390136));
#62756=CARTESIAN_POINT('Ctrl Pts',(-4.76090724023141,1.56078236823718,64.1276151411235));
#62757=CARTESIAN_POINT('Ctrl Pts',(-4.93502599479208,0.780971213387874,
64.1526473432333));
#62758=CARTESIAN_POINT('Ctrl Pts',(-4.9340004404197,0.000727385793248169,
64.1776795453432));
#62759=CARTESIAN_POINT('Origin',(0.,0.,16.));
#62760=CARTESIAN_POINT('',(-4.94144181990917,-0.00451754960951789,65.3223204546568));
#62761=CARTESIAN_POINT('',(-4.94223974397651,-0.00450342756324047,65.1776795453432));
#62762=CARTESIAN_POINT('',(-4.942,-6.05220448138622E-16,16.));
#62763=CARTESIAN_POINT('Ctrl Pts',(-4.94144181990917,-0.00451754960951789,
65.3223204546568));
#62764=CARTESIAN_POINT('Ctrl Pts',(-4.93014544737618,1.2373328062097,65.2823270183674));
#62765=CARTESIAN_POINT('Ctrl Pts',(-4.45501720554112,2.48688539619672,65.2423335820779));
#62766=CARTESIAN_POINT('Ctrl Pts',(-3.60889481176119,3.38813765554137,65.2023401457884));
#62767=CARTESIAN_POINT('Ctrl Pts',(-2.48928579044125,4.58069580961582,65.1494198917065));
#62768=CARTESIAN_POINT('Ctrl Pts',(-0.720095544969354,5.16340781391902,
65.0964996376245));
#62769=CARTESIAN_POINT('Ctrl Pts',(0.889067448016765,4.86961575569687,65.0435793835425));
#62770=CARTESIAN_POINT('Ctrl Pts',(2.49823044100288,4.57582369747472,64.9906591294606));
#62771=CARTESIAN_POINT('Ctrl Pts',(3.94736618150317,3.40552757672724,64.9377388753786));
#62772=CARTESIAN_POINT('Ctrl Pts',(4.57332802245098,1.89427277188866,64.8848186212967));
#62773=CARTESIAN_POINT('Ctrl Pts',(5.19928986339881,0.383017967050043,64.8318983672147));
#62774=CARTESIAN_POINT('Ctrl Pts',(5.00207780479406,-1.46919552187978,64.7789781131327));
#62775=CARTESIAN_POINT('Ctrl Pts',(4.07193909661463,-2.81476651406745,64.7260578590508));
#62776=CARTESIAN_POINT('Ctrl Pts',(3.14180038843529,-4.16033750625501,64.6731376049688));
#62777=CARTESIAN_POINT('Ctrl Pts',(1.47873503068148,-4.99926600170063,64.6202173508868));
#62778=CARTESIAN_POINT('Ctrl Pts',(-0.156212869442396,-4.94764550818617,
64.5672970968049));
#62779=CARTESIAN_POINT('Ctrl Pts',(-1.79116076956636,-4.8960250146717,64.5143768427229));
#62780=CARTESIAN_POINT('Ctrl Pts',(-3.39799121206035,-3.95385553219706,
64.461456588641));
#62781=CARTESIAN_POINT('Ctrl Pts',(-4.24139404580168,-2.55228820541339,
64.408536334559));
#62782=CARTESIAN_POINT('Ctrl Pts',(-4.69940845940318,-1.7911595826268,64.379797707925));
#62783=CARTESIAN_POINT('Ctrl Pts',(-4.93228112128365,-0.89455035340317,
64.3510590812909));
#62784=CARTESIAN_POINT('Ctrl Pts',(-4.93415080838549,0.00115309545102804,
64.3223204546568));
#62785=CARTESIAN_POINT('Ctrl Pts',(-4.9340004404197,0.000727385793248169,
64.1776795453432));
#62786=CARTESIAN_POINT('Ctrl Pts',(-4.93285788358386,-0.868532151155221,
64.2055675973153));
#62787=CARTESIAN_POINT('Ctrl Pts',(-4.71432797343864,-1.73832871715993,
64.2334556492873));
#62788=CARTESIAN_POINT('Ctrl Pts',(-4.28176794905193,-2.48396104258879,
64.2613437012593));
#62789=CARTESIAN_POINT('Ctrl Pts',(-3.46094380474913,-3.89886991298749,
64.3142639553413));
#62790=CARTESIAN_POINT('Ctrl Pts',(-1.86942497108703,-4.86667945271791,
64.3671842094234));
#62791=CARTESIAN_POINT('Ctrl Pts',(-0.23551477313756,-4.94450523533559,
64.4201044635053));
#62792=CARTESIAN_POINT('Ctrl Pts',(1.39839542481181,-5.02233101795326,64.4730247175873));
#62793=CARTESIAN_POINT('Ctrl Pts',(3.0746969870487,-4.21017304345841,64.5259449716692));
#62794=CARTESIAN_POINT('Ctrl Pts',(4.0262887170445,-2.87968720482404,64.5788652257512));
#62795=CARTESIAN_POINT('Ctrl Pts',(4.97788044704027,-1.5492013661897,64.6317854798331));
#62796=CARTESIAN_POINT('Ctrl Pts',(5.20476234479506,0.299612336584008,64.6847057339151));
#62797=CARTESIAN_POINT('Ctrl Pts',(4.6031097887974,1.82070851673316,64.7376259879971));
#62798=CARTESIAN_POINT('Ctrl Pts',(4.00145723279969,3.34180469688243,64.790546242079));
#62799=CARTESIAN_POINT('Ctrl Pts',(2.57127022304931,4.535183354407,64.843466496161));
#62800=CARTESIAN_POINT('Ctrl Pts',(0.967024178023638,4.85473618951069,64.896386750243));
#62801=CARTESIAN_POINT('Ctrl Pts',(-0.637221867001943,5.17428902461436,
64.9493070043249));
#62802=CARTESIAN_POINT('Ctrl Pts',(-2.41552694730285,4.62001603729727,65.0022272584069));
#62803=CARTESIAN_POINT('Ctrl Pts',(-3.55411149861537,3.44556101180013,65.0551475124888));
#62804=CARTESIAN_POINT('Ctrl Pts',(-4.43287447301319,2.53911309775405,65.0959915234403));
#62805=CARTESIAN_POINT('Ctrl Pts',(-4.93056880366583,1.26323522569467,65.1368355343917));
#62806=CARTESIAN_POINT('Ctrl Pts',(-4.94223974397651,-0.00450342756324047,
65.1776795453432));
#62807=CARTESIAN_POINT('Origin',(0.,0.,16.));
#62808=CARTESIAN_POINT('',(-4.94946148968121,0.00162189178913478,66.3223204546568));
#62809=CARTESIAN_POINT('',(-4.94905436241693,0.00206350582114702,66.1776795453432));
#62810=CARTESIAN_POINT('',(-4.942,-6.05220448138622E-16,16.));
#62811=CARTESIAN_POINT('Ctrl Pts',(-4.94946148968121,0.00162189178913478,
66.3223204546568));
#62812=CARTESIAN_POINT('Ctrl Pts',(-4.94984329083445,0.0908281755408331,
66.3194354636078));
#62813=CARTESIAN_POINT('Ctrl Pts',(-4.94764036946139,0.180015220631608,
66.3165504725587));
#62814=CARTESIAN_POINT('Ctrl Pts',(-4.9427933546869,0.26905833589981,66.3136654815097));
#62815=CARTESIAN_POINT('Ctrl Pts',(-4.8538831123176,1.90240284342791,66.2607452274277));
#62816=CARTESIAN_POINT('Ctrl Pts',(-3.87529724194047,3.48731832979629,66.2078249733457));
#62817=CARTESIAN_POINT('Ctrl Pts',(-2.45485158348742,4.2985232625058,66.1549047192638));
#62818=CARTESIAN_POINT('Ctrl Pts',(-1.03440592503428,5.10972819521536,66.1019844651818));
#62819=CARTESIAN_POINT('Ctrl Pts',(0.827899521494876,5.14722257426599,66.0490642110999));
#62820=CARTESIAN_POINT('Ctrl Pts',(2.27984534133793,4.39384839916376,65.9961439570179));
#62821=CARTESIAN_POINT('Ctrl Pts',(3.7317911611809,3.64047422406158,65.9432237029359));
#62822=CARTESIAN_POINT('Ctrl Pts',(4.77337735433786,2.09623149480659,65.8903034488539));
#62823=CARTESIAN_POINT('Ctrl Pts',(4.9279581709879,0.467789269060101,65.8373831947719));
#62824=CARTESIAN_POINT('Ctrl Pts',(5.08253898763794,-1.16065295668643,65.78446294069));
#62825=CARTESIAN_POINT('Ctrl Pts',(4.35011442778111,-2.87329467892442,65.7315426866081));
#62826=CARTESIAN_POINT('Ctrl Pts',(3.06585315610755,-3.88640488889663,65.6786224325261));
#62827=CARTESIAN_POINT('Ctrl Pts',(1.78159188443402,-4.89951509886881,65.6257021784442));
#62828=CARTESIAN_POINT('Ctrl Pts',(-0.0545060990562027,-5.21309379657515,
65.5727819243622));
#62829=CARTESIAN_POINT('Ctrl Pts',(-1.60221431494639,-4.6836425807522,65.5198616702802));
#62830=CARTESIAN_POINT('Ctrl Pts',(-3.14992253083658,-4.15419136492924,
65.4669414161983));
#62831=CARTESIAN_POINT('Ctrl Pts',(-4.40924097912677,-2.78171023557699,
65.4140211621163));
#62832=CARTESIAN_POINT('Ctrl Pts',(-4.80388630468793,-1.19426751897802,
65.3611009080343));
#62833=CARTESIAN_POINT('Ctrl Pts',(-4.90028622386234,-0.806503266718003,
65.3481740902418));
#62834=CARTESIAN_POINT('Ctrl Pts',(-4.9450930727896,-0.405912747537303,
65.3352472724493));
#62835=CARTESIAN_POINT('Ctrl Pts',(-4.94144181990917,-0.00451754960951789,
65.3223204546568));
#62836=CARTESIAN_POINT('Ctrl Pts',(-4.94223974397651,-0.00450342756324047,
65.1776795453432));
#62837=CARTESIAN_POINT('Ctrl Pts',(-4.94569046072715,-0.379332437889885,
65.1897557884737));
#62838=CARTESIAN_POINT('Ctrl Pts',(-4.90665339169033,-0.753449924055778,
65.2018320316042));
#62839=CARTESIAN_POINT('Ctrl Pts',(-4.82241576997234,-1.11709684994147,
65.2139082747347));
#62840=CARTESIAN_POINT('Ctrl Pts',(-4.45327146769261,-2.71066262250856,
65.2668285288167));
#62841=CARTESIAN_POINT('Ctrl Pts',(-3.21611884080908,-4.10315710396555,
65.3197487828986));
#62842=CARTESIAN_POINT('Ctrl Pts',(-1.67709782604308,-4.65735355244893,
65.3726690369806));
#62843=CARTESIAN_POINT('Ctrl Pts',(-0.138076811276997,-5.21155000093235,
65.4255892910626));
#62844=CARTESIAN_POINT('Ctrl Pts',(1.70281259137165,-4.92744841644198,65.4785095451446));
#62845=CARTESIAN_POINT('Ctrl Pts',(3.00315127590115,-3.9350580230386,65.5314297992265));
#62846=CARTESIAN_POINT('Ctrl Pts',(4.30348996043062,-2.94266762963524,65.5843500533085));
#62847=CARTESIAN_POINT('Ctrl Pts',(5.06327792684106,-1.24198842731896,65.6372703073904));
#62848=CARTESIAN_POINT('Ctrl Pts',(4.93482459769029,0.388722806969066,65.6901905614724));
#62849=CARTESIAN_POINT('Ctrl Pts',(4.80637126853953,2.019434041257,65.7431108155543));
#62850=CARTESIAN_POINT('Ctrl Pts',(3.78967664382766,3.58017730751661,65.7960310696363));
#62851=CARTESIAN_POINT('Ctrl Pts',(2.34999571149359,4.35673265034576,65.8489513237183));
#62852=CARTESIAN_POINT('Ctrl Pts',(0.910314779159406,5.13328799317498,65.9018715778003));
#62853=CARTESIAN_POINT('Ctrl Pts',(-0.952352460797159,5.1256554125735,65.9547918318822));
#62854=CARTESIAN_POINT('Ctrl Pts',(-2.38562103141592,4.33732769399468,66.0077120859641));
#62855=CARTESIAN_POINT('Ctrl Pts',(-3.81888960203473,3.54899997541583,66.0606323400461));
#62856=CARTESIAN_POINT('Ctrl Pts',(-4.82275950331579,1.97997711885965,66.1135525941282));
#62857=CARTESIAN_POINT('Ctrl Pts',(-4.93784453663019,0.348267946699855,
66.1664728482101));
#62858=CARTESIAN_POINT('Ctrl Pts',(-4.94596822597675,0.233087909497783,
66.1702084139211));
#62859=CARTESIAN_POINT('Ctrl Pts',(-4.94966332434242,0.117595522185004,
66.1739439796322));
#62860=CARTESIAN_POINT('Ctrl Pts',(-4.94905436241693,0.00206350582114702,
66.1776795453432));
#62861=CARTESIAN_POINT('Origin',(0.,0.,16.));
#62862=CARTESIAN_POINT('',(-4.93665814957204,0.00348993981812262,67.3223204546568));
#62863=CARTESIAN_POINT('',(-4.93610990017314,0.00319438934087567,67.1776795453432));
#62864=CARTESIAN_POINT('',(-4.942,-6.05220448138622E-16,16.));
#62865=CARTESIAN_POINT('Ctrl Pts',(-4.93665814957204,0.00348993981812262,
67.3223204546568));
#62866=CARTESIAN_POINT('Ctrl Pts',(-4.94045351450443,0.585476451976408,
67.3036236547662));
#62867=CARTESIAN_POINT('Ctrl Pts',(-4.84535018635696,1.16626258658175,67.2849268548756));
#62868=CARTESIAN_POINT('Ctrl Pts',(-4.64586699339373,1.70865983008581,67.266230054985));
#62869=CARTESIAN_POINT('Ctrl Pts',(-4.08124089061357,3.24388511502926,67.213309800903));
#62870=CARTESIAN_POINT('Ctrl Pts',(-2.68038427233572,4.47156102489275,67.1603895468211));
#62871=CARTESIAN_POINT('Ctrl Pts',(-1.08435052194541,4.82988431339829,67.1074692927391));
#62872=CARTESIAN_POINT('Ctrl Pts',(0.511683228444911,5.18820760190384,67.0545490386571));
#62873=CARTESIAN_POINT('Ctrl Pts',(2.3028941109477,4.67717826905144,67.0016287845752));
#62874=CARTESIAN_POINT('Ctrl Pts',(3.4695966691053,3.53065114235145,66.9487085304932));
#62875=CARTESIAN_POINT('Ctrl Pts',(4.6362992272629,2.38412401565146,66.8957882764113));
#62876=CARTESIAN_POINT('Ctrl Pts',(5.17849346107531,0.602099095103884,66.8428680223293));
#62877=CARTESIAN_POINT('Ctrl Pts',(4.84806300838071,-0.999941799318743,
66.7899477682473));
#62878=CARTESIAN_POINT('Ctrl Pts',(4.51763255568609,-2.60198269374146,66.7370275141654));
#62879=CARTESIAN_POINT('Ctrl Pts',(3.31457741648437,-4.02403956203921,66.6841072600834));
#62880=CARTESIAN_POINT('Ctrl Pts',(1.78943399637315,-4.61535746263258,66.6311870060014));
#62881=CARTESIAN_POINT('Ctrl Pts',(0.264290576262007,-5.20667536322592,
66.5782667519194));
#62882=CARTESIAN_POINT('Ctrl Pts',(-1.5829411247586,-4.96725429611497,66.5253464978375));
#62883=CARTESIAN_POINT('Ctrl Pts',(-2.90693966808815,-4.00665699821556,
66.4724262437555));
#62884=CARTESIAN_POINT('Ctrl Pts',(-4.15875934507,-3.09842744975845,66.4223909807226));
#62885=CARTESIAN_POINT('Ctrl Pts',(-4.94283979803511,-1.54550938030458,
66.3723557176897));
#62886=CARTESIAN_POINT('Ctrl Pts',(-4.94946148968121,0.00162189178913478,
66.3223204546568));
#62887=CARTESIAN_POINT('Ctrl Pts',(-4.94905436241693,0.00206350582114702,
66.1776795453432));
#62888=CARTESIAN_POINT('Ctrl Pts',(-4.94103640614155,-1.51909999692026,
66.2268642337141));
#62889=CARTESIAN_POINT('Ctrl Pts',(-4.18686966888732,-3.04713356331113,
66.276048922085));
#62890=CARTESIAN_POINT('Ctrl Pts',(-2.97080189349508,-3.95953726339747,
66.3252336104559));
#62891=CARTESIAN_POINT('Ctrl Pts',(-1.66237405169773,-4.94123781357185,
66.3781538645379));
#62892=CARTESIAN_POINT('Ctrl Pts',(0.180781797244686,-5.21024342615729,
66.4310741186199));
#62893=CARTESIAN_POINT('Ctrl Pts',(1.71520938689206,-4.643453024393,66.4839943727019));
#62894=CARTESIAN_POINT('Ctrl Pts',(3.24963697653938,-4.07666262262872,66.5369146267838));
#62895=CARTESIAN_POINT('Ctrl Pts',(4.47533630689159,-2.6740762065147,66.5898348808657));
#62896=CARTESIAN_POINT('Ctrl Pts',(4.83140864464272,-1.0775387413447,66.6427551349477));
#62897=CARTESIAN_POINT('Ctrl Pts',(5.18748098239386,0.518998723825342,66.6956753890297));
#62898=CARTESIAN_POINT('Ctrl Pts',(4.67392632754393,2.30948723805131,66.7485956431117));
#62899=CARTESIAN_POINT('Ctrl Pts',(3.52575513351784,3.47457191163166,66.8015158971936));
#62900=CARTESIAN_POINT('Ctrl Pts',(2.37758393949173,4.63965658521205,66.8544361512756));
#62901=CARTESIAN_POINT('Ctrl Pts',(0.59479620628932,5.17933741814667,66.9073564053575));
#62902=CARTESIAN_POINT('Ctrl Pts',(-1.0067771713956,4.84664821890178,66.9602766594395));
#62903=CARTESIAN_POINT('Ctrl Pts',(-2.60835054908043,4.5139590196569,67.0131969135215));
#62904=CARTESIAN_POINT('Ctrl Pts',(-4.02870957124789,3.3088997882326,67.0661171676034));
#62905=CARTESIAN_POINT('Ctrl Pts',(-4.61787625663849,1.78292403343541,67.1190374216854));
#62906=CARTESIAN_POINT('Ctrl Pts',(-4.83549920786993,1.2192680163841,67.138584796238));
#62907=CARTESIAN_POINT('Ctrl Pts',(-4.93971654397597,0.611827024271365,
67.1581321707906));
#62908=CARTESIAN_POINT('Ctrl Pts',(-4.93610990017314,0.00319438934087567,
67.1776795453432));
#62909=CARTESIAN_POINT('Origin',(0.,0.,16.));
#62910=CARTESIAN_POINT('',(-4.93685333923596,-0.0035819126635156,68.3223204546569));
#62911=CARTESIAN_POINT('',(-4.9374673003319,-0.00383358773467055,68.1776795453432));
#62912=CARTESIAN_POINT('',(-4.942,-6.05220448138622E-16,16.));
#62913=CARTESIAN_POINT('Ctrl Pts',(-4.93685333923596,-0.0035819126635156,
68.3223204546569));
#62914=CARTESIAN_POINT('Ctrl Pts',(-4.92964532583484,1.0704814894781,68.2878118459247));
#62915=CARTESIAN_POINT('Ctrl Pts',(-4.585217373837,2.14875374624117,68.2533032371925));
#62916=CARTESIAN_POINT('Ctrl Pts',(-3.93928885933925,2.99759934246388,68.2187946284603));
#62917=CARTESIAN_POINT('Ctrl Pts',(-2.94873310059188,4.29933610551658,68.1658743743783));
#62918=CARTESIAN_POINT('Ctrl Pts',(-1.24912700565894,5.06152146794402,68.1129541202964));
#62919=CARTESIAN_POINT('Ctrl Pts',(0.3817637188463,4.93536776727194,68.0600338662144));
#62920=CARTESIAN_POINT('Ctrl Pts',(2.01265444335154,4.80921406659986,68.0071136121325));
#62921=CARTESIAN_POINT('Ctrl Pts',(3.57482979742896,3.79472130282827,67.9541933580505));
#62922=CARTESIAN_POINT('Ctrl Pts',(4.35341448041909,2.35613685870146,67.9012731039685));
#62923=CARTESIAN_POINT('Ctrl Pts',(5.13199916340922,0.91755241457464,67.8483528498866));
#62924=CARTESIAN_POINT('Ctrl Pts',(5.12699317531198,-0.945123709907305,
67.7954325958046));
#62925=CARTESIAN_POINT('Ctrl Pts',(4.34068733273566,-2.37950247209,67.7425123417227));
#62926=CARTESIAN_POINT('Ctrl Pts',(3.55438149015938,-3.81388123427261,67.6895920876407));
#62927=CARTESIAN_POINT('Ctrl Pts',(1.98677579310383,-4.81996263415611,67.6366718335588));
#62928=CARTESIAN_POINT('Ctrl Pts',(0.355230550111662,-4.93734845757534,
67.5837515794768));
#62929=CARTESIAN_POINT('Ctrl Pts',(-1.27631469288069,-5.05473428099459,
67.5308313253949));
#62930=CARTESIAN_POINT('Ctrl Pts',(-2.9717994818098,-4.28342452794957,67.4779110713129));
#62931=CARTESIAN_POINT('Ctrl Pts',(-3.95534408263313,-2.97638232141527,
67.4249908172309));
#62932=CARTESIAN_POINT('Ctrl Pts',(-4.59140099837083,-2.13111995717548,
67.3907673630395));
#62933=CARTESIAN_POINT('Ctrl Pts',(-4.92971094477425,-1.06180405997696,
67.3565439088482));
#62934=CARTESIAN_POINT('Ctrl Pts',(-4.93665814957204,0.00348993981812262,
67.3223204546568));
#62935=CARTESIAN_POINT('Ctrl Pts',(-4.93610990017314,0.00319438934087567,
67.1776795453432));
#62936=CARTESIAN_POINT('Ctrl Pts',(-4.929952342348,-1.03591311578948,67.2110524248726));
#62937=CARTESIAN_POINT('Ctrl Pts',(-4.60950819503561,-2.07849403525122,
67.2444253044019));
#62938=CARTESIAN_POINT('Ctrl Pts',(-4.00255393693903,-2.91258668755472,
67.2777981839313));
#62939=CARTESIAN_POINT('Ctrl Pts',(-3.0400905832352,-4.23522937557753,67.3307184380133));
#62940=CARTESIAN_POINT('Ctrl Pts',(-1.35718952721374,-5.03362247345304,
67.3836386920952));
#62941=CARTESIAN_POINT('Ctrl Pts',(0.276028005448868,-4.94240910597606,
67.4365589461772));
#62942=CARTESIAN_POINT('Ctrl Pts',(1.90924553811157,-4.85119573849907,67.4894792002592));
#62943=CARTESIAN_POINT('Ctrl Pts',(3.49277954741543,-3.87037590566948,67.5423994543411));
#62944=CARTESIAN_POINT('Ctrl Pts',(4.30198068586489,-2.4487877427561,67.5953197084231));
#62945=CARTESIAN_POINT('Ctrl Pts',(5.11118182431431,-1.0271995798428,67.6482399625051));
#62946=CARTESIAN_POINT('Ctrl Pts',(5.14605009190941,0.835156913154248,67.7011602165871));
#62947=CARTESIAN_POINT('Ctrl Pts',(4.39062923686613,2.28603896182972,67.754080470669));
#62948=CARTESIAN_POINT('Ctrl Pts',(3.63520838182284,3.73692101050519,67.8070007247509));
#62949=CARTESIAN_POINT('Ctrl Pts',(2.08949840414118,4.77632861485907,67.8599209788329));
#62950=CARTESIAN_POINT('Ctrl Pts',(0.460839796771268,4.92861298057972,67.9128412329148));
#62951=CARTESIAN_POINT('Ctrl Pts',(-1.16781881059865,5.08089734630037,67.9657614869968));
#62952=CARTESIAN_POINT('Ctrl Pts',(-2.87942604765681,4.34605847338777,68.0186817410788));
#62953=CARTESIAN_POINT('Ctrl Pts',(-3.89072430186352,3.06036985305955,68.0716019951608));
#62954=CARTESIAN_POINT('Ctrl Pts',(-4.56643308401115,2.20132447426127,68.1069611785549));
#62955=CARTESIAN_POINT('Ctrl Pts',(-4.92949771464715,1.09635914283018,68.142320361949));
#62956=CARTESIAN_POINT('Ctrl Pts',(-4.9374673003319,-0.00383358773467055,
68.1776795453432));
#62957=CARTESIAN_POINT('Origin',(0.,0.,16.));
#62958=CARTESIAN_POINT('',(-4.94957828458471,-0.00146882823891858,69.3223204546568));
#62959=CARTESIAN_POINT('',(-4.94986277816997,-0.00100007488610477,69.1776795453432));
#62960=CARTESIAN_POINT('',(-4.942,-6.05220448138622E-16,16.));
#62961=CARTESIAN_POINT('Ctrl Pts',(-4.94957828458471,-0.00146882823891858,
69.3223204546568));
#62962=CARTESIAN_POINT('Ctrl Pts',(-4.94347825971363,1.5543817607618,69.2720000370831));
#62963=CARTESIAN_POINT('Ctrl Pts',(-4.14920711766337,3.115598423098,69.2216796195094));
#62964=CARTESIAN_POINT('Ctrl Pts',(-2.8853618522021,4.0222239516356,69.1713592019357));
#62965=CARTESIAN_POINT('Ctrl Pts',(-1.55621921401708,4.97569086707049,69.1184389478537));
#62966=CARTESIAN_POINT('Ctrl Pts',(0.292272693635941,5.20517958568956,69.0655186937718));
#62967=CARTESIAN_POINT('Ctrl Pts',(1.81421574235462,4.60567256494064,69.0125984396898));
#62968=CARTESIAN_POINT('Ctrl Pts',(3.3361587910733,4.00616554419172,68.9596781856078));
#62969=CARTESIAN_POINT('Ctrl Pts',(4.53155298085772,2.57766278407475,68.9067579315258));
#62970=CARTESIAN_POINT('Ctrl Pts',(4.85336767356702,0.973868964711821,68.8538376774439));
#62971=CARTESIAN_POINT('Ctrl Pts',(5.17518236627633,-0.629924854651203,
68.8009174233619));
#62972=CARTESIAN_POINT('Ctrl Pts',(4.62341756191056,-2.40900973326008,68.74799716928));
#62973=CARTESIAN_POINT('Ctrl Pts',(3.45056926188509,-3.5492492592361,68.695076915198));
#62974=CARTESIAN_POINT('Ctrl Pts',(2.27772096185968,-4.68948878521204,68.6421566611161));
#62975=CARTESIAN_POINT('Ctrl Pts',(0.483789166174606,-5.19088295855499,
68.5892364070341));
#62976=CARTESIAN_POINT('Ctrl Pts',(-1.11029553728448,-4.82398614790096,
68.5363161529521));
#62977=CARTESIAN_POINT('Ctrl Pts',(-2.70438024074366,-4.45708933724691,
68.4833958988701));
#62978=CARTESIAN_POINT('Ctrl Pts',(-4.09861785197692,-3.22190154259576,
68.4304756447882));
#62979=CARTESIAN_POINT('Ctrl Pts',(-4.65498394631264,-1.6836635634312,68.3775553907063));
#62980=CARTESIAN_POINT('Ctrl Pts',(-4.84855095371391,-1.14849054456963,
68.3591437453565));
#62981=CARTESIAN_POINT('Ctrl Pts',(-4.94069908646524,-0.576635280213381,
68.3407321000067));
#62982=CARTESIAN_POINT('Ctrl Pts',(-4.93685333923596,-0.0035819126635156,
68.3223204546569));
#62983=CARTESIAN_POINT('Ctrl Pts',(-4.9374673003319,-0.00383358773467055,
68.1776795453432));
#62984=CARTESIAN_POINT('Ctrl Pts',(-4.94142537979325,-0.550242199503817,
68.195240616031));
#62985=CARTESIAN_POINT('Ctrl Pts',(-4.85779595713247,-1.09547360479138,
68.2128016867188));
#62986=CARTESIAN_POINT('Ctrl Pts',(-4.68137867571166,-1.60881724419501,
68.2303627574066));
#62987=CARTESIAN_POINT('Ctrl Pts',(-4.14974552399779,-3.15577735337756,
68.2832830114886));
#62988=CARTESIAN_POINT('Ctrl Pts',(-2.77548994921469,-4.41315920399872,
68.3362032655706));
#62989=CARTESIAN_POINT('Ctrl Pts',(-1.18749229097476,-4.8055656575998,68.3891235196525));
#62990=CARTESIAN_POINT('Ctrl Pts',(0.400505367265077,-5.19797211120086,
68.4420437737345));
#62991=CARTESIAN_POINT('Ctrl Pts',(2.20224510896182,-4.72540316778197,68.4949640278164));
#62992=CARTESIAN_POINT('Ctrl Pts',(3.39322331088645,-3.60411359325479,68.5478842818984));
#62993=CARTESIAN_POINT('Ctrl Pts',(4.58420151281108,-2.48282401872761,68.6008045359804));
#62994=CARTESIAN_POINT('Ctrl Pts',(5.16441817496363,-0.71281381309235,68.6537247900624));
#62995=CARTESIAN_POINT('Ctrl Pts',(4.8683572912689,0.895933320719813,68.7066450441443));
#62996=CARTESIAN_POINT('Ctrl Pts',(4.57229640757415,2.50468045453207,68.7595652982263));
#62997=CARTESIAN_POINT('Ctrl Pts',(3.39995797803181,3.95216451652107,68.8124855523082));
#62998=CARTESIAN_POINT('Ctrl Pts',(1.88782197277238,4.57599469293234,68.8654058063902));
#62999=CARTESIAN_POINT('Ctrl Pts',(0.375685967513026,5.19982486934357,68.9183260604721));
#63000=CARTESIAN_POINT('Ctrl Pts',(-1.47624761346349,5.00000116017722,68.9712463145541));
#63001=CARTESIAN_POINT('Ctrl Pts',(-2.82050567947833,4.06796594659513,69.0241665686361));
#63002=CARTESIAN_POINT('Ctrl Pts',(-4.1203297308193,3.16673885490861,69.0753375608718));
#63003=CARTESIAN_POINT('Ctrl Pts',(-4.94548567424374,1.58090626393571,69.1265085531075));
#63004=CARTESIAN_POINT('Ctrl Pts',(-4.94986277816997,-0.00100007488610477,
69.1776795453432));
#63005=CARTESIAN_POINT('Origin',(0.,0.,16.));
#63006=CARTESIAN_POINT('',(-4.94117660785543,0.00451214175946527,70.3223204546568));
#63007=CARTESIAN_POINT('',(-4.94039592783718,0.00446617472429873,70.1776795453432));
#63008=CARTESIAN_POINT('',(-4.942,-6.05220448138622E-16,16.));
#63009=CARTESIAN_POINT('Ctrl Pts',(-4.94117660785543,0.00451214175946527,
70.3223204546568));
#63010=CARTESIAN_POINT('Ctrl Pts',(-4.94488654917412,0.414817947726635,
70.3091084823236));
#63011=CARTESIAN_POINT('Ctrl Pts',(-4.8980529188199,0.824288512579107,70.2958965099902));
#63012=CARTESIAN_POINT('Ctrl Pts',(-4.79739770972192,1.22007120694207,70.2826845376569));
#63013=CARTESIAN_POINT('Ctrl Pts',(-4.39422556359881,2.80536976937794,70.229764283575));
#63014=CARTESIAN_POINT('Ctrl Pts',(-3.12754820616573,4.17106222260404,70.176844029493));
#63015=CARTESIAN_POINT('Ctrl Pts',(-1.57701654176587,4.69218684221452,70.123923775411));
#63016=CARTESIAN_POINT('Ctrl Pts',(-0.0264848773660925,5.21331146182497,
70.071003521329));
#63017=CARTESIAN_POINT('Ctrl Pts',(1.80790109400033,4.88986824781988,70.0180832672471));
#63018=CARTESIAN_POINT('Ctrl Pts',(3.0866983358117,3.86986975477877,69.9651630131651));
#63019=CARTESIAN_POINT('Ctrl Pts',(4.36549557762306,2.84987126173766,69.9122427590831));
#63020=CARTESIAN_POINT('Ctrl Pts',(5.08870408987935,1.13331748966031,69.8593225050012));
#63021=CARTESIAN_POINT('Ctrl Pts',(4.9253726120261,-0.494270338941504,69.8064022509192));
#63022=CARTESIAN_POINT('Ctrl Pts',(4.76204113417285,-2.12185816754332,69.7534819968373));
#63023=CARTESIAN_POINT('Ctrl Pts',(3.71216966621028,-3.66048005266973,69.7005617427553));
#63024=CARTESIAN_POINT('Ctrl Pts',(2.25619542624873,-4.40603912077827,69.6476414886733));
#63025=CARTESIAN_POINT('Ctrl Pts',(0.80022118628726,-5.15159818888676,69.5947212345913));
#63026=CARTESIAN_POINT('Ctrl Pts',(-1.06185582567303,-5.10409443997744,
69.5418009805094));
#63027=CARTESIAN_POINT('Ctrl Pts',(-2.47792073001783,-4.28526631506165,
69.4888807264275));
#63028=CARTESIAN_POINT('Ctrl Pts',(-3.89398563436272,-3.46643819014582,
69.4359604723455));
#63029=CARTESIAN_POINT('Ctrl Pts',(-4.864038431092,-1.87628568922347,69.3830402182635));
#63030=CARTESIAN_POINT('Ctrl Pts',(-4.94416814509815,-0.242486882636884,
69.3301199641816));
#63031=CARTESIAN_POINT('Ctrl Pts',(-4.94810471266539,-0.162222532848887,
69.3275201276733));
#63032=CARTESIAN_POINT('Ctrl Pts',(-4.94989344626512,-0.081852842476203,
69.3249202911651));
#63033=CARTESIAN_POINT('Ctrl Pts',(-4.94957828458471,-0.00146882823891858,
69.3223204546568));
#63034=CARTESIAN_POINT('Ctrl Pts',(-4.94986277816997,-0.00100007488610477,
69.1776795453432));
#63035=CARTESIAN_POINT('Ctrl Pts',(-4.95001240788323,-0.0550769704471047,
69.1794288071895));
#63036=CARTESIAN_POINT('Ctrl Pts',(-4.94920288408253,-0.10914927783116,
69.1811780690357));
#63037=CARTESIAN_POINT('Ctrl Pts',(-4.94742038040276,-0.163189491703912,
69.182927330882));
#63038=CARTESIAN_POINT('Ctrl Pts',(-4.89349446425897,-1.79806299842275,
69.2358475849639));
#63039=CARTESIAN_POINT('Ctrl Pts',(-3.94906008091826,-3.40356329386249,
69.2887678390458));
#63040=CARTESIAN_POINT('Ctrl Pts',(-2.54630482825922,-4.24498892250744,
69.3416880931278));
#63041=CARTESIAN_POINT('Ctrl Pts',(-1.14354957560017,-5.0864145511524,69.3946083472098));
#63042=CARTESIAN_POINT('Ctrl Pts',(0.717526546377131,-5.16376551300254,
69.4475286012918));
#63043=CARTESIAN_POINT('Ctrl Pts',(2.18526668060081,-4.44164482655728,69.5004488553738));
#63044=CARTESIAN_POINT('Ctrl Pts',(3.65300681482441,-3.71952414011206,69.5533691094558));
#63045=CARTESIAN_POINT('Ctrl Pts',(4.72741096129446,-2.19793180537131,69.6062893635377));
#63046=CARTESIAN_POINT('Ctrl Pts',(4.91681537353513,-0.573171713534203,
69.6592096176196));
#63047=CARTESIAN_POINT('Ctrl Pts',(5.1062197857758,1.05158837830299,69.7121298717016));
#63048=CARTESIAN_POINT('Ctrl Pts',(4.41062446378718,2.77951622723674,69.7650501257836));
#63049=CARTESIAN_POINT('Ctrl Pts',(3.14834445052908,3.81988565947332,69.8179703798655));
#63050=CARTESIAN_POINT('Ctrl Pts',(1.88606443727098,4.8602550917099,69.8708906339475));
#63051=CARTESIAN_POINT('Ctrl Pts',(0.0570997327434936,5.21306610724925,
69.9238108880295));
#63052=CARTESIAN_POINT('Ctrl Pts',(-1.50158748103454,4.71686699700421,69.9767311421114));
#63053=CARTESIAN_POINT('Ctrl Pts',(-3.06027469481266,4.22066788675913,70.0296513961934));
#63054=CARTESIAN_POINT('Ctrl Pts',(-4.34868441784121,2.87545865072958,70.0825716502754));
#63055=CARTESIAN_POINT('Ctrl Pts',(-4.77722068336862,1.29682758029823,70.1354919043573));
#63056=CARTESIAN_POINT('Ctrl Pts',(-4.8910960129131,0.877336517731382,70.1495544513526));
#63057=CARTESIAN_POINT('Ctrl Pts',(-4.9442531721895,0.441362859310636,70.1636169983479));
#63058=CARTESIAN_POINT('Ctrl Pts',(-4.94039592783718,0.00446617472429873,
70.1776795453432));
#63059=CARTESIAN_POINT('Origin',(0.,0.,16.));
#63060=CARTESIAN_POINT('',(-4.93421645959303,-0.00129368103133631,71.3223204546568));
#63061=CARTESIAN_POINT('',(-4.93445704478049,-0.00170468936910681,71.1776795453431));
#63062=CARTESIAN_POINT('',(-4.942,-6.05220448138622E-16,16.));
#63063=CARTESIAN_POINT('Ctrl Pts',(-4.93421645959303,-0.00129368103133631,
71.3223204546568));
#63064=CARTESIAN_POINT('Ctrl Pts',(-4.93209641645617,0.903267203006942,
71.293296673482));
#63065=CARTESIAN_POINT('Ctrl Pts',(-4.69429817649842,1.80886543486343,71.2642728923071));
#63066=CARTESIAN_POINT('Ctrl Pts',(-4.22761420074216,2.5750488742813,71.2352491111322));
#63067=CARTESIAN_POINT('Ctrl Pts',(-3.37669011114097,3.97206265560444,71.1823288570503));
#63068=CARTESIAN_POINT('Ctrl Pts',(-1.76481870913523,4.90558179736215,71.1294086029683));
#63069=CARTESIAN_POINT('Ctrl Pts',(-0.129616965909283,4.94841368292938,
71.0764883488863));
#63070=CARTESIAN_POINT('Ctrl Pts',(1.50558477731675,4.9912455684966,71.0235680948044));
#63071=CARTESIAN_POINT('Ctrl Pts',(3.164116861763,4.14339019787323,70.9706478407224));
#63072=CARTESIAN_POINT('Ctrl Pts',(4.08700967532571,2.79283913769631,70.9177275866405));
#63073=CARTESIAN_POINT('Ctrl Pts',(5.00990248888837,1.44228807751946,70.8648073325585));
#63074=CARTESIAN_POINT('Ctrl Pts',(5.19715603156758,-0.410958672210887,
70.8118870784765));
#63075=CARTESIAN_POINT('Ctrl Pts',(4.56308022236637,-1.91882709473861,70.7589668243946));
#63076=CARTESIAN_POINT('Ctrl Pts',(3.92900441316517,-3.42669551726634,70.7060465703126));
#63077=CARTESIAN_POINT('Ctrl Pts',(2.47359925208355,-4.58918561259145,70.6531263162307));
#63078=CARTESIAN_POINT('Ctrl Pts',(0.86288036879719,-4.87432415873202,70.6002060621487));
#63079=CARTESIAN_POINT('Ctrl Pts',(-0.747838514489167,-5.1594627048726,
70.5472858080667));
#63080=CARTESIAN_POINT('Ctrl Pts',(-2.51387111998026,-4.56724970182864,
70.4943655539847));
#63081=CARTESIAN_POINT('Ctrl Pts',(-3.62705395531922,-3.36869086448392,
70.4414452999028));
#63082=CARTESIAN_POINT('Ctrl Pts',(-4.46232163175454,-2.46936200011537,
70.4017370181541));
#63083=CARTESIAN_POINT('Ctrl Pts',(-4.93002646377116,-1.22865260726002,
70.3620287364055));
#63084=CARTESIAN_POINT('Ctrl Pts',(-4.94117660785543,0.00451214175946527,
70.3223204546568));
#63085=CARTESIAN_POINT('Ctrl Pts',(-4.94039592783718,0.00446617472429873,
70.1776795453432));
#63086=CARTESIAN_POINT('Ctrl Pts',(-4.92973756905946,-1.20276914349332,
70.2165372524299));
#63087=CARTESIAN_POINT('Ctrl Pts',(-4.48375687255021,-2.4170520476298,70.2553949595166));
#63088=CARTESIAN_POINT('Ctrl Pts',(-3.68059559417778,-3.31010805001079,
70.2942526666032));
#63089=CARTESIAN_POINT('Ctrl Pts',(-2.58677143143322,-4.52635970505561,
70.3471729206852));
#63090=CARTESIAN_POINT('Ctrl Pts',(-0.83046029791784,-5.14681011031225,
70.4000931747671));
#63091=CARTESIAN_POINT('Ctrl Pts',(0.784623008060776,-4.88753168438311,
70.453013428849));
#63092=CARTESIAN_POINT('Ctrl Pts',(2.3997063140393,-4.62825325845398,70.505933682931));
#63093=CARTESIAN_POINT('Ctrl Pts',(3.87356179248119,-3.48924600133894,70.558853937013));
#63094=CARTESIAN_POINT('Ctrl Pts',(4.53173066670028,-1.99173702960891,70.611774191095));
#63095=CARTESIAN_POINT('Ctrl Pts',(5.18989954091941,-0.494228057878804,
70.664694445177));
#63096=CARTESIAN_POINT('Ctrl Pts',(5.0323818109159,1.36178262846646,70.7176146992589));
#63097=CARTESIAN_POINT('Ctrl Pts',(4.13125999566019,2.72695619306305,70.7705349533408));
#63098=CARTESIAN_POINT('Ctrl Pts',(3.23013818040442,4.09212975765972,70.8234552074228));
#63099=CARTESIAN_POINT('Ctrl Pts',(1.58541227989642,4.96646620050757,70.8763754615048));
#63100=CARTESIAN_POINT('Ctrl Pts',(-0.0502660143879759,4.94985581188227,
70.9292957155868));
#63101=CARTESIAN_POINT('Ctrl Pts',(-1.68594430867228,4.93324542325696,70.9822159696687));
#63102=CARTESIAN_POINT('Ctrl Pts',(-3.3125749967329,4.02568820315859,71.0351362237507));
#63103=CARTESIAN_POINT('Ctrl Pts',(-4.18578703267271,2.64249619635225,71.0880564778327));
#63104=CARTESIAN_POINT('Ctrl Pts',(-4.67872962214464,1.86166150614078,71.1179308336695));
#63105=CARTESIAN_POINT('Ctrl Pts',(-4.93157361279594,0.929252063276933,
71.1478051895063));
#63106=CARTESIAN_POINT('Ctrl Pts',(-4.93445704478049,-0.00170468936910681,
71.1776795453431));
#63107=CARTESIAN_POINT('Origin',(0.,0.,16.));
#63108=CARTESIAN_POINT('',(-4.9459185577707,-0.00382965742011687,72.3223204546568));
#63109=CARTESIAN_POINT('',(-4.9466376895248,-0.00356105100536129,72.1776795453432));
#63110=CARTESIAN_POINT('',(-4.942,-6.05220448138622E-16,16.));
#63111=CARTESIAN_POINT('Ctrl Pts',(-4.9459185577707,-0.00382965742011687,
72.3223204546568));
#63112=CARTESIAN_POINT('Ctrl Pts',(-4.93404671791329,1.38513423103216,72.2774848646404));
#63113=CARTESIAN_POINT('Ctrl Pts',(-4.32176677967432,2.78326338156107,72.232649274624));
#63114=CARTESIAN_POINT('Ctrl Pts',(-3.28505857961465,3.70297024883463,72.1878136846076));
#63115=CARTESIAN_POINT('Ctrl Pts',(-2.06141322698447,4.78851682197505,72.1348934305256));
#63116=CARTESIAN_POINT('Ctrl Pts',(-0.246475391513582,5.20754910952386,
72.0819731764437));
#63117=CARTESIAN_POINT('Ctrl Pts',(1.32921165428745,4.76831153694478,72.0290529223617));
#63118=CARTESIAN_POINT('Ctrl Pts',(2.90489870008848,4.32907396436569,71.9761326682797));
#63119=CARTESIAN_POINT('Ctrl Pts',(4.24133495621976,3.03156653165866,71.9232124141978));
#63120=CARTESIAN_POINT('Ctrl Pts',(4.72694678088706,1.46954845647079,71.8702921601158));
#63121=CARTESIAN_POINT('Ctrl Pts',(5.21255860555439,-0.09246961871717,71.8173719060338));
#63122=CARTESIAN_POINT('Ctrl Pts',(4.84734599875778,-1.91899833638585,71.7644516519519));
#63123=CARTESIAN_POINT('Ctrl Pts',(3.79843582714949,-3.17419025930731,71.7115313978699));
#63124=CARTESIAN_POINT('Ctrl Pts',(2.74952565554119,-4.42938218222877,71.658611143788));
#63125=CARTESIAN_POINT('Ctrl Pts',(1.0169179191211,-5.1132373104028,71.605690889706));
#63126=CARTESIAN_POINT('Ctrl Pts',(-0.60651962032857,-4.91281309286346,
71.552770635624));
#63127=CARTESIAN_POINT('Ctrl Pts',(-2.22995715977815,-4.71238887532414,
71.4998503815421));
#63128=CARTESIAN_POINT('Ctrl Pts',(-3.74422450225742,-3.62768531207155,
71.4469301274601));
#63129=CARTESIAN_POINT('Ctrl Pts',(-4.45636978489872,-2.15507932000099,
71.3940098733781));
#63130=CARTESIAN_POINT('Ctrl Pts',(-4.77794345735694,-1.49011484084619,
71.370113400471));
#63131=CARTESIAN_POINT('Ctrl Pts',(-4.93596197831358,-0.746055865118146,
71.3462169275639));
#63132=CARTESIAN_POINT('Ctrl Pts',(-4.93421645959303,-0.00129368103133631,
71.3223204546568));
#63133=CARTESIAN_POINT('Ctrl Pts',(-4.93445704478049,-0.00170468936910681,
71.1776795453431));
#63134=CARTESIAN_POINT('Ctrl Pts',(-4.93668140337337,-0.71987028628676,
71.2007254435883));
#63135=CARTESIAN_POINT('Ctrl Pts',(-4.79015415455198,-1.43717138679696,
71.2237713418334));
#63136=CARTESIAN_POINT('Ctrl Pts',(-4.49034790212576,-2.08335665417659,
71.2468172400785));
#63137=CARTESIAN_POINT('Ctrl Pts',(-3.80190335182005,-3.56719070438483,
71.2997374941605));
#63138=CARTESIAN_POINT('Ctrl Pts',(-2.30522086738965,-4.67603201128707,
71.3526577482425));
#63139=CARTESIAN_POINT('Ctrl Pts',(-0.685205212090817,-4.90245785784546,
71.4055780023244));
#63140=CARTESIAN_POINT('Ctrl Pts',(0.934810443208014,-5.12888370440385,
71.4584982564064));
#63141=CARTESIAN_POINT('Ctrl Pts',(2.67815926937537,-4.47289409061839,71.5114185104883));
#63142=CARTESIAN_POINT('Ctrl Pts',(3.74705821791536,-3.23467988248916,71.5643387645703));
#63143=CARTESIAN_POINT('Ctrl Pts',(4.8159571664554,-1.99646567435987,71.6172590186523));
#63144=CARTESIAN_POINT('Ctrl Pts',(5.21040623736806,-0.176026871886955,
71.6701792727342));
#63145=CARTESIAN_POINT('Ctrl Pts',(4.74989951150191,1.39357592590467,71.7230995268162));
#63146=CARTESIAN_POINT('Ctrl Pts',(4.28939278563578,2.96317872369621,71.7760197808982));
#63147=CARTESIAN_POINT('Ctrl Pts',(2.97393026299076,4.28194551680631,71.8289400349801));
#63148=CARTESIAN_POINT('Ctrl Pts',(1.40548768459228,4.74638847957966,71.8818602890621));
#63149=CARTESIAN_POINT('Ctrl Pts',(-0.162954893806299,5.21083144235304,
71.934780543144));
#63150=CARTESIAN_POINT('Ctrl Pts',(-1.98437752795848,4.82095057478956,71.987700797226));
#63151=CARTESIAN_POINT('Ctrl Pts',(-3.22526940243671,3.7551613164194,72.040621051308));
#63152=CARTESIAN_POINT('Ctrl Pts',(-4.29653392126676,2.83506324782479,72.0863072159864));
#63153=CARTESIAN_POINT('Ctrl Pts',(-4.93513440489649,1.41121710573191,72.1319933806648));
#63154=CARTESIAN_POINT('Ctrl Pts',(-4.9466376895248,-0.00356105100536129,
72.1776795453432));
#63155=CARTESIAN_POINT('Origin',(0.,0.,16.));
#63156=CARTESIAN_POINT('',(-4.94622533435752,0.00372181280100414,73.3223204546568));
#63157=CARTESIAN_POINT('',(-4.94548609638219,0.00396606047658106,73.1776795453432));
#63158=CARTESIAN_POINT('',(-4.942,-6.05220448138622E-16,16.));
#63159=CARTESIAN_POINT('Ctrl Pts',(-4.94622533435752,0.00372181280100414,
73.3223204546568));
#63160=CARTESIAN_POINT('Ctrl Pts',(-4.94823216917571,0.243062776937041,
73.3145933098808));
#63161=CARTESIAN_POINT('Ctrl Pts',(-4.93236152324834,0.482136497176127,
73.3068661651048));
#63162=CARTESIAN_POINT('Ctrl Pts',(-4.89769574881769,0.718453121134063,
73.2991390203288));
#63163=CARTESIAN_POINT('Ctrl Pts',(-4.66028314118601,2.33689513900433,73.2462187662469));
#63164=CARTESIAN_POINT('Ctrl Pts',(-3.5413122266531,3.82601954517773,73.1932985121649));
#63165=CARTESIAN_POINT('Ctrl Pts',(-2.05284118541496,4.50438026844074,73.1403782580829));
#63166=CARTESIAN_POINT('Ctrl Pts',(-0.564370144176819,5.18274099170376,
73.087458004001));
#63167=CARTESIAN_POINT('Ctrl Pts',(1.29360102376645,5.05033803205637,73.034537749919));
#63168=CARTESIAN_POINT('Ctrl Pts',(2.67083633572998,4.16776100598374,72.9816174958371));
#63169=CARTESIAN_POINT('Ctrl Pts',(4.04807164769343,3.28518397991116,72.9286972417551));
#63170=CARTESIAN_POINT('Ctrl Pts',(4.9445711036771,1.6524328874135,72.8757769876731));
#63171=CARTESIAN_POINT('Ctrl Pts',(4.95008286065676,0.0166795649332413,
72.8228567335911));
#63172=CARTESIAN_POINT('Ctrl Pts',(4.95559461763642,-1.61907375754711,72.7699364795092));
#63173=CARTESIAN_POINT('Ctrl Pts',(4.07011867561174,-3.25782931001015,72.7170162254272));
#63174=CARTESIAN_POINT('Ctrl Pts',(2.69886234926083,-4.14966752342842,72.6640959713453));
#63175=CARTESIAN_POINT('Ctrl Pts',(1.32760602290984,-5.04150573684673,72.6111757172633));
#63176=CARTESIAN_POINT('Ctrl Pts',(-0.529430687767451,-5.18642661122039,
72.5582554631813));
#63177=CARTESIAN_POINT('Ctrl Pts',(-2.02243942200268,-4.51811214110315,
72.5053352090994));
#63178=CARTESIAN_POINT('Ctrl Pts',(-3.51544815623782,-3.84979767098594,
72.4524149550174));
#63179=CARTESIAN_POINT('Ctrl Pts',(-4.64442891403086,-2.36824785637795,
72.3994947009354));
#63180=CARTESIAN_POINT('Ctrl Pts',(-4.89274285803262,-0.751442519707904,
72.3465744468535));
#63181=CARTESIAN_POINT('Ctrl Pts',(-4.93067795216383,-0.50444204261031,
72.3384897827879));
#63182=CARTESIAN_POINT('Ctrl Pts',(-4.9480592642285,-0.254284852349217,
72.3304051187224));
#63183=CARTESIAN_POINT('Ctrl Pts',(-4.9459185577707,-0.00382965742011687,
72.3223204546568));
#63184=CARTESIAN_POINT('Ctrl Pts',(-4.9466376895248,-0.00356105100536129,
72.1776795453432));
#63185=CARTESIAN_POINT('Ctrl Pts',(-4.94845915538918,-0.227581424440414,
72.1849136347467));
#63186=CARTESIAN_POINT('Ctrl Pts',(-4.93455770132463,-0.451374440445247,
72.1921477241503));
#63187=CARTESIAN_POINT('Ctrl Pts',(-4.90416141521875,-0.672904186423828,
72.1993818135539));
#63188=CARTESIAN_POINT('Ctrl Pts',(-4.68180043871832,-2.29348278172022,
72.2523020676359));
#63189=CARTESIAN_POINT('Ctrl Pts',(-3.57671737091314,-3.79294232313627,
72.3052223217178));
#63190=CARTESIAN_POINT('Ctrl Pts',(-2.09461510123176,-4.48510722372598,
72.3581425757998));
#63191=CARTESIAN_POINT('Ctrl Pts',(-0.612512831550301,-5.17727212431573,
72.4110628298817));
#63192=CARTESIAN_POINT('Ctrl Pts',(1.24660864000739,-5.06214238407903,72.4639830839637));
#63193=CARTESIAN_POINT('Ctrl Pts',(2.63198693425408,-4.19240313049007,72.5169033380457));
#63194=CARTESIAN_POINT('Ctrl Pts',(4.01736522850069,-3.32266387690115,72.5698235921276));
#63195=CARTESIAN_POINT('Ctrl Pts',(4.92900034543634,-1.69831510996005,72.6227438462096));
#63196=CARTESIAN_POINT('Ctrl Pts',(4.94971413242267,-0.0626836336085702,
72.6756641002916));
#63197=CARTESIAN_POINT('Ctrl Pts',(4.97042791940901,1.57294784274291,72.7285843543735));
#63198=CARTESIAN_POINT('Ctrl Pts',(4.10022037644603,3.21986202850478,72.7815046084555));
#63199=CARTESIAN_POINT('Ctrl Pts',(2.73731176561134,4.12440583944801,72.8344248625374));
#63200=CARTESIAN_POINT('Ctrl Pts',(1.37440315477665,5.02894965039124,72.8873451166194));
#63201=CARTESIAN_POINT('Ctrl Pts',(-0.481206523929751,5.19112308651582,
72.9402653707013));
#63202=CARTESIAN_POINT('Ctrl Pts',(-1.98036194136401,4.53671310662511,72.9931856247833));
#63203=CARTESIAN_POINT('Ctrl Pts',(-3.47951735879827,3.8823031267344,73.0461058788653));
#63204=CARTESIAN_POINT('Ctrl Pts',(-4.62221851496038,2.41130973082838,73.0990261329473));
#63205=CARTESIAN_POINT('Ctrl Pts',(-4.88554790865992,0.796881962912803,
73.1519463870292));
#63206=CARTESIAN_POINT('Ctrl Pts',(-4.92823035034716,0.535203165516849,
73.1605241064672));
#63207=CARTESIAN_POINT('Ctrl Pts',(-4.94780958080646,0.269756002185876,
73.1691018259052));
#63208=CARTESIAN_POINT('Ctrl Pts',(-4.94548609638219,0.00396606047658106,
73.1776795453432));
#63209=CARTESIAN_POINT('Origin',(0.,0.,16.));
#63210=CARTESIAN_POINT('',(-4.93430944804537,0.00146807591443893,74.3223204546568));
#63211=CARTESIAN_POINT('',(-4.93410780896188,0.00104985362950368,74.1776795453432));
#63212=CARTESIAN_POINT('',(-4.942,-6.05220448138622E-16,16.));
#63213=CARTESIAN_POINT('Ctrl Pts',(-4.93430944804537,0.00146807591443893,
74.3223204546568));
#63214=CARTESIAN_POINT('Ctrl Pts',(-4.93626271862051,0.735053226945857,
74.2987815010393));
#63215=CARTESIAN_POINT('Ctrl Pts',(-4.78313292282981,1.46786315098495,74.2752425474217));
#63216=CARTESIAN_POINT('Ctrl Pts',(-4.47079173349639,2.12499877904777,74.2517035938041));
#63217=CARTESIAN_POINT('Ctrl Pts',(-3.76858655614047,3.60237049949084,74.1987833397222));
#63218=CARTESIAN_POINT('Ctrl Pts',(-2.2616634474919,4.69725412310252,74.1458630856402));
#63219=CARTESIAN_POINT('Ctrl Pts',(-0.639613436851163,4.9086141818902,74.0929428315583));
#63220=CARTESIAN_POINT('Ctrl Pts',(0.982436573789575,5.11997424067789,74.0400225774763));
#63221=CARTESIAN_POINT('Ctrl Pts',(2.71961348642258,4.44781073464159,73.9871023233943));
#63222=CARTESIAN_POINT('Ctrl Pts',(3.77695861444706,3.19971594989436,73.9341820693124));
#63223=CARTESIAN_POINT('Ctrl Pts',(4.83430374247159,1.95162116514706,73.8812618152304));
#63224=CARTESIAN_POINT('Ctrl Pts',(5.21181708588759,0.127595101688968,73.8283415611484));
#63225=CARTESIAN_POINT('Ctrl Pts',(4.73674277310034,-1.43766005604103,73.7754213070665));
#63226=CARTESIAN_POINT('Ctrl Pts',(4.26166846031312,-3.00291521377094,73.7225010529845));
#63227=CARTESIAN_POINT('Ctrl Pts',(2.9340064913226,-4.30939946577263,73.6695807989026));
#63228=CARTESIAN_POINT('Ctrl Pts',(1.36131526012037,-4.7592456647895,73.6166605448206));
#63229=CARTESIAN_POINT('Ctrl Pts',(-0.211375971081961,-5.2090918638064,
73.5637402907386));
#63230=CARTESIAN_POINT('Ctrl Pts',(-2.02909646449615,-4.80230000983842,
73.5108200366566));
#63231=CARTESIAN_POINT('Ctrl Pts',(-3.260029560838,-3.72502426807083,73.4578997825747));
#63232=CARTESIAN_POINT('Ctrl Pts',(-4.31122810355742,-2.80504681907828,
73.4127066732687));
#63233=CARTESIAN_POINT('Ctrl Pts',(-4.9344881263814,-1.3960917881023,73.3675135639628));
#63234=CARTESIAN_POINT('Ctrl Pts',(-4.94622533435752,0.00372181280100414,
73.3223204546568));
#63235=CARTESIAN_POINT('Ctrl Pts',(-4.94548609638219,0.00396606047658106,
73.1776795453432));
#63236=CARTESIAN_POINT('Ctrl Pts',(-4.9334748398561,-1.37003547728531,73.2220220799872));
#63237=CARTESIAN_POINT('Ctrl Pts',(-4.33614096919029,-2.75319733775313,
73.2663646146311));
#63238=CARTESIAN_POINT('Ctrl Pts',(-3.3193311989464,-3.67227989433378,73.3107071492751));
#63239=CARTESIAN_POINT('Ctrl Pts',(-2.10582746429627,-4.76915184373973,
73.3636274033571));
#63240=CARTESIAN_POINT('Ctrl Pts',(-0.29486236375909,-5.2050336026263,73.416547657439));
#63241=CARTESIAN_POINT('Ctrl Pts',(1.28483881433472,-4.78045902103617,73.469467911521));
#63242=CARTESIAN_POINT('Ctrl Pts',(2.86453999242835,-4.35588443944609,73.522388165603));
#63243=CARTESIAN_POINT('Ctrl Pts',(4.21297724807857,-3.07085351737952,73.5753084196849));
#63244=CARTESIAN_POINT('Ctrl Pts',(4.71308509882384,-1.51341603066432,73.6282286737669));
#63245=CARTESIAN_POINT('Ctrl Pts',(5.21319294956918,0.0440214560510618,
73.6811489278489));
#63246=CARTESIAN_POINT('Ctrl Pts',(4.8649713954092,1.87386550741532,73.7340691819308));
#63247=CARTESIAN_POINT('Ctrl Pts',(3.82777193781054,3.13875153886656,73.7869894360128));
#63248=CARTESIAN_POINT('Ctrl Pts',(2.790572480212,4.40363757031766,73.8399096900947));
#63249=CARTESIAN_POINT('Ctrl Pts',(1.06439511917504,5.10356558185611,73.8928299441767));
#63250=CARTESIAN_POINT('Ctrl Pts',(-0.560835021503018,4.91823782561222,
73.9457501982587));
#63251=CARTESIAN_POINT('Ctrl Pts',(-2.18606516218117,4.73291006936832,73.9986704523406));
#63252=CARTESIAN_POINT('Ctrl Pts',(-3.71034808250029,3.662326545342,74.0515907064226));
#63253=CARTESIAN_POINT('Ctrl Pts',(-4.43614863820842,2.1964026248274,74.1045109605045));
#63254=CARTESIAN_POINT('Ctrl Pts',(-4.77065068257367,1.52079753684611,74.1289004887841));
#63255=CARTESIAN_POINT('Ctrl Pts',(-4.9355517737741,0.761220515306077,74.1532900170636));
#63256=CARTESIAN_POINT('Ctrl Pts',(-4.93410780896188,0.00104985362950368,
74.1776795453432));
#63257=CARTESIAN_POINT('Origin',(0.,0.,16.));
#63258=CARTESIAN_POINT('',(-4.94084634488987,-0.00449823523784309,75.3223204546568));
#63259=CARTESIAN_POINT('',(-4.94163609422309,-0.00451829382380276,75.1776795453432));
#63260=CARTESIAN_POINT('',(-4.942,-6.05220448138622E-16,16.));
#63261=CARTESIAN_POINT('Ctrl Pts',(-4.94084634488987,-0.00449823523784309,
75.3223204546568));
#63262=CARTESIAN_POINT('Ctrl Pts',(-4.92989311437387,1.21777170867941,75.2829696921977));
#63263=CARTESIAN_POINT('Ctrl Pts',(-4.47139568953686,2.44738194782565,75.2436189297386));
#63264=CARTESIAN_POINT('Ctrl Pts',(-3.64967329880456,3.34417154871685,75.2042681672795));
#63265=CARTESIAN_POINT('Ctrl Pts',(-2.54459286363954,4.55020494099322,75.1513479131975));
#63266=CARTESIAN_POINT('Ctrl Pts',(-0.782591300857919,5.15430584099797,
75.0984276591155));
#63267=CARTESIAN_POINT('Ctrl Pts',(0.83001256389233,4.88002845063787,75.0455074050336));
#63268=CARTESIAN_POINT('Ctrl Pts',(2.44261642864267,4.60575106027776,74.9925871509516));
#63269=CARTESIAN_POINT('Ctrl Pts',(3.90582259536151,3.45309537955268,74.9396668968697));
#63270=CARTESIAN_POINT('Ctrl Pts',(4.55004557505128,1.94953425212549,74.8867466427877));
#63271=CARTESIAN_POINT('Ctrl Pts',(5.19426855474108,0.445973124698207,74.8338263887057));
#63272=CARTESIAN_POINT('Ctrl Pts',(5.01950834740155,-1.40849344943142,74.7809061346238));
#63273=CARTESIAN_POINT('Ctrl Pts',(4.10573789297132,-2.76523324323168,74.7279858805418));
#63274=CARTESIAN_POINT('Ctrl Pts',(3.19196743854115,-4.12197303703186,74.6750656264599));
#63275=CARTESIAN_POINT('Ctrl Pts',(1.53918673702048,-4.98098605050295,74.6221453723779));
#63276=CARTESIAN_POINT('Ctrl Pts',(-0.0962665201530125,-4.94917480923354,
74.5692251182959));
#63277=CARTESIAN_POINT('Ctrl Pts',(-1.73171977732641,-4.91736356796412,
74.516304864214));
#63278=CARTESIAN_POINT('Ctrl Pts',(-3.34984559015253,-3.99472807195434,
74.463384610132));
#63279=CARTESIAN_POINT('Ctrl Pts',(-4.21016487353403,-2.60348041531225,
74.4104643560501));
#63280=CARTESIAN_POINT('Ctrl Pts',(-4.68781373971693,-1.8310603631163,74.3810830555857));
#63281=CARTESIAN_POINT('Ctrl Pts',(-4.93187137749265,-0.914192241399431,
74.3517017551212));
#63282=CARTESIAN_POINT('Ctrl Pts',(-4.93430944804537,0.00146807591443893,
74.3223204546568));
#63283=CARTESIAN_POINT('Ctrl Pts',(-4.93410780896188,0.00104985362950368,
74.1776795453432));
#63284=CARTESIAN_POINT('Ctrl Pts',(-4.93241866747241,-0.888193286408816,
74.2062102711456));
#63285=CARTESIAN_POINT('Ctrl Pts',(-4.70309992547236,-1.77824877440845,
74.234740996948));
#63286=CARTESIAN_POINT('Ctrl Pts',(-4.25136351730091,-2.53564734819139,
74.2632717227504));
#63287=CARTESIAN_POINT('Ctrl Pts',(-3.41345964958825,-3.94050908369249,
74.3161919768324));
#63288=CARTESIAN_POINT('Ctrl Pts',(-1.8103337230659,-4.88896823769192,74.3691122309144));
#63289=CARTESIAN_POINT('Ctrl Pts',(-0.175600645770052,-4.94699541578848,
74.4220324849964));
#63290=CARTESIAN_POINT('Ctrl Pts',(1.45913243152579,-5.00502259388504,74.4749527390783));
#63291=CARTESIAN_POINT('Ctrl Pts',(3.12547265959522,-4.17261779607872,74.5278729931603));
#63292=CARTESIAN_POINT('Ctrl Pts',(4.06087730056111,-2.83070217091354,74.5807932472422));
#63293=CARTESIAN_POINT('Ctrl Pts',(4.99628194152704,-1.48878654574829,74.6337135013242));
#63294=CARTESIAN_POINT('Ctrl Pts',(5.20075099538943,0.36263990677569,74.6866337554061));
#63295=CARTESIAN_POINT('Ctrl Pts',(4.58071630030657,1.87633616570506,74.7395540094881));
#63296=CARTESIAN_POINT('Ctrl Pts',(3.96068160522376,3.39003242463435,74.7924742635701));
#63297=CARTESIAN_POINT('Ctrl Pts',(2.51614316119567,4.56599848996891,74.8453945176521));
#63298=CARTESIAN_POINT('Ctrl Pts',(0.908143822210297,4.86609433003599,74.898314771734));
#63299=CARTESIAN_POINT('Ctrl Pts',(-0.699855516775171,5.16619017010308,
74.951235025816));
#63300=CARTESIAN_POINT('Ctrl Pts',(-2.47131575071806,4.59041578490263,75.0041552798979));
#63301=CARTESIAN_POINT('Ctrl Pts',(-3.59558962158726,3.4022543267312,75.0570755339799));
#63302=CARTESIAN_POINT('Ctrl Pts',(-4.44965416990239,2.49965701001681,75.097276871101));
#63303=CARTESIAN_POINT('Ctrl Pts',(-4.93023943833446,1.2436624400959,75.1374782082221));
#63304=CARTESIAN_POINT('Ctrl Pts',(-4.94163609422309,-0.00451829382380276,
75.1776795453432));
#63305=CARTESIAN_POINT('Origin',(0.,0.,16.));
#63306=CARTESIAN_POINT('',(-4.949709811623,0.00127385101247733,76.3223204546568));
#63307=CARTESIAN_POINT('',(-4.94936999019276,0.00173199160742904,76.1776795453431));
#63308=CARTESIAN_POINT('',(-4.942,-6.05220448138622E-16,16.));
#63309=CARTESIAN_POINT('Ctrl Pts',(-4.949709811623,0.00127385101247733,
76.3223204546568));
#63310=CARTESIAN_POINT('Ctrl Pts',(-4.94994903879905,0.0705988515890139,
76.3200781374381));
#63311=CARTESIAN_POINT('Ctrl Pts',(-4.94861862980554,0.139914463982202,
76.3178358202194));
#63312=CARTESIAN_POINT('Ctrl Pts',(-4.94569000143091,0.209162484687126,
76.3155935030007));
#63313=CARTESIAN_POINT('Ctrl Pts',(-4.87657232423312,1.84346418821971,76.2626732489188));
#63314=CARTESIAN_POINT('Ctrl Pts',(-3.91725763853945,3.44011779449909,76.2097529948368));
#63315=CARTESIAN_POINT('Ctrl Pts',(-2.50674299584768,4.26847022808205,76.1568327407548));
#63316=CARTESIAN_POINT('Ctrl Pts',(-1.09622835315598,5.09682266166495,76.1039124866729));
#63317=CARTESIAN_POINT('Ctrl Pts',(0.765486246533761,5.15687392255156,76.0509922325909));
#63318=CARTESIAN_POINT('Ctrl Pts',(2.22645176899709,4.4211436366153,75.9980719785089));
#63319=CARTESIAN_POINT('Ctrl Pts',(3.68741729146043,3.68541335067904,75.9451517244269));
#63320=CARTESIAN_POINT('Ctrl Pts',(4.74763373669735,2.15390151791992,75.892231470345));
#63321=CARTESIAN_POINT('Ctrl Pts',(4.92192986700097,0.527451343327534,75.8393112162631));
#63322=CARTESIAN_POINT('Ctrl Pts',(5.09622599730458,-1.09899883126485,75.7863909621811));
#63323=CARTESIAN_POINT('Ctrl Pts',(4.38460181267489,-2.8203873476905,75.7334707080991));
#63324=CARTESIAN_POINT('Ctrl Pts',(3.1127074084203,-3.84898053058463,75.6805504540171));
#63325=CARTESIAN_POINT('Ctrl Pts',(1.84081300416571,-4.87757371347876,75.6276301999351));
#63326=CARTESIAN_POINT('Ctrl Pts',(0.00864838028622472,-5.21337156284137,
75.5747099458532));
#63327=CARTESIAN_POINT('Ctrl Pts',(-1.54535994923236,-4.70270785426469,
75.5217896917713));
#63328=CARTESIAN_POINT('Ctrl Pts',(-3.09936827875094,-4.19204414568801,
75.4688694376893));
#63329=CARTESIAN_POINT('Ctrl Pts',(-4.37522031390861,-2.83491887917204,
75.4159491836074));
#63330=CARTESIAN_POINT('Ctrl Pts',(-4.78906667771331,-1.25237330364,75.3630289295254));
#63331=CARTESIAN_POINT('Ctrl Pts',(-4.89518266041626,-0.846586534424758,
75.3494594379025));
#63332=CARTESIAN_POINT('Ctrl Pts',(-4.94462339418807,-0.425978804568305,
75.3358899462797));
#63333=CARTESIAN_POINT('Ctrl Pts',(-4.94084634488987,-0.00449823523784309,
75.3223204546568));
#63334=CARTESIAN_POINT('Ctrl Pts',(-4.94163609422309,-0.00451829382380276,
75.1776795453432));
#63335=CARTESIAN_POINT('Ctrl Pts',(-4.94524177329398,-0.3994182708838,75.1903984623041));
#63336=CARTESIAN_POINT('Ctrl Pts',(-4.90188327382623,-0.793536109632625,
75.2031173792649));
#63337=CARTESIAN_POINT('Ctrl Pts',(-4.80852961499291,-1.17543275960954,
75.2158362962258));
#63338=CARTESIAN_POINT('Ctrl Pts',(-4.42010822973382,-2.76440985663659,
75.2687565503078));
#63339=CARTESIAN_POINT('Ctrl Pts',(-3.16617795142011,-4.14181551954833,
75.3216768043897));
#63340=CARTESIAN_POINT('Ctrl Pts',(-1.62055642630759,-4.6773278802945,75.3745970584716));
#63341=CARTESIAN_POINT('Ctrl Pts',(-0.0749349011951517,-5.21284024104065,
75.4275173125536));
#63342=CARTESIAN_POINT('Ctrl Pts',(1.76237787071597,-4.90645929962131,75.4804375666356));
#63343=CARTESIAN_POINT('Ctrl Pts',(3.05059950427476,-3.89838965409382,75.5333578207175));
#63344=CARTESIAN_POINT('Ctrl Pts',(4.3388211378337,-2.8903200085662,75.5862780747995));
#63345=CARTESIAN_POINT('Ctrl Pts',(5.07795163304007,-1.18056165893029,75.6391983288815));
#63346=CARTESIAN_POINT('Ctrl Pts',(4.92975358676999,0.448473861396107,75.6921185829634));
#63347=CARTESIAN_POINT('Ctrl Pts',(4.78155554049993,2.07750938172241,75.7450388370454));
#63348=CARTESIAN_POINT('Ctrl Pts',(3.74602895275332,3.62582207273939,75.7979590911274));
#63349=CARTESIAN_POINT('Ctrl Pts',(2.29704660536897,4.38488040012382,75.8508793452094));
#63350=CARTESIAN_POINT('Ctrl Pts',(0.848064257984615,5.14393872750825,75.9037995992913));
#63351=CARTESIAN_POINT('Ctrl Pts',(-1.0143738490375,5.11374269126039,75.9567198533733));
#63352=CARTESIAN_POINT('Ctrl Pts',(-2.43798759346781,4.30811045874223,76.0096401074552));
#63353=CARTESIAN_POINT('Ctrl Pts',(-3.86160133789813,3.50247822622406,76.0625603615372));
#63354=CARTESIAN_POINT('Ctrl Pts',(-4.84639071973656,1.92140979743563,76.1154806156192));
#63355=CARTESIAN_POINT('Ctrl Pts',(-4.94170107746221,0.28842623257243,76.1684008697011));
#63356=CARTESIAN_POINT('Ctrl Pts',(-4.94727143302206,0.192987506953041,
76.1714937615818));
#63357=CARTESIAN_POINT('Ctrl Pts',(-4.94980355369306,0.0973714523878282,
76.1745866534625));
#63358=CARTESIAN_POINT('Ctrl Pts',(-4.94936999019276,0.00173199160742904,
76.1776795453431));
#63359=CARTESIAN_POINT('Origin',(0.,0.,16.));
#63360=CARTESIAN_POINT('',(-4.93710573305067,0.00369191742993435,77.3223204546568));
#63361=CARTESIAN_POINT('',(-4.93651943436554,0.00342058198068374,77.1776795453431));
#63362=CARTESIAN_POINT('',(-4.942,-6.05220448138622E-16,16.));
#63363=CARTESIAN_POINT('Ctrl Pts',(-4.93710573305067,0.00369191742993435,
77.3223204546568));
#63364=CARTESIAN_POINT('Ctrl Pts',(-4.94100558540341,0.565545404544723,
77.3042663285965));
#63365=CARTESIAN_POINT('Ctrl Pts',(-4.85249197896959,1.12620708123838,77.2862122025363));
#63366=CARTESIAN_POINT('Ctrl Pts',(-4.66622450050179,1.65225526059718,77.2681580764761));
#63367=CARTESIAN_POINT('Ctrl Pts',(-4.12023726994686,3.19420767735372,77.2152378223941));
#63368=CARTESIAN_POINT('Ctrl Pts',(-2.73435528454182,4.43876323142188,77.1623175683121));
#63369=CARTESIAN_POINT('Ctrl Pts',(-1.14277930696628,4.81639429353784,77.1093973142302));
#63370=CARTESIAN_POINT('Ctrl Pts',(0.448796670609252,5.1940253556538,77.0564770601482));
#63371=CARTESIAN_POINT('Ctrl Pts',(2.24606664035538,4.70473192581759,77.0035568060662));
#63372=CARTESIAN_POINT('Ctrl Pts',(3.42657241495318,3.57242215035347,76.9506365519843));
#63373=CARTESIAN_POINT('Ctrl Pts',(4.60707818955111,2.44011237488923,76.8977162979023));
#63374=CARTESIAN_POINT('Ctrl Pts',(5.1708197690006,0.664786253797156,76.8447960438203));
#63375=CARTESIAN_POINT('Ctrl Pts',(4.85982039669027,-0.941139865890017,
76.7918757897384));
#63376=CARTESIAN_POINT('Ctrl Pts',(4.54882102437996,-2.54706598557701,76.7389555356564));
#63377=CARTESIAN_POINT('Ctrl Pts',(3.36308070030987,-3.983592103859,76.6860352815744));
#63378=CARTESIAN_POINT('Ctrl Pts',(1.84521230622943,-4.59334192937927,76.6331150274925));
#63379=CARTESIAN_POINT('Ctrl Pts',(0.327343912148982,-5.20309175489953,
76.5801947734105));
#63380=CARTESIAN_POINT('Ctrl Pts',(-1.52265255194192,-4.98606528765813,
76.5272745193286));
#63381=CARTESIAN_POINT('Ctrl Pts',(-2.85819044963632,-4.04157715364459,
76.4743542652466));
#63382=CARTESIAN_POINT('Ctrl Pts',(-4.13713943489684,-3.13710851769457,
76.4236763283833));
#63383=CARTESIAN_POINT('Ctrl Pts',(-4.94430311018814,-1.56551963073416,
76.3729983915201));
#63384=CARTESIAN_POINT('Ctrl Pts',(-4.949709811623,0.00127385101247733,
76.3223204546568));
#63385=CARTESIAN_POINT('Ctrl Pts',(-4.94936999019276,0.00173199160742904,
76.1776795453431));
#63386=CARTESIAN_POINT('Ctrl Pts',(-4.9423851596845,-1.5390467478049,76.2275069075444));
#63387=CARTESIAN_POINT('Ctrl Pts',(-4.16568308583621,-3.08590036450939,
76.2773342697457));
#63388=CARTESIAN_POINT('Ctrl Pts',(-2.92261878913845,-3.99523449174163,
76.327161631947));
#63389=CARTESIAN_POINT('Ctrl Pts',(-1.60239480947616,-4.96101295025462,
76.380081886029));
#63390=CARTESIAN_POINT('Ctrl Pts',(0.243884483461281,-5.20767116634268,
76.4330021401109));
#63391=CARTESIAN_POINT('Ctrl Pts',(1.77133348755807,-4.62233457318728,76.4859223941929));
#63392=CARTESIAN_POINT('Ctrl Pts',(3.29878249165486,-4.03699798003188,76.5388426482749));
#63393=CARTESIAN_POINT('Ctrl Pts',(4.507401206911,-2.61966657763301,76.5917629023568));
#63394=CARTESIAN_POINT('Ctrl Pts',(4.84410725035561,-1.01893286220407,76.6446831564388));
#63395=CARTESIAN_POINT('Ctrl Pts',(5.18081329380023,0.581800853224953,76.6976034105207));
#63396=CARTESIAN_POINT('Ctrl Pts',(4.64560666543322,2.36593688168406,76.7505236646027));
#63397=CARTESIAN_POINT('Ctrl Pts',(3.483406092445,3.51702732797801,76.8034439186847));
#63398=CARTESIAN_POINT('Ctrl Pts',(2.32120551945685,4.6681177742719,76.8563641727667));
#63399=CARTESIAN_POINT('Ctrl Pts',(0.532011001847567,5.1861626384007,76.9092844268486));
#63400=CARTESIAN_POINT('Ctrl Pts',(-1.06541472329578,4.83409667859588,76.9622046809306));
#63401=CARTESIAN_POINT('Ctrl Pts',(-2.66284044843913,4.48203071879105,77.0151249350126));
#63402=CARTESIAN_POINT('Ctrl Pts',(-4.06849738111654,3.2598539350526,77.0680451890945));
#63403=CARTESIAN_POINT('Ctrl Pts',(-4.63913544075982,1.72685308955721,77.1209654431764));
#63404=CARTESIAN_POINT('Ctrl Pts',(-4.84298445708464,1.17921924512925,77.1398701438987));
#63405=CARTESIAN_POINT('Ctrl Pts',(-4.94027400061573,0.591920131780996,
77.1587748446209));
#63406=CARTESIAN_POINT('Ctrl Pts',(-4.93651943436554,0.00342058198068374,
77.1776795453431));
#63407=CARTESIAN_POINT('Origin',(0.,0.,16.));
#63408=CARTESIAN_POINT('',(-4.93642136366389,-0.0033694929564293,78.3223204546568));
#63409=CARTESIAN_POINT('',(-4.93699915860479,-0.00364661157755484,78.1776795453431));
#63410=CARTESIAN_POINT('',(-4.942,-6.05220448138622E-16,16.));
#63411=CARTESIAN_POINT('Ctrl Pts',(-4.93642136366389,-0.0033694929564293,
78.3223204546568));
#63412=CARTESIAN_POINT('Ctrl Pts',(-4.92980420575396,1.05092284524382,78.288454519755));
#63413=CARTESIAN_POINT('Ctrl Pts',(-4.59907343284897,2.10900469043804,78.2545885848532));
#63414=CARTESIAN_POINT('Ctrl Pts',(-3.975312192884,2.94965955736624,78.2207226499514));
#63415=CARTESIAN_POINT('Ctrl Pts',(-3.00059812102546,4.26330021964482,78.1678023958694));
#63416=CARTESIAN_POINT('Ctrl Pts',(-1.31034971100207,5.04601837903923,78.1148821417875));
#63417=CARTESIAN_POINT('Ctrl Pts',(0.321949550104491,4.93963025159188,78.0619618877055));
#63418=CARTESIAN_POINT('Ctrl Pts',(1.95424881121096,4.83324212414454,78.0090416336236));
#63419=CARTESIAN_POINT('Ctrl Pts',(3.52859892340051,3.83774770985554,77.9561213795416));
#63420=CARTESIAN_POINT('Ctrl Pts',(4.32455323076013,2.40870045658987,77.9032011254596));
#63421=CARTESIAN_POINT('Ctrl Pts',(5.12050753811972,0.979653203324283,77.8502808713777));
#63422=CARTESIAN_POINT('Ctrl Pts',(5.13806604064937,-0.882946888918111,
77.7973606172957));
#63423=CARTESIAN_POINT('Ctrl Pts',(4.36919369942578,-2.32674557099659,77.7444403632137));
#63424=CARTESIAN_POINT('Ctrl Pts',(3.60032135820212,-3.77054425307524,77.6915201091318));
#63425=CARTESIAN_POINT('Ctrl Pts',(2.04501817322514,-4.79554152499005,77.6385998550498));
#63426=CARTESIAN_POINT('Ctrl Pts',(0.415014635617477,-4.93268298063817,
77.5856796009678));
#63427=CARTESIAN_POINT('Ctrl Pts',(-1.21498890199009,-5.06982443628629,
77.5327593468859));
#63428=CARTESIAN_POINT('Ctrl Pts',(-2.91969279222824,-4.3191100756678,77.4798390928039));
#63429=CARTESIAN_POINT('Ctrl Pts',(-3.91899849949491,-3.02407825563606,
77.4269188387219));
#63430=CARTESIAN_POINT('Ctrl Pts',(-4.57738386303512,-2.17085587390878,
77.3920527107002));
#63431=CARTESIAN_POINT('Ctrl Pts',(-4.92957433823582,-1.08135952985832,
77.3571865826785));
#63432=CARTESIAN_POINT('Ctrl Pts',(-4.93710573305067,0.00369191742993435,
77.3223204546568));
#63433=CARTESIAN_POINT('Ctrl Pts',(-4.93651943436554,0.00342058198068374,
77.1776795453431));
#63434=CARTESIAN_POINT('Ctrl Pts',(-4.92976377869543,-1.05547678606275,
77.2116950987028));
#63435=CARTESIAN_POINT('Ctrl Pts',(-4.59587353108828,-2.11826061804498,
77.2457106520626));
#63436=CARTESIAN_POINT('Ctrl Pts',(-3.96697769860343,-2.96085919445861,
77.2797262054223));
#63437=CARTESIAN_POINT('Ctrl Pts',(-2.98856271019464,-4.27174572572668,
77.3326464595043));
#63438=CARTESIAN_POINT('Ctrl Pts',(-1.29611354676788,-5.0496938810105,77.3855667135863));
#63439=CARTESIAN_POINT('Ctrl Pts',(0.335879206226305,-4.93870270308427,
77.4384869676682));
#63440=CARTESIAN_POINT('Ctrl Pts',(1.96787195922058,-4.82771152515804,77.4914072217502));
#63441=CARTESIAN_POINT('Ctrl Pts',(3.53940830178236,-3.82778101402163,77.5443274758322));
#63442=CARTESIAN_POINT('Ctrl Pts',(4.33132920195393,-2.39649464320875,77.5972477299141));
#63443=CARTESIAN_POINT('Ctrl Pts',(5.12325010212551,-0.96520827239587,77.6501679839961));
#63444=CARTESIAN_POINT('Ctrl Pts',(5.13555555990697,0.897433958093309,77.7030882380781));
#63445=CARTESIAN_POINT('Ctrl Pts',(4.36261440987998,2.33905851601337,77.75600849216));
#63446=CARTESIAN_POINT('Ctrl Pts',(3.58967325985303,3.78068307393336,77.808928746242));
#63447=CARTESIAN_POINT('Ctrl Pts',(2.03148550201762,4.8012899592841,77.8618490003239));
#63448=CARTESIAN_POINT('Ctrl Pts',(0.40110165209169,4.93383387390743,77.9147692544059));
#63449=CARTESIAN_POINT('Ctrl Pts',(-1.22928219783424,5.06637778853077,77.9676895084879));
#63450=CARTESIAN_POINT('Ctrl Pts',(-2.93186213985079,4.31085873242671,78.0206097625698));
#63451=CARTESIAN_POINT('Ctrl Pts',(-3.92751158950039,3.01301376448353,78.0735300166518));
#63452=CARTESIAN_POINT('Ctrl Pts',(-4.58067311036902,2.16160728461073,78.1082465262156));
#63453=CARTESIAN_POINT('Ctrl Pts',(-4.92960256861,1.07680737701515,78.1429630357793));
#63454=CARTESIAN_POINT('Ctrl Pts',(-4.93699915860479,-0.00364661157755484,
78.1776795453431));
#63455=CARTESIAN_POINT('Origin',(0.,0.,16.));
#63456=CARTESIAN_POINT('',(-4.94930076406873,-0.0018103975202266,79.3223204546568));
#63457=CARTESIAN_POINT('',(-4.94965689841004,-0.00135584006909748,79.1776795453431));
#63458=CARTESIAN_POINT('',(-4.942,-6.05220448138622E-16,16.));
#63459=CARTESIAN_POINT('Ctrl Pts',(-4.94930076406873,-0.0018103975202266,
79.3223204546568));
#63460=CARTESIAN_POINT('Ctrl Pts',(-4.94206344439878,1.53439887470602,79.2726427109135));
#63461=CARTESIAN_POINT('Ctrl Pts',(-4.17064455342085,3.07688083896746,79.2229649671701));
#63462=CARTESIAN_POINT('Ctrl Pts',(-2.93387463574621,3.9869760667678,79.1732872234267));
#63463=CARTESIAN_POINT('Ctrl Pts',(-1.61637965001588,4.95647401624775,79.1203669693448));
#63464=CARTESIAN_POINT('Ctrl Pts',(0.229196639493549,5.20833819439267,79.0674467152628));
#63465=CARTESIAN_POINT('Ctrl Pts',(1.75829033577168,4.62731170663768,79.0145264611808));
#63466=CARTESIAN_POINT('Ctrl Pts',(3.28738403204981,4.04628521888269,78.9616062070989));
#63467=CARTESIAN_POINT('Ctrl Pts',(4.49999513509664,2.6323680652278,78.9086859530169));
#63468=CARTESIAN_POINT('Ctrl Pts',(4.84121428431374,1.03259032951638,78.8557656989349));
#63469=CARTESIAN_POINT('Ctrl Pts',(5.18243343353085,-0.567187406195048,
78.802845444853));
#63470=CARTESIAN_POINT('Ctrl Pts',(4.65226062891823,-2.35282572396301,78.749925190771));
#63471=CARTESIAN_POINT('Ctrl Pts',(3.49331104303619,-3.50718925806059,78.6970049366891));
#63472=CARTESIAN_POINT('Ctrl Pts',(2.33436145715409,-4.66155279215825,78.6440846826071));
#63473=CARTESIAN_POINT('Ctrl Pts',(0.546635090002505,-5.18464154258545,
78.5911644285251));
#63474=CARTESIAN_POINT('Ctrl Pts',(-1.05177716940348,-4.83708210816974,
78.5382441744432));
#63475=CARTESIAN_POINT('Ctrl Pts',(-2.65018942880937,-4.48952267375405,
78.4853239203612));
#63476=CARTESIAN_POINT('Ctrl Pts',(-4.05928758046969,-3.27131505449554,
78.4324036662792));
#63477=CARTESIAN_POINT('Ctrl Pts',(-4.63424678945294,-1.73992966228502,
78.3794834121973));
#63478=CARTESIAN_POINT('Ctrl Pts',(-4.84126499965602,-1.18854330639521,
78.3604290930171));
#63479=CARTESIAN_POINT('Ctrl Pts',(-4.94014443935181,-0.596556209328453,
78.3413747738369));
#63480=CARTESIAN_POINT('Ctrl Pts',(-4.93642136366389,-0.0033694929564293,
78.3223204546568));
#63481=CARTESIAN_POINT('Ctrl Pts',(-4.93699915860479,-0.00364661157755484,
78.1776795453431));
#63482=CARTESIAN_POINT('Ctrl Pts',(-4.94087759097782,-0.57018710251793,
78.1958832898613));
#63483=CARTESIAN_POINT('Ctrl Pts',(-4.85085250590991,-1.13553269504931,
78.2140870343795));
#63484=CARTESIAN_POINT('Ctrl Pts',(-4.66154625697823,-1.66540857589943,
78.2322907788976));
#63485=CARTESIAN_POINT('Ctrl Pts',(-4.11121251752373,-3.20581506855694,
78.2852110329796));
#63486=CARTESIAN_POINT('Ctrl Pts',(-2.72182608133198,-4.44645717408944,
78.3381312870616));
#63487=CARTESIAN_POINT('Ctrl Pts',(-1.12919140128498,-4.819598117052,78.3910515411436));
#63488=CARTESIAN_POINT('Ctrl Pts',(0.463443278761841,-5.19273906001451,
78.4439717952256));
#63489=CARTESIAN_POINT('Ctrl Pts',(2.25932620266378,-4.69837884040726,78.4968920493075));
#63490=CARTESIAN_POINT('Ctrl Pts',(3.43663391646442,-3.56274424493725,78.5498123033895));
#63491=CARTESIAN_POINT('Ctrl Pts',(4.6139416302652,-2.42710964946711,78.6027325574714));
#63492=CARTESIAN_POINT('Ctrl Pts',(5.17267413396446,-0.65020067813383,78.6556528115534));
#63493=CARTESIAN_POINT('Ctrl Pts',(4.85714690051601,0.954841985584431,78.7085730656353));
#63494=CARTESIAN_POINT('Ctrl Pts',(4.54161966706758,2.5598846493026,78.7614933197173));
#63495=CARTESIAN_POINT('Ctrl Pts',(3.35183269647175,3.99306100540591,78.8144135737993));
#63496=CARTESIAN_POINT('Ctrl Pts',(1.83225067773116,4.59852766487066,78.8673338278812));
#63497=CARTESIAN_POINT('Ctrl Pts',(0.312668658990661,5.20399432433538,78.9202540819632));
#63498=CARTESIAN_POINT('Ctrl Pts',(-1.53670840789443,4.98175128716162,78.9731743360452));
#63499=CARTESIAN_POINT('Ctrl Pts',(-2.86957733213866,4.03350036141105,79.0260945901271));
#63500=CARTESIAN_POINT('Ctrl Pts',(-4.14220208735026,3.12810930583763,79.0766229085325));
#63501=CARTESIAN_POINT('Ctrl Pts',(-4.94395467452422,1.56085664483311,79.1271512269378));
#63502=CARTESIAN_POINT('Ctrl Pts',(-4.94965689841004,-0.00135584006909748,
79.1776795453431));
#63503=CARTESIAN_POINT('Origin',(0.,0.,16.));
#63504=CARTESIAN_POINT('',(-4.94177616066966,0.00451715357047341,80.3223204546568));
#63505=CARTESIAN_POINT('',(-4.94098429374081,0.00450501606805162,80.1776795453432));
#63506=CARTESIAN_POINT('',(-4.942,-6.05220448138622E-16,16.));
#63507=CARTESIAN_POINT('Ctrl Pts',(-4.94177616066966,0.00451715357047341,
80.3223204546568));
#63508=CARTESIAN_POINT('Ctrl Pts',(-4.94534763047119,0.394743465756727,
80.3097511561539));
#63509=CARTESIAN_POINT('Ctrl Pts',(-4.90301618269456,0.784203971238864,
80.2971818576509));
#63510=CARTESIAN_POINT('Ctrl Pts',(-4.81182542362119,1.16186687182505,80.284612559148));
#63511=CARTESIAN_POINT('Ctrl Pts',(-4.42788688170829,2.75193306777578,80.231692305066));
#63512=CARTESIAN_POINT('Ctrl Pts',(-3.17784621930909,4.13286961482545,80.178772050984));
#63513=CARTESIAN_POINT('Ctrl Pts',(-1.63374113503097,4.67273885841708,80.125851796902));
#63514=CARTESIAN_POINT('Ctrl Pts',(-0.0896360507527699,5.21260810200875,
80.07293154282));
#63515=CARTESIAN_POINT('Ctrl Pts',(1.74853345540447,4.91141004214231,80.0200112887381));
#63516=CARTESIAN_POINT('Ctrl Pts',(3.03959294361313,3.90697751111939,79.9670910346562));
#63517=CARTESIAN_POINT('Ctrl Pts',(4.33065243182171,2.90254498009653,79.9141707805742));
#63518=CARTESIAN_POINT('Ctrl Pts',(5.0746019020818,1.1948779779175,79.8612505264923));
#63519=CARTESIAN_POINT('Ctrl Pts',(4.93099871468662,-0.43456899453677,79.8083302724103));
#63520=CARTESIAN_POINT('Ctrl Pts',(4.78739552729143,-2.06401596699104,79.7554100183283));
#63521=CARTESIAN_POINT('Ctrl Pts',(3.7562396822408,-3.61524290972046,79.7024897642464));
#63522=CARTESIAN_POINT('Ctrl Pts',(2.30940384276248,-4.37838468231013,79.6495695101644));
#63523=CARTESIAN_POINT('Ctrl Pts',(0.86256800328416,-5.14152645489981,79.5966492560824));
#63524=CARTESIAN_POINT('Ctrl Pts',(-0.999947830621951,-5.1165830573498,
79.5437290020005));
#63525=CARTESIAN_POINT('Ctrl Pts',(-2.4258279677168,-4.31496896933192,79.4908087479185));
#63526=CARTESIAN_POINT('Ctrl Pts',(-3.85170810481173,-3.51335488131399,
79.4378884938365));
#63527=CARTESIAN_POINT('Ctrl Pts',(-4.84095254509543,-1.93507010282805,
79.3849682397546));
#63528=CARTESIAN_POINT('Ctrl Pts',(-4.9408679242616,-0.302361853177563,
79.3320479856726));
#63529=CARTESIAN_POINT('Ctrl Pts',(-4.94698990261473,-0.202323153982769,
79.328805475334));
#63530=CARTESIAN_POINT('Ctrl Pts',(-4.94977315033439,-0.10208013749047,
79.3255629649954));
#63531=CARTESIAN_POINT('Ctrl Pts',(-4.94930076406873,-0.0018103975202266,
79.3223204546568));
#63532=CARTESIAN_POINT('Ctrl Pts',(-4.94965689841004,-0.00135584006909748,
79.1776795453431));
#63533=CARTESIAN_POINT('Ctrl Pts',(-4.9499268332343,-0.0753086628631314,
79.1800714810198));
#63534=CARTESIAN_POINT('Ctrl Pts',(-4.94841287075996,-0.149250190949008,
79.1824634166964));
#63535=CARTESIAN_POINT('Ctrl Pts',(-4.94508051525459,-0.223109677684533,
79.184855352373));
#63536=CARTESIAN_POINT('Ctrl Pts',(-4.87135399252289,-1.85720997670206,
79.237775606455));
#63537=CARTESIAN_POINT('Ctrl Pts',(-3.90754016545605,-3.45115176040958,
79.290695860537));
#63538=CARTESIAN_POINT('Ctrl Pts',(-2.49469496135826,-4.27552292478954,
79.3436161146189));
#63539=CARTESIAN_POINT('Ctrl Pts',(-1.08184975726055,-5.09989408916944,
79.3965363687009));
#63540=CARTESIAN_POINT('Ctrl Pts',(0.780026823868144,-5.15469463422192,
79.4494566227829));
#63541=CARTESIAN_POINT('Ctrl Pts',(2.23891162262289,-4.41484699357874,79.5023768768648));
#63542=CARTESIAN_POINT('Ctrl Pts',(3.69779642137764,-3.67499935293556,79.5552971309468));
#63543=CARTESIAN_POINT('Ctrl Pts',(4.75368943775855,-2.14050352659667,79.6082173850287));
#63544=CARTESIAN_POINT('Ctrl Pts',(4.92339790113362,-0.51356824058747,79.6611376391107));
#63545=CARTESIAN_POINT('Ctrl Pts',(5.0931063645087,1.11336704542182,79.7140578931926));
#63546=CARTESIAN_POINT('Ctrl Pts',(4.37663027487802,2.83274179110132,79.7669781472746));
#63547=CARTESIAN_POINT('Ctrl Pts',(3.10184003337994,3.85774385333563,79.8198984013566));
#63548=CARTESIAN_POINT('Ctrl Pts',(1.82704979188194,4.88274591556987,79.8728186554386));
#63549=CARTESIAN_POINT('Ctrl Pts',(-0.00605460148340203,5.21337529435879,
79.9257389095204));
#63550=CARTESIAN_POINT('Ctrl Pts',(-1.55861657986055,4.69833093636568,79.9786591636024));
#63551=CARTESIAN_POINT('Ctrl Pts',(-3.11117855823778,4.18328657837255,80.0315794176844));
#63552=CARTESIAN_POINT('Ctrl Pts',(-4.38319812162688,2.82256848359726,80.0844996717665));
#63553=CARTESIAN_POINT('Ctrl Pts',(-4.79257969064933,1.23886203404666,80.1374199258484));
#63554=CARTESIAN_POINT('Ctrl Pts',(-4.89639341618109,0.837255124705079,
80.1508397990133));
#63555=CARTESIAN_POINT('Ctrl Pts',(-4.94473415317796,0.421308677192607,
80.1642596721782));
#63556=CARTESIAN_POINT('Ctrl Pts',(-4.94098429374081,0.00450501606805162,
80.1776795453432));
#63557=CARTESIAN_POINT('Origin',(0.,0.,16.));
#63558=CARTESIAN_POINT('',(-4.93407925753408,-0.000975201913082646,81.3223204546568));
#63559=CARTESIAN_POINT('',(-4.93426916398102,-0.00139536187133696,81.1776795453431));
#63560=CARTESIAN_POINT('',(-4.942,-6.05220448138622E-16,16.));
#63561=CARTESIAN_POINT('Ctrl Pts',(-4.93407925753408,-0.000975201913082646,
81.3223204546568));
#63562=CARTESIAN_POINT('Ctrl Pts',(-4.93251895945243,0.883617373199263,
81.2939393473123));
#63563=CARTESIAN_POINT('Ctrl Pts',(-4.70573849196771,1.76895636928203,81.2655582399678));
#63564=CARTESIAN_POINT('Ctrl Pts',(-4.25849767807825,2.52364737255269,81.2371771326233));
#63565=CARTESIAN_POINT('Ctrl Pts',(-3.42455919852679,3.93086658925474,81.1842568785413));
#63566=CARTESIAN_POINT('Ctrl Pts',(-1.8241145504932,4.88384315405391,81.1313366244594));
#63567=CARTESIAN_POINT('Ctrl Pts',(-0.189551647970844,4.94648043642473,
81.0784163703775));
#63568=CARTESIAN_POINT('Ctrl Pts',(1.44501125455142,5.00911771879556,81.0254961162955));
#63569=CARTESIAN_POINT('Ctrl Pts',(3.11369241156233,4.18141571873815,80.9725758622135));
#63570=CARTESIAN_POINT('Ctrl Pts',(4.05287784031979,2.84214351269564,80.9196556081315));
#63571=CARTESIAN_POINT('Ctrl Pts',(4.99206326907725,1.50287130665312,80.8667353540495));
#63572=CARTESIAN_POINT('Ctrl Pts',(5.20175296958118,-0.347971105374417,
80.8138150999676));
#63573=CARTESIAN_POINT('Ctrl Pts',(4.58598973236862,-1.86340996827063,80.7608948458856));
#63574=CARTESIAN_POINT('Ctrl Pts',(3.97022649515609,-3.37884883116675,80.7079745918037));
#63575=CARTESIAN_POINT('Ctrl Pts',(2.52901032022692,-4.5588841449317,80.6550543377218));
#63576=CARTESIAN_POINT('Ctrl Pts',(0.92186374048162,-4.86351372766964,80.6021340836398));
#63577=CARTESIAN_POINT('Ctrl Pts',(-0.685282839263774,-5.16814331040758,
80.5492138295578));
#63578=CARTESIAN_POINT('Ctrl Pts',(-2.45835982382543,-4.59736716211862,
80.4962935754758));
#63579=CARTESIAN_POINT('Ctrl Pts',(-3.58598010539301,-3.41238116554821,
80.4433733213938));
#63580=CARTESIAN_POINT('Ctrl Pts',(-4.44577484147009,-2.5088458719475,80.4030223658148));
#63581=CARTESIAN_POINT('Ctrl Pts',(-4.93031074601031,-1.24821819877227,
80.3626714102358));
#63582=CARTESIAN_POINT('Ctrl Pts',(-4.94177616066966,0.00451715357047341,
80.3223204546568));
#63583=CARTESIAN_POINT('Ctrl Pts',(-4.94098429374081,0.00450501606805162,
80.1776795453432));
#63584=CARTESIAN_POINT('Ctrl Pts',(-4.92994686631264,-1.22232501277905,
80.2171799262602));
#63585=CARTESIAN_POINT('Ctrl Pts',(-4.46760970741441,-2.45658172320469,
80.2566803071772));
#63586=CARTESIAN_POINT('Ctrl Pts',(-3.64022747730309,-3.35445124336543,
80.2961806880942));
#63587=CARTESIAN_POINT('Ctrl Pts',(-2.53175012027843,-4.55736326690124,
80.3491009421762));
#63588=CARTESIAN_POINT('Ctrl Pts',(-0.768051831573162,-5.1564925096469,
80.4020211962582));
#63589=CARTESIAN_POINT('Ctrl Pts',(0.843772115467599,-4.87766827980189,
80.4549414503402));
#63590=CARTESIAN_POINT('Ctrl Pts',(2.45559606250818,-4.59884404995691,80.5078617044222));
#63591=CARTESIAN_POINT('Ctrl Pts',(3.91554566788429,-3.4420663475215,80.5607819585041));
#63592=CARTESIAN_POINT('Ctrl Pts',(4.55552569480652,-1.93669431624669,80.613702212586));
#63593=CARTESIAN_POINT('Ctrl Pts',(5.19550572172878,-0.431322284971791,
80.666622466668));
#63594=CARTESIAN_POINT('Ctrl Pts',(5.01551617019705,1.42264407514254,80.71954272075));
#63595=CARTESIAN_POINT('Ctrl Pts',(4.09792300791601,2.7768014426365,80.7724629748319));
#63596=CARTESIAN_POINT('Ctrl Pts',(3.18032984563491,4.13095881013054,80.8253832289139));
#63597=CARTESIAN_POINT('Ctrl Pts',(1.52513307260442,4.98530718500416,80.8783034829959));
#63598=CARTESIAN_POINT('Ctrl Pts',(-0.110223988510079,4.94888370271273,
80.9312237370779));
#63599=CARTESIAN_POINT('Ctrl Pts',(-1.74558104962448,4.9124602204213,80.9841439911598));
#63600=CARTESIAN_POINT('Ctrl Pts',(-3.36109839882289,3.98526488096493,81.0370642452417));
#63601=CARTESIAN_POINT('Ctrl Pts',(-4.21749062381118,2.59159643244825,81.0899844993237));
#63602=CARTESIAN_POINT('Ctrl Pts',(-4.69053795942863,1.82177259814856,81.1192161813301));
#63603=CARTESIAN_POINT('Ctrl Pts',(-4.93196472022524,0.909620752018895,
81.1484478633366));
#63604=CARTESIAN_POINT('Ctrl Pts',(-4.93426916398102,-0.00139536187133696,
81.1776795453431));
#63605=CARTESIAN_POINT('Origin',(0.,0.,16.));
#63606=CARTESIAN_POINT('',(-4.94535283272668,-0.00400458364991862,82.3223204546568));
#63607=CARTESIAN_POINT('',(-4.94609777444767,-0.00376784846301249,82.1776795453432));
#63608=CARTESIAN_POINT('',(-4.942,-6.05220448138622E-16,16.));
#63609=CARTESIAN_POINT('Ctrl Pts',(-4.94535283272668,-0.00400458364991862,
82.3223204546568));
#63610=CARTESIAN_POINT('Ctrl Pts',(-4.93330953662462,1.36545649397123,82.2781275384708));
#63611=CARTESIAN_POINT('Ctrl Pts',(-4.34046622285376,2.74406818932791,82.2339346222847));
#63612=CARTESIAN_POINT('Ctrl Pts',(-3.32967465270896,3.66290393572493,82.1897417060986));
#63613=CARTESIAN_POINT('Ctrl Pts',(-2.11926920015238,4.76319387708596,82.1368214520167));
#63614=CARTESIAN_POINT('Ctrl Pts',(-0.309540619040862,5.20418124698654,
82.0839011979348));
#63615=CARTESIAN_POINT('Ctrl Pts',(1.27135165523017,4.78406349239674,82.0309809438528));
#63616=CARTESIAN_POINT('Ctrl Pts',(2.85224392950138,4.3639457378069,81.9780606897708));
#63617=CARTESIAN_POINT('Ctrl Pts',(4.20429989693216,3.08272285872646,81.9251404356888));
#63618=CARTESIAN_POINT('Ctrl Pts',(4.7087980958408,1.52670201104665,81.8722201816068));
#63619=CARTESIAN_POINT('Ctrl Pts',(5.21329629474935,-0.0293188366329011,
81.8192999275248));
#63620=CARTESIAN_POINT('Ctrl Pts',(4.87023672513615,-1.86013765291182,81.7663796734429));
#63621=CARTESIAN_POINT('Ctrl Pts',(3.83660868625431,-3.12794378523385,81.713459419361));
#63622=CARTESIAN_POINT('Ctrl Pts',(2.80298064737236,-4.39574991755603,81.660539165279));
#63623=CARTESIAN_POINT('Ctrl Pts',(1.07878413922189,-5.10054336592114,81.607618911197));
#63624=CARTESIAN_POINT('Ctrl Pts',(-0.546962183326737,-4.91979988461579,
81.554698657115));
#63625=CARTESIAN_POINT('Ctrl Pts',(-2.17270850587518,-4.73905640331046,
81.5017784030331));
#63626=CARTESIAN_POINT('Ctrl Pts',(-3.70000464282163,-3.6727759923347,81.4488581489512));
#63627=CARTESIAN_POINT('Ctrl Pts',(-4.42993655576027,-2.20890485254455,
81.3959378948692));
#63628=CARTESIAN_POINT('Ctrl Pts',(-4.7684063275082,-1.53010711570026,81.3713987481318));
#63629=CARTESIAN_POINT('Ctrl Pts',(-4.93542833750884,-0.765820165151225,
81.3468596013943));
#63630=CARTESIAN_POINT('Ctrl Pts',(-4.93407925753408,-0.000975201913082646,
81.3223204546568));
#63631=CARTESIAN_POINT('Ctrl Pts',(-4.93426916398102,-0.00139536187133696,
81.1776795453431));
#63632=CARTESIAN_POINT('Ctrl Pts',(-4.93613662347209,-0.739658417382295,
81.2013681174186));
#63633=CARTESIAN_POINT('Ctrl Pts',(-4.78097132279663,-1.47717563214288,
81.2250566894941));
#63634=CARTESIAN_POINT('Ctrl Pts',(-4.46478101528126,-2.13759905414229,
81.2487452615696));
#63635=CARTESIAN_POINT('Ctrl Pts',(-3.75841208098482,-3.61298453463955,
81.3016655156515));
#63636=CARTESIAN_POINT('Ctrl Pts',(-2.24840711161364,-4.7036139380569,81.3545857697334));
#63637=CARTESIAN_POINT('Ctrl Pts',(-0.625767443036273,-4.91039859255742,
81.4075060238154));
#63638=CARTESIAN_POINT('Ctrl Pts',(0.996872225541001,-5.11718324705793,
81.4604262778974));
#63639=CARTESIAN_POINT('Ctrl Pts',(2.73214659332435,-4.44012315264172,81.5133465319795));
#63640=CARTESIAN_POINT('Ctrl Pts',(3.7859676073568,-3.18905134900772,81.5662667860614));
#63641=CARTESIAN_POINT('Ctrl Pts',(4.83978862138919,-1.9379795453738,81.6191870401434));
#63642=CARTESIAN_POINT('Ctrl Pts',(5.21215628167071,-0.112896032521955,
81.6721072942252));
#63643=CARTESIAN_POINT('Ctrl Pts',(4.7326694596758,1.45101310003748,81.7250275483072));
#63644=CARTESIAN_POINT('Ctrl Pts',(4.25318263768082,3.01492223259719,81.7779478023891));
#63645=CARTESIAN_POINT('Ctrl Pts',(2.92184133340926,4.31765698486456,81.8308680564712));
#63646=CARTESIAN_POINT('Ctrl Pts',(1.34788766110338,4.7630660380761,81.8837883105532));
#63647=CARTESIAN_POINT('Ctrl Pts',(-0.226066011202234,5.20847509128757,
81.9367085646351));
#63648=CARTESIAN_POINT('Ctrl Pts',(-2.04263205154196,4.79655844544351,81.989628818717));
#63649=CARTESIAN_POINT('Ctrl Pts',(-3.27052209643622,3.71581544847434,82.042549072799));
#63650=CARTESIAN_POINT('Ctrl Pts',(-4.31565037405029,2.79593253903751,82.087592563647));
#63651=CARTESIAN_POINT('Ctrl Pts',(-4.93430071630666,1.39150518826543,82.1326360544951));
#63652=CARTESIAN_POINT('Ctrl Pts',(-4.94609777444767,-0.00376784846301249,
82.1776795453432));
#63653=CARTESIAN_POINT('Origin',(0.,0.,16.));
#63654=CARTESIAN_POINT('',(-4.94676006163664,0.00350952918951444,83.3223204546568));
#63655=CARTESIAN_POINT('',(-4.94604776483535,0.00378542647206983,83.1776795453431));
#63656=CARTESIAN_POINT('',(-4.942,-6.05220448138622E-16,16.));
#63657=CARTESIAN_POINT('Ctrl Pts',(-4.94676006163664,0.00350952918951444,
83.3223204546568));
#63658=CARTESIAN_POINT('Ctrl Pts',(-4.94852531327494,0.222882433779423,
83.3152359837111));
#63659=CARTESIAN_POINT('Ctrl Pts',(-4.93519531289187,0.442039477932862,
83.3081515127655));
#63660=CARTESIAN_POINT('Ctrl Pts',(-4.90603966821321,0.659070530865341,
83.3010670418199));
#63661=CARTESIAN_POINT('Ctrl Pts',(-4.68825006385762,2.28026970762846,83.2481467877379));
#63662=CARTESIAN_POINT('Ctrl Pts',(-3.58740009065817,3.78283999594482,83.1952265336559));
#63663=CARTESIAN_POINT('Ctrl Pts',(-2.10725577029135,4.47918204688364,83.1423062795739));
#63664=CARTESIAN_POINT('Ctrl Pts',(-0.627111449924431,5.1755240978225,83.089386025492));
#63665=CARTESIAN_POINT('Ctrl Pts',(1.23232721760991,5.06563791138373,83.0364657714101));
#63666=CARTESIAN_POINT('Ctrl Pts',(2.62015283567102,4.19980920832437,82.9835455173281));
#63667=CARTESIAN_POINT('Ctrl Pts',(4.00797845373196,3.33398050526512,82.9306252632462));
#63668=CARTESIAN_POINT('Ctrl Pts',(4.9241910223198,1.71220928558549,82.8777050091641));
#63669=CARTESIAN_POINT('Ctrl Pts',(4.94951760585997,0.0766427637077434,
82.8247847550821));
#63670=CARTESIAN_POINT('Ctrl Pts',(4.97484418940015,-1.55892375817019,82.7718645010002));
#63671=CARTESIAN_POINT('Ctrl Pts',(4.10928478789245,-3.20828558224624,82.7189442469183));
#63672=CARTESIAN_POINT('Ctrl Pts',(2.74893264004429,-4.11666951392571,82.6660239928363));
#63673=CARTESIAN_POINT('Ctrl Pts',(1.38858049219621,-5.02505344560512,82.6131037387543));
#63674=CARTESIAN_POINT('Ctrl Pts',(-0.466564401992278,-5.19245948488802,
82.5601834846723));
#63675=CARTESIAN_POINT('Ctrl Pts',(-1.96755942526789,-4.5422800890475,82.5072632305904));
#63676=CARTESIAN_POINT('Ctrl Pts',(-3.4685544485435,-3.89210069320699,82.4543429765084));
#63677=CARTESIAN_POINT('Ctrl Pts',(-4.61539960090623,-2.42433586224305,
82.4014227224265));
#63678=CARTESIAN_POINT('Ctrl Pts',(-4.88328101508674,-0.810657190350331,
82.3485024683445));
#63679=CARTESIAN_POINT('Ctrl Pts',(-4.92745864911638,-0.544537549215846,
82.3397751304486));
#63680=CARTESIAN_POINT('Ctrl Pts',(-4.94773117576294,-0.274449500871191,
82.3310477925527));
#63681=CARTESIAN_POINT('Ctrl Pts',(-4.94535283272668,-0.00400458364991862,
82.3223204546568));
#63682=CARTESIAN_POINT('Ctrl Pts',(-4.94609777444767,-0.00376784846301249,
82.1776795453432));
#63683=CARTESIAN_POINT('Ctrl Pts',(-4.94816072809722,-0.247759491874606,
82.1855563085771));
#63684=CARTESIAN_POINT('Ctrl Pts',(-4.93166636384428,-0.49147120021732,
82.193433071811));
#63685=CARTESIAN_POINT('Ctrl Pts',(-4.89565013237716,-0.732262940926013,
82.201309835045));
#63686=CARTESIAN_POINT('Ctrl Pts',(-4.65367407397507,-2.35002898526266,
82.2542300891269));
#63687=CARTESIAN_POINT('Ctrl Pts',(-3.53050790772224,-3.83599172584166,
82.3071503432088));
#63688=CARTESIAN_POINT('Ctrl Pts',(-2.04012962670993,-4.51015191896435,
82.3600705972908));
#63689=CARTESIAN_POINT('Ctrl Pts',(-0.549751345697456,-5.18431211208712,
82.4129908513727));
#63690=CARTESIAN_POINT('Ctrl Pts',(1.3078390500746,-5.04666975775335,82.4659111054547));
#63691=CARTESIAN_POINT('Ctrl Pts',(2.68257982821446,-4.16021209746218,82.5188313595367));
#63692=CARTESIAN_POINT('Ctrl Pts',(4.05732060635432,-3.273754437171,82.5717516136187));
#63693=CARTESIAN_POINT('Ctrl Pts',(4.94921176686199,-1.63848147092241,82.6246718677007));
#63694=CARTESIAN_POINT('Ctrl Pts',(4.95011028710458,-0.00271908696136483,
82.6775921217826));
#63695=CARTESIAN_POINT('Ctrl Pts',(4.95100880734717,1.63304329699958,82.7305123758646));
#63696=CARTESIAN_POINT('Ctrl Pts',(4.06091468732478,3.26929509867298,82.7834326299465));
#63697=CARTESIAN_POINT('Ctrl Pts',(2.68714860199004,4.15726251102139,82.8363528840285));
#63698=CARTESIAN_POINT('Ctrl Pts',(1.31338251665521,5.04522992336985,82.8892731381104));
#63699=CARTESIAN_POINT('Ctrl Pts',(-0.544055533992037,5.18491294639323,
82.9421933921924));
#63700=CARTESIAN_POINT('Ctrl Pts',(-2.0351735518924,4.51239048126625,82.9951136462744));
#63701=CARTESIAN_POINT('Ctrl Pts',(-3.52629156979259,3.83986801613934,83.0480339003563));
#63702=CARTESIAN_POINT('Ctrl Pts',(-4.651089554946,2.35514006286229,83.1009541544383));
#63703=CARTESIAN_POINT('Ctrl Pts',(-4.8948427284911,0.737640835765265,83.1538744085202));
#63704=CARTESIAN_POINT('Ctrl Pts',(-4.9313919209059,0.495107417134616,83.1618094541278));
#63705=CARTESIAN_POINT('Ctrl Pts',(-4.94813254848979,0.249588896780995,
83.1697444997355));
#63706=CARTESIAN_POINT('Ctrl Pts',(-4.94604776483535,0.00378542647206983,
83.1776795453431));
#63707=CARTESIAN_POINT('Origin',(0.,0.,16.));
#63708=CARTESIAN_POINT('',(-4.93450205841395,0.0017791821159216,84.3223204546568));
#63709=CARTESIAN_POINT('',(-4.93425329604086,0.00136738585504144,84.1776795453431));
#63710=CARTESIAN_POINT('',(-4.942,-6.05220448138622E-16,16.));
#63711=CARTESIAN_POINT('Ctrl Pts',(-4.93450205841395,0.0017791821159216,
84.3223204546568));
#63712=CARTESIAN_POINT('Ctrl Pts',(-4.9368080070955,0.715261896051447,84.2994241748696));
#63713=CARTESIAN_POINT('Ctrl Pts',(-4.79225594661696,1.42785481900567,84.2765278950824));
#63714=CARTESIAN_POINT('Ctrl Pts',(-4.49620929648531,2.07068108576527,84.2536316152951));
#63715=CARTESIAN_POINT('Ctrl Pts',(-3.81195560589931,3.55644775544483,84.2007113612132));
#63716=CARTESIAN_POINT('Ctrl Pts',(-2.31839897625278,4.66951227096791,84.1477911071313));
#63717=CARTESIAN_POINT('Ctrl Pts',(-0.699026613519106,4.90050762812279,
84.0948708530493));
#63718=CARTESIAN_POINT('Ctrl Pts',(0.92034574921447,5.13150298527765,84.0419505989674));
#63719=CARTESIAN_POINT('Ctrl Pts',(2.66553384503535,4.48042918406423,83.9890303448854));
#63720=CARTESIAN_POINT('Ctrl Pts',(3.73791967339092,3.24523363926685,83.9361100908034));
#63721=CARTESIAN_POINT('Ctrl Pts',(4.81030550174656,2.01003809446939,83.8831898367214));
#63722=CARTESIAN_POINT('Ctrl Pts',(5.20988906263709,0.190720806087873,83.8302695826395));
#63723=CARTESIAN_POINT('Ctrl Pts',(4.75381130414694,-1.38017403364147,83.7773493285575));
#63724=CARTESIAN_POINT('Ctrl Pts',(4.29773354565674,-2.951068873371,83.7244290744756));
#63725=CARTESIAN_POINT('Ctrl Pts',(2.9859944677857,-4.27354126444818,83.6715088203937));
#63726=CARTESIAN_POINT('Ctrl Pts',(1.41886773993217,-4.74240598011873,83.6185885663117));
#63727=CARTESIAN_POINT('Ctrl Pts',(-0.148258987921171,-5.21127069578923,
83.5656683122296));
#63728=CARTESIAN_POINT('Ctrl Pts',(-1.97077336575683,-4.82652773605328,
83.5127480581476));
#63729=CARTESIAN_POINT('Ctrl Pts',(-3.21466593691877,-3.76424222358033,
83.4598278040656));
#63730=CARTESIAN_POINT('Ctrl Pts',(-4.29203775090064,-2.84416560597453,
83.4139920209293));
#63731=CARTESIAN_POINT('Ctrl Pts',(-4.93533906889132,-1.41581012896607,
83.3681562377931));
#63732=CARTESIAN_POINT('Ctrl Pts',(-4.94676006163664,0.00350952918951444,
83.3223204546568));
#63733=CARTESIAN_POINT('Ctrl Pts',(-4.94604776483535,0.00378542647206983,
83.1776795453431));
#63734=CARTESIAN_POINT('Ctrl Pts',(-4.93422874929891,-1.38971889629444,
83.2226647538174));
#63735=CARTESIAN_POINT('Ctrl Pts',(-4.31736833349613,-2.79238139987207,
83.2676499622918));
#63736=CARTESIAN_POINT('Ctrl Pts',(-3.27460228178232,-3.71222020633235,
83.3126351707661));
#63737=CARTESIAN_POINT('Ctrl Pts',(-2.04790029959144,-4.7943115204161,83.3655554248481));
#63738=CARTESIAN_POINT('Ctrl Pts',(-0.231787973272793,-5.20822364766616,
83.4184756789301));
#63739=CARTESIAN_POINT('Ctrl Pts',(1.34265411435701,-4.76454397765274,83.4713959330121));
#63740=CARTESIAN_POINT('Ctrl Pts',(2.91709620198673,-4.32086430763936,83.524316187094));
#63741=CARTESIAN_POINT('Ctrl Pts',(4.24986805092773,-3.01959284036256,83.577236441176));
#63742=CARTESIAN_POINT('Ctrl Pts',(4.73107261188716,-1.45621146364564,83.630156695258));
#63743=CARTESIAN_POINT('Ctrl Pts',(5.21227717284655,0.107169913071196,83.6830769493399));
#63744=CARTESIAN_POINT('Ctrl Pts',(4.84191444582465,1.93266119922796,83.7359972034218));
#63745=CARTESIAN_POINT('Ctrl Pts',(3.78946863845564,3.18489006691465,83.7889174575038));
#63746=CARTESIAN_POINT('Ctrl Pts',(2.73702283108663,4.43711893460135,83.8418377115857));
#63747=CARTESIAN_POINT('Ctrl Pts',(1.00249394337044,5.11608538381779,83.8947579656677));
#63748=CARTESIAN_POINT('Ctrl Pts',(-0.620372201325573,4.91108329901265,
83.9476782197497));
#63749=CARTESIAN_POINT('Ctrl Pts',(-2.24323834602159,4.70608121420751,84.0005984738317));
#63750=CARTESIAN_POINT('Ctrl Pts',(-3.75444174769753,3.6171105953808,84.0535187279136));
#63751=CARTESIAN_POINT('Ctrl Pts',(-4.4624305684118,2.14250236754745,84.1064389819956));
#63752=CARTESIAN_POINT('Ctrl Pts',(-4.78012570742429,1.48080284317098,84.1301858364447));
#63753=CARTESIAN_POINT('Ctrl Pts',(-4.93608736949663,0.741452199377731,
84.1539326908939));
#63754=CARTESIAN_POINT('Ctrl Pts',(-4.93425329604086,0.00136738585504144,
84.1776795453431));
#63755=CARTESIAN_POINT('Origin',(0.,0.,16.));
#63756=CARTESIAN_POINT('',(-4.93983901057914,-0.00407131671605609,85.3223204546568));
#63757=CARTESIAN_POINT('',(-4.94096920053978,-0.0044629540342261,85.1776795453431));
#63758=CARTESIAN_POINT('',(-4.942,-6.05220448138622E-16,16.));
#63759=CARTESIAN_POINT('Ctrl Pts',(-4.93983901057914,-0.00407131671605609,
85.3223204546568));
#63760=CARTESIAN_POINT('Ctrl Pts',(-4.92935782359351,1.19852489561668,85.283612366028));
#63761=CARTESIAN_POINT('Ctrl Pts',(-4.48753687762877,2.40778661262928,85.2449042773993));
#63762=CARTESIAN_POINT('Ctrl Pts',(-3.69010132050912,3.2995468819145,85.2061961887705));
#63763=CARTESIAN_POINT('Ctrl Pts',(-2.59987718928131,4.51872823916,85.1532759346885));
#63764=CARTESIAN_POINT('Ctrl Pts',(-0.844961773498813,5.14445691330988,
85.1003556806066));
#63765=CARTESIAN_POINT('Ctrl Pts',(0.770932612771407,4.88981272332166,85.0474354265247));
#63766=CARTESIAN_POINT('Ctrl Pts',(2.38682699904172,4.63516853333343,84.9945151724427));
#63767=CARTESIAN_POINT('Ctrl Pts',(3.86370035579973,3.500151479207,84.9415949183607));
#63768=CARTESIAN_POINT('Ctrl Pts',(4.52604489048226,2.00446382425534,84.8886746642787));
#63769=CARTESIAN_POINT('Ctrl Pts',(5.18838942516471,0.508776169303851,84.8357544101967));
#63770=CARTESIAN_POINT('Ctrl Pts',(5.0362051377719,-1.34758208647277,84.7828341561149));
#63771=CARTESIAN_POINT('Ctrl Pts',(4.13896054991356,-2.7152702523835,84.7299139020329));
#63772=CARTESIAN_POINT('Ctrl Pts',(3.24171596205511,-4.08295841829439,84.6769936479509));
#63773=CARTESIAN_POINT('Ctrl Pts',(1.59941107373096,-4.96197649433929,84.6240733938688));
#63774=CARTESIAN_POINT('Ctrl Pts',(-0.0363198163526684,-4.94999030922869,
84.5711531397869));
#63775=CARTESIAN_POINT('Ctrl Pts',(-1.67205070643629,-4.93800412411811,
84.518232885705));
#63776=CARTESIAN_POINT('Ctrl Pts',(-3.30120759827939,-4.03501367785208,
84.4653126316231));
#63777=CARTESIAN_POINT('Ctrl Pts',(-4.17831066843813,-2.65428404280099,
84.4123923775412));
#63778=CARTESIAN_POINT('Ctrl Pts',(-4.67592959505013,-1.87093574279885,
84.3823684032464));
#63779=CARTESIAN_POINT('Ctrl Pts',(-4.93147825958796,-0.9338132749143,84.3523444289516));
#63780=CARTESIAN_POINT('Ctrl Pts',(-4.93450205841395,0.0017791821159216,
84.3223204546568));
#63781=CARTESIAN_POINT('Ctrl Pts',(-4.93425329604086,0.00136738585504144,
84.1776795453431));
#63782=CARTESIAN_POINT('Ctrl Pts',(-4.93200010676076,-0.907838929165127,
84.2068529449759));
#63783=CARTESIAN_POINT('Ctrl Pts',(-4.6915933103023,-1.81815329167953,84.2360263446087));
#63784=CARTESIAN_POINT('Ctrl Pts',(-4.22033403606684,-2.58696080038834,
84.2651997442415));
#63785=CARTESIAN_POINT('Ctrl Pts',(-3.36547444325506,-3.98156990365044,
84.3181199983235));
#63786=CARTESIAN_POINT('Ctrl Pts',(-1.75098101787896,-4.91054227333463,
84.3710402524054));
#63787=CARTESIAN_POINT('Ctrl Pts',(-0.115662974249316,-4.94876105553069,
84.4239605064874));
#63788=CARTESIAN_POINT('Ctrl Pts',(1.51965506938033,-4.98697983772675,84.4768807605693));
#63789=CARTESIAN_POINT('Ctrl Pts',(3.17579773126353,-4.1344450324347,84.5298010146513));
#63790=CARTESIAN_POINT('Ctrl Pts',(4.09487421234139,-2.78129899063739,84.5827212687333));
#63791=CARTESIAN_POINT('Ctrl Pts',(5.01395069341925,-1.42815294884008,84.6356415228152));
#63792=CARTESIAN_POINT('Ctrl Pts',(5.19596099369178,0.425604329462498,84.6885617768972));
#63793=CARTESIAN_POINT('Ctrl Pts',(4.55764242829978,1.93168321282745,84.7414820309791));
#63794=CARTESIAN_POINT('Ctrl Pts',(3.91932386290774,3.43776209619249,84.7944022850611));
#63795=CARTESIAN_POINT('Ctrl Pts',(2.46067643185109,4.59616258461988,84.8473225391431));
#63796=CARTESIAN_POINT('Ctrl Pts',(0.849145831707845,4.87674842560418,84.9002427932251));
#63797=CARTESIAN_POINT('Ctrl Pts',(-0.762384768435213,5.15733426658845,
84.9531630473071));
#63798=CARTESIAN_POINT('Ctrl Pts',(-2.52679853766482,4.5601054601299,85.006083301389));
#63799=CARTESIAN_POINT('Ctrl Pts',(-3.63657003853315,3.35842910333814,85.059003555471));
#63800=CARTESIAN_POINT('Ctrl Pts',(-4.46614045337841,2.46015846561364,85.0985622187617));
#63801=CARTESIAN_POINT('Ctrl Pts',(-4.92991110676884,1.22413577549367,85.1381208820524));
#63802=CARTESIAN_POINT('Ctrl Pts',(-4.94096920053978,-0.0044629540342261,
85.1776795453431));
#63803=CARTESIAN_POINT('Origin',(0.,0.,24.1514101080949));
#63804=CARTESIAN_POINT('',(-4.37008825460381,-0.00360173951420115,85.6514101080948));
#63805=CARTESIAN_POINT('',(-4.37741404908174,0.00054794132368214,85.8485898919049));
#63806=CARTESIAN_POINT('',(-4.372,3.82579154166093E-12,24.1514101080949));
#63807=CARTESIAN_POINT('',(2.54472701347433,-3.56250531650779,85.9999999999999));
#63808=CARTESIAN_POINT('Ctrl Pts',(-4.37008825460381,-0.00360173951420056,
85.6514101080948));
#63809=CARTESIAN_POINT('Ctrl Pts',(-4.37349270028371,-0.394222905349127,
85.665622273548));
#63810=CARTESIAN_POINT('Ctrl Pts',(-4.14658524106498,-2.2356015936124,85.7327546930832));
#63811=CARTESIAN_POINT('Ctrl Pts',(-1.63914477126166,-4.84388062782939,
85.8489513237184));
#63812=CARTESIAN_POINT('Ctrl Pts',(1.44818750565376,-4.33531680853971,85.9509357889001));
#63813=CARTESIAN_POINT('Ctrl Pts',(2.54472701347433,-3.56250531650779,85.9999999999999));
#63814=CARTESIAN_POINT('',(-2.53835875722777,-3.5596515025498,86.));
#63815=CARTESIAN_POINT('Origin',(0.,0.,86.));
#63816=CARTESIAN_POINT('Ctrl Pts',(-4.37741404908174,0.000547941323682409,
85.8485898919049));
#63817=CARTESIAN_POINT('Ctrl Pts',(-4.37702756934774,-0.658293262144059,
85.8725998008956));
#63818=CARTESIAN_POINT('Ctrl Pts',(-4.04502790407186,-2.04740376323306,
85.9230698369273));
#63819=CARTESIAN_POINT('Ctrl Pts',(-3.130164636136,-3.13763950664809,85.973539872959));
#63820=CARTESIAN_POINT('Ctrl Pts',(-2.53835875722777,-3.5596515025498,86.));
#63821=CARTESIAN_POINT('Origin',(0.,0.,24.1514101080949));
#63822=CARTESIAN_POINT('',(-4.3653668553998,0.00157397495328755,84.6514101080948));
#63823=CARTESIAN_POINT('',(-4.37108809080528,-0.00394820619502134,84.8485898919049));
#63824=CARTESIAN_POINT('',(-4.372,3.82579154166093E-12,24.1514101080949));
#63825=CARTESIAN_POINT('Ctrl Pts',(-4.3653668553998,0.00157397495328733,
84.6514101080948));
#63826=CARTESIAN_POINT('Ctrl Pts',(-4.36269181524081,-0.826109194237039,
84.6814340823896));
#63827=CARTESIAN_POINT('Ctrl Pts',(-3.73813921667308,-3.11640593107392,
84.7643783107663));
#63828=CARTESIAN_POINT('Ctrl Pts',(-0.0379465312430282,-5.16730640666113,
84.9002427932251));
#63829=CARTESIAN_POINT('Ctrl Pts',(4.32070804489202,-2.83440452778566,85.059003555471));
#63830=CARTESIAN_POINT('Ctrl Pts',(4.72460304963626,2.09234474027741,85.2177643177169));
#63831=CARTESIAN_POINT('Ctrl Pts',(0.805001482004623,5.10466438453535,85.3765250799626));
#63832=CARTESIAN_POINT('Ctrl Pts',(-3.43558144629758,3.5926517202867,85.5210736767555));
#63833=CARTESIAN_POINT('Ctrl Pts',(-4.3608159459227,1.06028952724385,85.6127020194661));
#63834=CARTESIAN_POINT('Ctrl Pts',(-4.37008825460381,-0.00360173951420056,
85.6514101080948));
#63835=CARTESIAN_POINT('Ctrl Pts',(-4.37108809080528,-0.00394820619502242,
84.8485898919049));
#63836=CARTESIAN_POINT('Ctrl Pts',(-4.37439235100703,-0.371064815037356,
84.8619514826962));
#63837=CARTESIAN_POINT('Ctrl Pts',(-4.16412636077677,-2.18847582560682,
84.9282333275694));
#63838=CARTESIAN_POINT('Ctrl Pts',(-1.63279460579437,-4.90302030367583,
85.0474354265246));
#63839=CARTESIAN_POINT('Ctrl Pts',(3.23428855022947,-4.03017982392474,85.2061961887705));
#63840=CARTESIAN_POINT('Ctrl Pts',(5.13873193725801,0.529582954402255,85.3649569510164));
#63841=CARTESIAN_POINT('Ctrl Pts',(2.34489518331184,4.6077777382683,85.5237177132623));
#63842=CARTESIAN_POINT('Ctrl Pts',(-2.60449736313211,4.46265913321349,85.6824784755082));
#63843=CARTESIAN_POINT('Ctrl Pts',(-4.34126539015093,1.58670061603872,85.7907692017224));
#63844=CARTESIAN_POINT('Ctrl Pts',(-4.37745348944865,0.0677828737684449,
85.8461396738546));
#63845=CARTESIAN_POINT('Ctrl Pts',(-4.37741404908174,0.000547941323682409,
85.8485898919049));
#63846=CARTESIAN_POINT('Origin',(0.,0.,24.1514101080949));
#63847=CARTESIAN_POINT('',(-4.37621104602901,0.00310474739351271,83.6514101080948));
#63848=CARTESIAN_POINT('',(-4.36514678476137,0.00120967441979231,83.8485898919049));
#63849=CARTESIAN_POINT('',(-4.372,3.82579154166093E-12,24.1514101080949));
#63850=CARTESIAN_POINT('Ctrl Pts',(-4.37621104602901,0.00310474739351276,
83.6514101080948));
#63851=CARTESIAN_POINT('Ctrl Pts',(-4.36610732682993,-1.25251353375917,
83.6972458912311));
#63852=CARTESIAN_POINT('Ctrl Pts',(-3.13993685867563,-3.97504379283746,
83.7960019284495));
#63853=CARTESIAN_POINT('Ctrl Pts',(1.4811502559097,-4.9505810809301,83.9476782197498));
#63854=CARTESIAN_POINT('Ctrl Pts',(4.96248771955931,-1.44075755171813,84.1064389819956));
#63855=CARTESIAN_POINT('Ctrl Pts',(3.90199844707087,3.38768549854763,84.2651997442416));
#63856=CARTESIAN_POINT('Ctrl Pts',(-0.729706746127024,5.11562640844579,
84.4239605064874));
#63857=CARTESIAN_POINT('Ctrl Pts',(-3.94395824097378,2.72022390956171,84.5526972944385));
#63858=CARTESIAN_POINT('Ctrl Pts',(-4.36740684075686,0.63276507679951,84.6285138283076));
#63859=CARTESIAN_POINT('Ctrl Pts',(-4.3653668553998,0.00157397495328733,
84.6514101080948));
#63860=CARTESIAN_POINT('Ctrl Pts',(-4.36514678476137,0.00120967441979238,
83.8485898919049));
#63861=CARTESIAN_POINT('Ctrl Pts',(-4.36315347364677,-0.803130675494322,
83.8777632915377));
#63862=CARTESIAN_POINT('Ctrl Pts',(-3.76467753114223,-3.06929475283447,
83.9598569452526));
#63863=CARTESIAN_POINT('Ctrl Pts',(-0.120745397495975,-5.1659971710397,
84.0948708530492));
#63864=CARTESIAN_POINT('Ctrl Pts',(4.27463443926266,-2.90338152834273,84.2536316152952));
#63865=CARTESIAN_POINT('Ctrl Pts',(4.75768727179541,2.01646478129229,84.412392377541));
#63866=CARTESIAN_POINT('Ctrl Pts',(0.886457060193665,5.09084373843816,84.571153139787));
#63867=CARTESIAN_POINT('Ctrl Pts',(-3.40216585276062,3.63920626636618,84.7165523112416));
#63868=CARTESIAN_POINT('Ctrl Pts',(-4.36130541456655,1.08294650151228,84.8090312286142));
#63869=CARTESIAN_POINT('Ctrl Pts',(-4.37108809080528,-0.00394820619502242,
84.8485898919049));
#63870=CARTESIAN_POINT('Origin',(0.,0.,24.1514101080949));
#63871=CARTESIAN_POINT('',(-4.37496612397431,-0.00354270330085218,82.6514101080948));
#63872=CARTESIAN_POINT('',(-4.37558090405915,0.00334882326136696,82.8485898919049));
#63873=CARTESIAN_POINT('',(-4.372,3.82579154166093E-12,24.1514101080949));
#63874=CARTESIAN_POINT('Ctrl Pts',(-4.37496612397431,-0.00354270330085171,
82.6514101080948));
#63875=CARTESIAN_POINT('Ctrl Pts',(-4.37707015387208,-0.242795066330439,
82.6601374459907));
#63876=CARTESIAN_POINT('Ctrl Pts',(-4.25038678075279,-1.93057999813071,
82.7217850379685));
#63877=CARTESIAN_POINT('Ctrl Pts',(-2.05392817541576,-4.74166978382725,
82.8363528840287));
#63878=CARTESIAN_POINT('Ctrl Pts',(2.86960084768762,-4.29737645901297,82.9951136462743));
#63879=CARTESIAN_POINT('Ctrl Pts',(5.16678358952832,0.0800071275065655,
83.1538744085204));
#63880=CARTESIAN_POINT('Ctrl Pts',(2.73516803922529,4.38416562959496,83.312635170766));
#63881=CARTESIAN_POINT('Ctrl Pts',(-2.19975659925683,4.67580205641259,83.4713959330121));
#63882=CARTESIAN_POINT('Ctrl Pts',(-4.27789107195956,1.83931825768632,83.5843209121216));
#63883=CARTESIAN_POINT('Ctrl Pts',(-4.37777269721528,0.197175637492073,
83.6443256371492));
#63884=CARTESIAN_POINT('Ctrl Pts',(-4.37621104602901,0.00310474739351276,
83.6514101080948));
#63885=CARTESIAN_POINT('Ctrl Pts',(-4.37558090405915,0.0033488232613671,
82.8485898919049));
#63886=CARTESIAN_POINT('Ctrl Pts',(-4.36512506919086,-1.22943160958811,
82.8935751003793));
#63887=CARTESIAN_POINT('Ctrl Pts',(-3.17743944272853,-3.93007838737006,
82.9914805629356));
#63888=CARTESIAN_POINT('Ctrl Pts',(1.40159167776471,-4.9736903294079,83.142306279574));
#63889=CARTESIAN_POINT('Ctrl Pts',(4.93874982643145,-1.52013376024582,83.3010670418199));
#63890=CARTESIAN_POINT('Ctrl Pts',(3.95581224496304,3.32469499516411,83.4598278040656));
#63891=CARTESIAN_POINT('Ctrl Pts',(-0.647603556591826,5.12666260907039,
83.6185885663118));
#63892=CARTESIAN_POINT('Ctrl Pts',(-3.92132004033239,2.76762804019117,83.7481759289246));
#63893=CARTESIAN_POINT('Ctrl Pts',(-4.36676931999915,0.655934645021535,
83.8248430374557));
#63894=CARTESIAN_POINT('Ctrl Pts',(-4.36514678476137,0.00120967441979238,
83.8485898919049));
#63895=CARTESIAN_POINT('Origin',(0.,0.,24.1514101080949));
#63896=CARTESIAN_POINT('',(-4.36499281949393,-0.000862724152283187,81.6514101080949));
#63897=CARTESIAN_POINT('',(-4.37562514566675,-0.00333327265474082,81.8485898919049));
#63898=CARTESIAN_POINT('',(-4.372,3.82579154166093E-12,24.1514101080949));
#63899=CARTESIAN_POINT('Ctrl Pts',(-4.36499281949393,-0.000862724152282945,
81.6514101080949));
#63900=CARTESIAN_POINT('Ctrl Pts',(-4.36618629939077,-0.677492060307118,
81.6759492548323));
#63901=CARTESIAN_POINT('Ctrl Pts',(-3.8997785113075,-2.81175799367349,81.7534086556517));
#63902=CARTESIAN_POINT('Ctrl Pts',(-0.57097184883837,-5.13576134197884,
81.8837883105532));
#63903=CARTESIAN_POINT('Ctrl Pts',(4.00502195951943,-3.26524922770216,82.0425490727989));
#63904=CARTESIAN_POINT('Ctrl Pts',(4.91549733690694,1.59371871934676,82.2013098350451));
#63905=CARTESIAN_POINT('Ctrl Pts',(1.32715940311121,4.99406661129702,82.3600705972907));
#63906=CARTESIAN_POINT('Ctrl Pts',(-3.21180689907642,3.88802958864094,82.510104021641));
#63907=CARTESIAN_POINT('Ctrl Pts',(-4.36431187659278,1.20796758228371,82.6072171919088));
#63908=CARTESIAN_POINT('Ctrl Pts',(-4.37496612397431,-0.00354270330085171,
82.6514101080948));
#63909=CARTESIAN_POINT('Ctrl Pts',(-4.37562514566675,-0.00333327265474043,
81.8485898919049));
#63910=CARTESIAN_POINT('Ctrl Pts',(-4.37745016253379,-0.219183427450699,
81.8564666551388));
#63911=CARTESIAN_POINT('Ctrl Pts',(-4.26482187642182,-1.88331740650866,
81.9172636724547));
#63912=CARTESIAN_POINT('Ctrl Pts',(-2.12968395259116,-4.7081313086182,82.0309809438528));
#63913=CARTESIAN_POINT('Ctrl Pts',(2.80033539806548,-4.3428303941221,82.1897417060986));
#63914=CARTESIAN_POINT('Ctrl Pts',(5.16740226597732,-0.00283844241944707,
82.3485024683445));
#63915=CARTESIAN_POINT('Ctrl Pts',(2.80510471878759,4.33975132503298,82.5072632305904));
#63916=CARTESIAN_POINT('Ctrl Pts',(-2.12451031000386,4.71046814615349,82.6660239928362));
#63917=CARTESIAN_POINT('Ctrl Pts',(-4.26384621089875,1.88655500314254,82.7797995466078));
#63918=CARTESIAN_POINT('Ctrl Pts',(-4.37742523310327,0.220801832606586,
82.8406548462974));
#63919=CARTESIAN_POINT('Ctrl Pts',(-4.37558090405915,0.0033488232613671,
82.8485898919049));
#63920=CARTESIAN_POINT('Origin',(0.,0.,24.1514101080949));
#63921=CARTESIAN_POINT('',(-4.37180197783241,0.00399615447510604,80.6514101080948));
#63922=CARTESIAN_POINT('',(-4.3651608225263,-0.00123442373144794,80.8485898919049));
#63923=CARTESIAN_POINT('',(-4.372,3.82579154166093E-12,24.1514101080949));
#63924=CARTESIAN_POINT('Ctrl Pts',(-4.37180197783241,0.00399615447510625,
80.6514101080948));
#63925=CARTESIAN_POINT('Ctrl Pts',(-4.36165896025063,-1.10425130818043,
80.6917610636739));
#63926=CARTESIAN_POINT('Ctrl Pts',(-3.37083349090091,-3.68210362881494,
80.7850322733349));
#63927=CARTESIAN_POINT('Ctrl Pts',(0.962330231331446,-5.07700442602626,
80.9312237370778));
#63928=CARTESIAN_POINT('Ctrl Pts',(4.78729812901886,-1.94520694012218,81.0899844993237));
#63929=CARTESIAN_POINT('Ctrl Pts',(4.2307845491307,2.96690335452649,81.2487452615696));
#63930=CARTESIAN_POINT('Ctrl Pts',(-0.19787228117179,5.16361307382143,81.4075060238155));
#63931=CARTESIAN_POINT('Ctrl Pts',(-3.78889879581372,3.02535473653369,81.541727639324));
#63932=CARTESIAN_POINT('Ctrl Pts',(-4.36361248294727,0.781702783413628,
81.6230290007504));
#63933=CARTESIAN_POINT('Ctrl Pts',(-4.36499281949393,-0.000862724152282945,
81.6514101080949));
#63934=CARTESIAN_POINT('Ctrl Pts',(-4.3651608225263,-0.00123442373144732,
80.8485898919049));
#63935=CARTESIAN_POINT('Ctrl Pts',(-4.36681289312482,-0.654347754103861,
80.8722784639804));
#63936=CARTESIAN_POINT('Ctrl Pts',(-3.92288549979199,-2.76438197736347,
80.9488872901379));
#63937=CARTESIAN_POINT('Ctrl Pts',(-0.653236375128765,-5.12594736724498,
81.0784163703773));
#63938=CARTESIAN_POINT('Ctrl Pts',(3.95215792026738,-3.32903919274863,81.2371771326234));
#63939=CARTESIAN_POINT('Ctrl Pts',(4.94041656702063,1.51470733791976,81.3959378948691));
#63940=CARTESIAN_POINT('Ctrl Pts',(1.40705506422376,4.97214744531344,81.5546986571151));
#63941=CARTESIAN_POINT('Ctrl Pts',(-3.17488990257063,3.9331654538798,81.7055826561271));
#63942=CARTESIAN_POINT('Ctrl Pts',(-4.36518873567112,1.23101187436481,81.8035464010569));
#63943=CARTESIAN_POINT('Ctrl Pts',(-4.37562514566675,-0.00333327265474043,
81.8485898919049));
#63944=CARTESIAN_POINT('Origin',(0.,0.,24.1514101080949));
#63945=CARTESIAN_POINT('',(-4.37845870912757,-0.00160159003492085,79.6514101080949));
#63946=CARTESIAN_POINT('',(-4.37110144318797,0.00398541688994905,79.8485898919049));
#63947=CARTESIAN_POINT('',(-4.372,3.82579154166093E-12,24.1514101080949));
#63948=CARTESIAN_POINT('Ctrl Pts',(-4.37845870912757,-0.00160159003492056,
79.6514101080949));
#63949=CARTESIAN_POINT('Ctrl Pts',(-4.37887661134401,-0.0903064267712891,
79.6546526184335));
#63950=CARTESIAN_POINT('Ctrl Pts',(-4.3362288360819,-1.62633270599671,79.7108153828541));
#63951=CARTESIAN_POINT('Ctrl Pts',(-2.53231305975701,-4.50438053270811,
79.8198984013567));
#63952=CARTESIAN_POINT('Ctrl Pts',(2.41077833593552,-4.57057996659486,79.9786591636024));
#63953=CARTESIAN_POINT('Ctrl Pts',(5.14745176039643,-0.453645004871452,
80.1374199258484));
#63954=CARTESIAN_POINT('Ctrl Pts',(3.1730201027819,4.07847972207792,80.2961806880942));
#63955=CARTESIAN_POINT('Ctrl Pts',(-1.70545647406065,4.87785522859546,80.4549414503402));
#63956=CARTESIAN_POINT('Ctrl Pts',(-4.17984164299754,2.14436901967187,80.573351257007));
#63957=CARTESIAN_POINT('Ctrl Pts',(-4.37496152173606,0.349214575534816,
80.6388408095919));
#63958=CARTESIAN_POINT('Ctrl Pts',(-4.37180197783241,0.00399615447510625,
80.6514101080948));
#63959=CARTESIAN_POINT('Ctrl Pts',(-4.37110144318797,0.00398541688994905,
79.8485898919049));
#63960=CARTESIAN_POINT('Ctrl Pts',(-4.36133704968111,-1.0813445883965,79.888090272822));
#63961=CARTESIAN_POINT('Ctrl Pts',(-3.40435481309659,-3.63610732924809,
79.980510907821));
#63962=CARTESIAN_POINT('Ctrl Pts',(0.880810665839244,-5.09178031191025,
80.125851796902));
#63963=CARTESIAN_POINT('Ctrl Pts',(4.75549683016874,-2.02170820645871,80.2846125591479));
#63964=CARTESIAN_POINT('Ctrl Pts',(4.27780703699033,2.89869300342805,80.4433733213939));
#63965=CARTESIAN_POINT('Ctrl Pts',(-0.11506242376767,5.16612183484124,80.6021340836397));
#63966=CARTESIAN_POINT('Ctrl Pts',(-3.76287956508864,3.07252682993506,80.7372062738101));
#63967=CARTESIAN_POINT('Ctrl Pts',(-4.36312216851904,0.804706986612936,
80.8193582098985));
#63968=CARTESIAN_POINT('Ctrl Pts',(-4.3651608225263,-0.00123442373144732,
80.8485898919049));
#63969=CARTESIAN_POINT('Origin',(0.,0.,24.1514101080949));
#63970=CARTESIAN_POINT('',(-4.36706479197461,-0.00298086264687759,78.6514101080949));
#63971=CARTESIAN_POINT('',(-4.37877376767475,-0.00119946029119966,78.8485898919049));
#63972=CARTESIAN_POINT('',(-4.372,3.82579154166093E-12,24.1514101080949));
#63973=CARTESIAN_POINT('Ctrl Pts',(-4.36706479197461,-0.00298086264687698,
78.6514101080949));
#63974=CARTESIAN_POINT('Ctrl Pts',(-4.37035845585727,-0.527750657057906,
78.670464427275));
#63975=CARTESIAN_POINT('Ctrl Pts',(-4.03993636744864,-2.50597397148776,
78.7424390005372));
#63976=CARTESIAN_POINT('Ctrl Pts',(-1.0979463908737,-5.04941255383462,78.8673338278812));
#63977=CARTESIAN_POINT('Ctrl Pts',(3.64665478912629,-3.66114220769932,79.0260945901272));
#63978=CARTESIAN_POINT('Ctrl Pts',(5.05372611759689,1.07791731796727,79.184855352373));
#63979=CARTESIAN_POINT('Ctrl Pts',(1.83547293516864,4.83043398881696,79.3436161146189));
#63980=CARTESIAN_POINT('Ctrl Pts',(-2.96262225304742,4.17564214514766,79.4991343665262));
#63981=CARTESIAN_POINT('Ctrl Pts',(-4.37205612685341,1.35742450024673,79.6017323643515));
#63982=CARTESIAN_POINT('Ctrl Pts',(-4.37845870912757,-0.00160159003492056,
79.6514101080949));
#63983=CARTESIAN_POINT('Ctrl Pts',(-4.37877376767475,-0.00119946029119964,
78.8485898919049));
#63984=CARTESIAN_POINT('Ctrl Pts',(-4.37901256877795,-0.0666227183370213,
78.8509818275816));
#63985=CARTESIAN_POINT('Ctrl Pts',(-4.34804095188971,-1.57926832145057,
78.9062940173403));
#63986=CARTESIAN_POINT('Ctrl Pts',(-2.60420306585193,-4.46320294918618,
79.0145264611808));
#63987=CARTESIAN_POINT('Ctrl Pts',(2.33719176176521,-4.60864284172174,79.1732872234268));
#63988=CARTESIAN_POINT('Ctrl Pts',(5.13951729856278,-0.536112032685121,
79.3320479856725));
#63989=CARTESIAN_POINT('Ctrl Pts',(3.23799961511593,4.02708488442023,79.4908087479186));
#63990=CARTESIAN_POINT('Ctrl Pts',(-1.62703422207133,4.90457070639472,79.6495695101643));
#63991=CARTESIAN_POINT('Ctrl Pts',(-4.16301218854004,2.19175778571074,79.7688298914932));
#63992=CARTESIAN_POINT('Ctrl Pts',(-4.37441880163748,0.372715810744746,
79.83517001874));
#63993=CARTESIAN_POINT('Ctrl Pts',(-4.37110144318797,0.00398541688994905,
79.8485898919049));
#63994=CARTESIAN_POINT('Origin',(0.,0.,24.1514101080949));
#63995=CARTESIAN_POINT('',(-4.36767022761989,0.00326609935392151,77.6514101080949));
#63996=CARTESIAN_POINT('',(-4.36757594524889,-0.00322601897944697,77.8485898919049));
#63997=CARTESIAN_POINT('',(-4.372,3.82579154166093E-12,24.1514101080949));
#63998=CARTESIAN_POINT('Ctrl Pts',(-4.36767022761989,0.00326609935392137,
77.6514101080949));
#63999=CARTESIAN_POINT('Ctrl Pts',(-4.36100748821687,-0.956637771051708,
77.6862762361166));
#64000=CARTESIAN_POINT('Ctrl Pts',(-3.57653367776381,-3.38339660944801,
77.7740626182202));
#64001=CARTESIAN_POINT('Ctrl Pts',(0.433232280173729,-5.14920995954434,
77.9147692544059));
#64002=CARTESIAN_POINT('Ctrl Pts',(4.56098553273524,-2.42888130344712,78.0735300166518));
#64003=CARTESIAN_POINT('Ctrl Pts',(4.51438550862023,2.51443371271033,78.2322907788977));
#64004=CARTESIAN_POINT('Ctrl Pts',(0.336081973315249,5.15646219061744,78.3910515411436));
#64005=CARTESIAN_POINT('Ctrl Pts',(-3.61142097688492,3.32845736892325,78.5307579842093));
#64006=CARTESIAN_POINT('Ctrl Pts',(-4.36121084329327,0.929711590329863,
78.6175441731931));
#64007=CARTESIAN_POINT('Ctrl Pts',(-4.36706479197461,-0.00298086264687698,
78.6514101080949));
#64008=CARTESIAN_POINT('Ctrl Pts',(-4.36757594524889,-0.00322601897944683,
77.8485898919049));
#64009=CARTESIAN_POINT('Ctrl Pts',(-4.37100704730013,-0.504422908173594,
77.8667936364231));
#64010=CARTESIAN_POINT('Ctrl Pts',(-4.05983800326864,-2.45852322858237,
77.9379176350233));
#64011=CARTESIAN_POINT('Ctrl Pts',(-1.17875882811733,-5.03116107861318,
78.0619618877055));
#64012=CARTESIAN_POINT('Ctrl Pts',(3.58748974126774,-3.71913585798031,78.2207226499514));
#64013=CARTESIAN_POINT('Ctrl Pts',(5.07035811814355,0.996756102360001,78.3794834121972));
#64014=CARTESIAN_POINT('Ctrl Pts',(1.91267986918918,4.80038643150889,78.5382441744432));
#64015=CARTESIAN_POINT('Ctrl Pts',(-2.92159273453857,4.2194430180671,78.6946130010123));
#64016=CARTESIAN_POINT('Ctrl Pts',(-4.37372922642899,1.38083068620526,78.7980615734996));
#64017=CARTESIAN_POINT('Ctrl Pts',(-4.37877376767475,-0.00119946029119964,
78.8485898919049));
#64018=CARTESIAN_POINT('Origin',(0.,0.,24.1514101080949));
#64019=CARTESIAN_POINT('',(-4.37882057798781,0.00112692768741051,76.6514101080949));
#64020=CARTESIAN_POINT('',(-4.36715155140556,0.00302605917446269,76.8485898919049));
#64021=CARTESIAN_POINT('',(-4.372,3.82579154166093E-12,24.1514101080949));
#64022=CARTESIAN_POINT('Ctrl Pts',(-4.37882057798781,0.00112692768741048,
76.6514101080949));
#64023=CARTESIAN_POINT('Ctrl Pts',(-4.37403747425012,-1.38495585300809,
76.7020880449581));
#64024=CARTESIAN_POINT('Ctrl Pts',(-2.91430837048911,-4.22712294708155,
76.8056862359034));
#64025=CARTESIAN_POINT('Ctrl Pts',(1.92621046639379,-4.79497306094723,76.9622046809306));
#64026=CARTESIAN_POINT('Ctrl Pts',(5.07314897115,-0.982452509068445,77.1209654431764));
#64027=CARTESIAN_POINT('Ctrl Pts',(3.5769865761566,3.7292385885125,77.2797262054224));
#64028=CARTESIAN_POINT('Ctrl Pts',(-1.19294319381297,5.02781661881079,77.4384869676682));
#64029=CARTESIAN_POINT('Ctrl Pts',(-4.06328911396928,2.45017653498889,77.5623816018925));
#64030=CARTESIAN_POINT('Ctrl Pts',(-4.37112027911439,0.500316573992826,
77.6333559820347));
#64031=CARTESIAN_POINT('Ctrl Pts',(-4.36767022761989,0.00326609935392137,
77.6514101080949));
#64032=CARTESIAN_POINT('Ctrl Pts',(-4.36715155140556,0.00302605917446276,
76.8485898919049));
#64033=CARTESIAN_POINT('Ctrl Pts',(-4.36117507900865,-0.933740289083742,
76.8826054452647));
#64034=CARTESIAN_POINT('Ctrl Pts',(-3.60625270295825,-3.33668347601213,
76.9695412527065));
#64035=CARTESIAN_POINT('Ctrl Pts',(0.350623091062388,-5.15549392607834,
77.1093973142301));
#64036=CARTESIAN_POINT('Ctrl Pts',(4.52145892049186,-2.50169210817825,77.268158076476));
#64037=CARTESIAN_POINT('Ctrl Pts',(4.55411743612604,2.44173474230699,77.4269188387219));
#64038=CARTESIAN_POINT('Ctrl Pts',(0.4187085668894,5.15041137287398,77.5856796009678));
#64039=CARTESIAN_POINT('Ctrl Pts',(-3.58180307113106,3.37518619718569,77.7262366186955));
#64040=CARTESIAN_POINT('Ctrl Pts',(-4.36103246255736,0.952610654051967,
77.8138733823412));
#64041=CARTESIAN_POINT('Ctrl Pts',(-4.36757594524889,-0.00322601897944683,
77.8485898919049));
#64042=CARTESIAN_POINT('Origin',(0.,0.,24.1514101080949));
#64043=CARTESIAN_POINT('',(-4.37097940507052,-0.00397941814148454,75.6514101080949));
#64044=CARTESIAN_POINT('',(-4.37851995085447,0.0015322273023494,75.8485898919049));
#64045=CARTESIAN_POINT('',(-4.372,3.82579154166093E-12,24.1514101080949));
#64046=CARTESIAN_POINT('Ctrl Pts',(-4.37097940507052,-0.00397941814148494,
75.6514101080949));
#64047=CARTESIAN_POINT('Ctrl Pts',(-4.3743208173595,-0.376847295339705,
75.6649795997177));
#64048=CARTESIAN_POINT('Ctrl Pts',(-4.16000539985281,-2.20009534110889,
75.7314693454226));
#64049=CARTESIAN_POINT('Ctrl Pts',(-1.61319567320764,-4.90913975519121,
75.8508793452094));
#64050=CARTESIAN_POINT('Ctrl Pts',(3.24934402869518,-4.01793688343129,76.0096401074552));
#64051=CARTESIAN_POINT('Ctrl Pts',(5.13798482303055,0.550604553524979,76.1684008697012));
#64052=CARTESIAN_POINT('Ctrl Pts',(2.32418496553848,4.61521588466023,76.3271616319469));
#64053=CARTESIAN_POINT('Ctrl Pts',(-2.61677996556865,4.45584066454958,76.485922394193));
#64054=CARTESIAN_POINT('Ctrl Pts',(-4.35007811558771,1.57099298812344,76.5940052195755));
#64055=CARTESIAN_POINT('Ctrl Pts',(-4.37903221319898,0.0624561269022633,
76.6491677908762));
#64056=CARTESIAN_POINT('Ctrl Pts',(-4.37882057798781,0.00112692768741048,
76.6514101080949));
#64057=CARTESIAN_POINT('Ctrl Pts',(-4.37851995085447,0.00153222730234961,
75.8485898919049));
#64058=CARTESIAN_POINT('Ctrl Pts',(-4.37234073616906,-1.36153629732671,
75.8984172541062));
#64059=CARTESIAN_POINT('Ctrl Pts',(-2.9554520406374,-4.18336396709743,76.0011648703895));
#64060=CARTESIAN_POINT('Ctrl Pts',(1.84908863423975,-4.82523837717284,76.1568327407549));
#64061=CARTESIAN_POINT('Ctrl Pts',(5.05674607440601,-1.06366033713594,76.3155935030006));
#64062=CARTESIAN_POINT('Ctrl Pts',(3.63631504695578,3.6714121333759,76.4743542652466));
#64063=CARTESIAN_POINT('Ctrl Pts',(-1.11218258415778,5.04629607467818,76.6331150274925));
#64064=CARTESIAN_POINT('Ctrl Pts',(-4.04347203458464,2.49762731386996,76.7578602363785));
#64065=CARTESIAN_POINT('Ctrl Pts',(-4.37047307379395,0.523649295054832,
76.8296851911827));
#64066=CARTESIAN_POINT('Ctrl Pts',(-4.36715155140556,0.00302605917446276,
76.8485898919049));
#64067=CARTESIAN_POINT('Origin',(0.,0.,24.1514101080949));
#64068=CARTESIAN_POINT('',(-4.36519646031047,0.00129875109319553,74.6514101080949));
#64069=CARTESIAN_POINT('',(-4.37167806635839,-0.00399716320838295,74.8485898919049));
#64070=CARTESIAN_POINT('',(-4.372,3.82579154166093E-12,24.1514101080949));
#64071=CARTESIAN_POINT('Ctrl Pts',(-4.36519646031047,0.00129875109319548,
74.6514101080949));
#64072=CARTESIAN_POINT('Ctrl Pts',(-4.36303959174397,-0.808751209913892,
74.6807914085593));
#64073=CARTESIAN_POINT('Ctrl Pts',(-3.75824647517972,-3.08081912741743,
74.7630929631056));
#64074=CARTESIAN_POINT('Ctrl Pts',(-0.100492272925181,-5.16642571988962,
74.898314771734));
#64075=CARTESIAN_POINT('Ctrl Pts',(4.28596496729055,-2.88661700182285,75.0570755339799));
#64076=CARTESIAN_POINT('Ctrl Pts',(4.74977615293751,2.03511176917654,75.2158362962258));
#64077=CARTESIAN_POINT('Ctrl Pts',(0.866447119614458,5.09424408572719,75.3745970584717));
#64078=CARTESIAN_POINT('Ctrl Pts',(-3.41018887347201,3.62800267766814,75.5197883290947));
#64079=CARTESIAN_POINT('Ctrl Pts',(-4.36128949737787,1.07731645292395,75.6120593456358));
#64080=CARTESIAN_POINT('Ctrl Pts',(-4.37097940507052,-0.00397941814148494,
75.6514101080949));
#64081=CARTESIAN_POINT('Ctrl Pts',(-4.37167806635839,-0.00399716320838302,
74.8485898919049));
#64082=CARTESIAN_POINT('Ctrl Pts',(-4.37486787390589,-0.3533501983587,74.8613088088659));
#64083=CARTESIAN_POINT('Ctrl Pts',(-4.1769137234544,-2.15270356402942,74.9269479799088));
#64084=CARTESIAN_POINT('Ctrl Pts',(-1.69169300421356,-4.88264569196979,
75.0455074050335));
#64085=CARTESIAN_POINT('Ctrl Pts',(3.18450981172911,-4.06951488912588,75.2042681672795));
#64086=CARTESIAN_POINT('Ctrl Pts',(5.14615197585861,0.468160245196775,75.3630289295254));
#64087=CARTESIAN_POINT('Ctrl Pts',(2.39787866042351,4.57736082297456,75.5217896917712));
#64088=CARTESIAN_POINT('Ctrl Pts',(-2.54500644918866,4.49722095825909,75.6805504540172));
#64089=CARTESIAN_POINT('Ctrl Pts',(-4.33833518668749,1.61805156266242,75.7894838540617));
#64090=CARTESIAN_POINT('Ctrl Pts',(-4.37890350804243,0.0861408316175627,
75.8454970000243));
#64091=CARTESIAN_POINT('Ctrl Pts',(-4.37851995085447,0.00153222730234961,
75.8485898919049));
#64092=CARTESIAN_POINT('Origin',(0.,0.,24.1514101080949));
#64093=CARTESIAN_POINT('',(-4.37573799308197,0.00329254665532695,73.6514101080949));
#64094=CARTESIAN_POINT('',(-4.36501807785945,0.000928765700389245,73.8485898919049));
#64095=CARTESIAN_POINT('',(-4.372,3.82579154166093E-12,24.1514101080949));
#64096=CARTESIAN_POINT('Ctrl Pts',(-4.37573799308197,0.00329254665532727,
73.6514101080949));
#64097=CARTESIAN_POINT('Ctrl Pts',(-4.36535453025917,-1.23506946531353,
73.6966032174009));
#64098=CARTESIAN_POINT('Ctrl Pts',(-3.16833117156948,-3.94108625070045,
73.7947165807888));
#64099=CARTESIAN_POINT('Ctrl Pts',(1.42107208653042,-4.9681593715318,73.9457501982587));
#64100=CARTESIAN_POINT('Ctrl Pts',(4.94466868411869,-1.50076814343543,74.1045109605046));
#64101=CARTESIAN_POINT('Ctrl Pts',(3.94275346512999,3.34017193109278,74.2632717227505));
#64102=CARTESIAN_POINT('Ctrl Pts',(-0.667690158118302,5.12408462740484,
74.4220324849963));
#64103=CARTESIAN_POINT('Ctrl Pts',(-3.9268970087966,2.75604594892831,74.5514119467779));
#64104=CARTESIAN_POINT('Ctrl Pts',(-4.3669244447204,0.650273716756605,74.6278711544774));
#64105=CARTESIAN_POINT('Ctrl Pts',(-4.36519646031047,0.00129875109319548,
74.6514101080949));
#64106=CARTESIAN_POINT('Ctrl Pts',(-4.36501807785945,0.000928765700389245,
73.8485898919049));
#64107=CARTESIAN_POINT('Ctrl Pts',(-4.36352375843653,-0.785750920308218,
73.8771206177074));
#64108=CARTESIAN_POINT('Ctrl Pts',(-3.78436122884701,-3.0336560998423,73.9585715975918));
#64109=CARTESIAN_POINT('Ctrl Pts',(-0.183308880309829,-5.16415065893858,
74.0929428315583));
#64110=CARTESIAN_POINT('Ctrl Pts',(4.23913515679244,-2.95495977912772,74.2517035938041));
#64111=CARTESIAN_POINT('Ctrl Pts',(4.78179321232898,1.95870055096247,74.4104643560501));
#64112=CARTESIAN_POINT('Ctrl Pts',(0.948008058166557,5.07969830752458,74.5692251182959));
#64113=CARTESIAN_POINT('Ctrl Pts',(-3.37677384390662,3.67402258696438,74.7152669635808));
#64114=CARTESIAN_POINT('Ctrl Pts',(-4.36159587705234,1.10022100123729,74.8083885547839));
#64115=CARTESIAN_POINT('Ctrl Pts',(-4.37167806635839,-0.00399716320838302,
74.8485898919049));
#64116=CARTESIAN_POINT('Origin',(0.,0.,24.1514101080949));
#64117=CARTESIAN_POINT('',(-4.37546659946853,-0.00338795269852561,72.6514101080949));
#64118=CARTESIAN_POINT('',(-4.37508401727703,0.00350862331529297,72.848589891905));
#64119=CARTESIAN_POINT('',(-4.372,3.82579154166093E-12,24.1514101080949));
#64120=CARTESIAN_POINT('Ctrl Pts',(-4.37546659946853,-0.00338795269852542,
72.6514101080949));
#64121=CARTESIAN_POINT('Ctrl Pts',(-4.37736040129649,-0.224956166423907,
72.6594947721605));
#64122=CARTESIAN_POINT('Ctrl Pts',(-4.26133239251396,-1.89486696261105,
72.720499690308));
#64123=CARTESIAN_POINT('Ctrl Pts',(-2.1112172128698,-4.71644095649861,72.8344248625374));
#64124=CARTESIAN_POINT('Ctrl Pts',(2.81733266516402,-4.33182294996633,72.9931856247833));
#64125=CARTESIAN_POINT('Ctrl Pts',(5.16737363149282,0.0174117376300544,
73.1519463870293));
#64126=CARTESIAN_POINT('Ctrl Pts',(2.78807641079671,4.35071067109887,73.3107071492751));
#64127=CARTESIAN_POINT('Ctrl Pts',(-2.14295350396336,4.70210630419026,73.469467911521));
#64128=CARTESIAN_POINT('Ctrl Pts',(-4.26731753777204,1.87500660994908,73.5830355644609));
#64129=CARTESIAN_POINT('Ctrl Pts',(-4.37751336374666,0.215028421847947,
73.6436829633189));
#64130=CARTESIAN_POINT('Ctrl Pts',(-4.37573799308197,0.00329254665532727,
73.6514101080949));
#64131=CARTESIAN_POINT('Ctrl Pts',(-4.37508401727703,0.00350862331529318,
72.848589891905));
#64132=CARTESIAN_POINT('Ctrl Pts',(-4.36445811409486,-1.21201843518349,
72.892932426549));
#64133=CARTESIAN_POINT('Ctrl Pts',(-3.20535851125622,-3.89598203052578,
72.9901952152748));
#64134=CARTESIAN_POINT('Ctrl Pts',(1.34123860080759,-4.99030391755056,73.140378258083));
#64135=CARTESIAN_POINT('Ctrl Pts',(4.91997252333115,-1.57984953191204,73.2991390203287));
#64136=CARTESIAN_POINT('Ctrl Pts',(3.99579730998455,3.27653140246455,73.4578997825747));
#64137=CARTESIAN_POINT('Ctrl Pts',(-0.585453654677876,5.13413071435083,
73.6166605448206));
#64138=CARTESIAN_POINT('Ctrl Pts',(-3.90388041542688,2.80342624447369,73.746890581264));
#64139=CARTESIAN_POINT('Ctrl Pts',(-4.36629549877317,0.673422924511184,
73.8242003636254));
#64140=CARTESIAN_POINT('Ctrl Pts',(-4.36501807785945,0.000928765700389245,
73.8485898919049));
#64141=CARTESIAN_POINT('Origin',(0.,0.,24.1514101080949));
#64142=CARTESIAN_POINT('',(-4.3651141969528,-0.00114447055126671,71.6514101080949));
#64143=CARTESIAN_POINT('',(-4.37610278806197,-0.00315032678594118,71.8485898919049));
#64144=CARTESIAN_POINT('',(-4.372,3.82579154166093E-12,24.1514101080949));
#64145=CARTESIAN_POINT('Ctrl Pts',(-4.3651141969528,-0.00114447055126629,
71.6514101080949));
#64146=CARTESIAN_POINT('Ctrl Pts',(-4.36665839117516,-0.660007333527467,
71.675306581002));
#64147=CARTESIAN_POINT('Ctrl Pts',(-3.91728495207162,-2.77596398718315,
71.7521233079911));
#64148=CARTESIAN_POINT('Ctrl Pts',(-0.63314364249968,-5.12846785541421,
71.8818602890621));
#64149=CARTESIAN_POINT('Ctrl Pts',(3.9651734499498,-3.31352575482195,72.040621051308));
#64150=CARTESIAN_POINT('Ctrl Pts',(4.93444268320512,1.53405632954553,72.1993818135539));
#64151=CARTESIAN_POINT('Ctrl Pts',(1.38755924827672,4.97762320275213,72.3581425757998));
#64152=CARTESIAN_POINT('Ctrl Pts',(-3.18397114357576,3.92214967618973,72.50881867398));
#64153=CARTESIAN_POINT('Ctrl Pts',(-4.36496403292504,1.22537573008428,72.6065745180785));
#64154=CARTESIAN_POINT('Ctrl Pts',(-4.37546659946853,-0.00338795269852542,
72.6514101080949));
#64155=CARTESIAN_POINT('Ctrl Pts',(-4.37610278806197,-0.00315032678594042,
71.8485898919049));
#64156=CARTESIAN_POINT('Ctrl Pts',(-4.37771416984263,-0.201332656341541,
71.8558239813086));
#64157=CARTESIAN_POINT('Ctrl Pts',(-4.27545064435103,-1.84762538881353,
71.9159783247941));
#64158=CARTESIAN_POINT('Ctrl Pts',(-2.18656114390733,-4.68198724237597,
72.0290529223616));
#64159=CARTESIAN_POINT('Ctrl Pts',(2.74752166081747,-4.3764344959288,72.1878136846077));
#64160=CARTESIAN_POINT('Ctrl Pts',(5.16698871742013,-0.0654352188752399,
72.3465744468534));
#64161=CARTESIAN_POINT('Ctrl Pts',(2.85746987211454,4.30545236923763,72.5053352090995));
#64162=CARTESIAN_POINT('Ctrl Pts',(-2.06729268270395,4.73585843726931,72.6640959713451));
#64163=CARTESIAN_POINT('Ctrl Pts',(-4.2529565583671,1.92226442851864,72.7785141989471));
#64164=CARTESIAN_POINT('Ctrl Pts',(-4.37713951584072,0.238642906024094,
72.840012172467));
#64165=CARTESIAN_POINT('Ctrl Pts',(-4.37508401727703,0.00350862331529318,
72.848589891905));
#64166=CARTESIAN_POINT('Origin',(0.,0.,24.1514101080949));
#64167=CARTESIAN_POINT('',(-4.37127157619262,0.00399172071570709,70.6514101080949));
#64168=CARTESIAN_POINT('',(-4.36532703354517,-0.00150807403881736,70.8485898919049));
#64169=CARTESIAN_POINT('',(-4.372,3.82579154166093E-12,24.1514101080949));
#64170=CARTESIAN_POINT('Ctrl Pts',(-4.37127157619262,0.00399172071570714,
70.6514101080949));
#64171=CARTESIAN_POINT('Ctrl Pts',(-4.36140746653353,-1.08694237129441,
70.6911183898435));
#64172=CARTESIAN_POINT('Ctrl Pts',(-3.39621711134158,-3.64736222930015,
70.7837469256742));
#64173=CARTESIAN_POINT('Ctrl Pts',(0.900757702520816,-5.08828939599587,
70.9292957155868));
#64174=CARTESIAN_POINT('Ctrl Pts',(4.76338297422217,-2.00305667841551,71.0880564778326));
#64175=CARTESIAN_POINT('Ctrl Pts',(4.26641464848803,2.9154346954137,71.2468172400786));
#64176=CARTESIAN_POINT('Ctrl Pts',(-0.135306682874774,5.16563118288797,
71.4055780023244));
#64177=CARTESIAN_POINT('Ctrl Pts',(-3.76928933575608,3.06100151884775,71.5404422916632));
#64178=CARTESIAN_POINT('Ctrl Pts',(-4.36323867518121,0.799086242725653,
71.62238632692));
#64179=CARTESIAN_POINT('Ctrl Pts',(-4.3651141969528,-0.00114447055126629,
71.6514101080949));
#64180=CARTESIAN_POINT('Ctrl Pts',(-4.36532703354517,-0.00150807403881757,
70.8485898919049));
#64181=CARTESIAN_POINT('Ctrl Pts',(-4.36729483924552,-0.636841944886774,
70.8716357901501));
#64182=CARTESIAN_POINT('Ctrl Pts',(-3.94000526365074,-2.72857085726927,
70.9476019424773));
#64183=CARTESIAN_POINT('Ctrl Pts',(-0.715283247733823,-5.11765806295492,
71.0764883488864));
#64184=CARTESIAN_POINT('Ctrl Pts',(3.91154054911197,-3.37667065413102,71.2352491111322));
#64185=CARTESIAN_POINT('Ctrl Pts',(4.95840295584866,1.45474887910182,71.3940098733782));
#64186=CARTESIAN_POINT('Ctrl Pts',(1.46718352100222,4.95473780229749,71.552770635624));
#64187=CARTESIAN_POINT('Ctrl Pts',(-3.14657975547223,3.96714821422749,71.7042973084663));
#64188=CARTESIAN_POINT('Ctrl Pts',(-4.36592626835323,1.24845026027391,71.8029037272266));
#64189=CARTESIAN_POINT('Ctrl Pts',(-4.37610278806197,-0.00315032678594042,
71.8485898919049));
#64190=CARTESIAN_POINT('Origin',(0.,0.,24.1514101080949));
#64191=CARTESIAN_POINT('',(-4.37870422100453,-0.0012994166445059,69.6514101080949));
#64192=CARTESIAN_POINT('',(-4.3705809381838,0.00395105542623939,69.848589891905));
#64193=CARTESIAN_POINT('',(-4.372,3.82579154166093E-12,24.1514101080949));
#64194=CARTESIAN_POINT('Ctrl Pts',(-4.37870422100453,-0.00129941664450634,
69.6514101080949));
#64195=CARTESIAN_POINT('Ctrl Pts',(-4.3789830325923,-0.0724121058889038,
69.6540099446031));
#64196=CARTESIAN_POINT('Ctrl Pts',(-4.34518999704772,-1.59076889411841,
69.7095300351934));
#64197=CARTESIAN_POINT('Ctrl Pts',(-2.58669250630018,-4.47337403912361,
69.8179703798655));
#64198=CARTESIAN_POINT('Ctrl Pts',(2.35523426198658,-4.5994483350962,69.9767311421114));
#64199=CARTESIAN_POINT('Ctrl Pts',(5.14157869213602,-0.51596702281012,70.1354919043573));
#64200=CARTESIAN_POINT('Ctrl Pts',(3.22219325167658,4.03974306916968,70.2942526666032));
#64201=CARTESIAN_POINT('Ctrl Pts',(-1.6462418758917,4.89815690868675,70.4530134288491));
#64202=CARTESIAN_POINT('Ctrl Pts',(-4.16716700492617,2.18017319825989,70.5720659093463));
#64203=CARTESIAN_POINT('Ctrl Pts',(-4.3745536205967,0.366973708511667,70.6381981357616));
#64204=CARTESIAN_POINT('Ctrl Pts',(-4.37127157619262,0.00399172071570714,
70.6514101080949));
#64205=CARTESIAN_POINT('Ctrl Pts',(-4.3705809381838,0.00395105542623928,
69.848589891905));
#64206=CARTESIAN_POINT('Ctrl Pts',(-4.36115189233779,-1.06404425239527,
69.8874475989916));
#64207=CARTESIAN_POINT('Ctrl Pts',(-3.42928322572819,-3.60126660220352,
69.9792255601602));
#64208=CARTESIAN_POINT('Ctrl Pts',(0.819065126108891,-5.102076684352,70.1239237754111));
#64209=CARTESIAN_POINT('Ctrl Pts',(4.73065728621489,-2.07916709626671,70.2826845376568));
#64210=CARTESIAN_POINT('Ctrl Pts',(4.31260739816882,2.84665972730784,70.4414452999028));
#64211=CARTESIAN_POINT('Ctrl Pts',(-0.0524725109896868,5.16713661609669,
70.6002060621488));
#64212=CARTESIAN_POINT('Ctrl Pts',(-3.74285914641375,3.1081338808624,70.7359209261493));
#64213=CARTESIAN_POINT('Ctrl Pts',(-4.36277617060702,0.822074063266301,
70.8187155360681));
#64214=CARTESIAN_POINT('Ctrl Pts',(-4.36532703354517,-0.00150807403881757,
70.8485898919049));
#64215=CARTESIAN_POINT('Origin',(0.,0.,24.1514101080949));
#64216=CARTESIAN_POINT('',(-4.36744694438276,-0.00316878230680772,68.6514101080949));
#64217=CARTESIAN_POINT('',(-4.37895590169143,-0.000884728325120654,68.848589891905));
#64218=CARTESIAN_POINT('',(-4.372,3.82579154166093E-12,24.1514101080949));
#64219=CARTESIAN_POINT('Ctrl Pts',(-4.36744694438276,-0.0031687823068071,
68.6514101080949));
#64220=CARTESIAN_POINT('Ctrl Pts',(-4.37084913112638,-0.510127366468858,
68.6698217534447));
#64221=CARTESIAN_POINT('Ctrl Pts',(-4.05501785193817,-2.47012128343436,
68.7411536528764));
#64222=CARTESIAN_POINT('Ctrl Pts',(-1.15903350388962,-5.03574172817834,
68.8654058063903));
#64223=CARTESIAN_POINT('Ctrl Pts',(3.60203679805415,-3.70504849111566,69.0241665686361));
#64224=CARTESIAN_POINT('Ctrl Pts',(5.06641299677213,1.01661829719571,69.182927330882));
#64225=CARTESIAN_POINT('Ctrl Pts',(1.89385326524434,4.80784496690336,69.3416880931279));
#64226=CARTESIAN_POINT('Ctrl Pts',(-2.93168118063718,4.20875891624129,69.4978490188655));
#64227=CARTESIAN_POINT('Ctrl Pts',(-4.37330776031301,1.37510260179151,69.6010896905212));
#64228=CARTESIAN_POINT('Ctrl Pts',(-4.37870422100453,-0.00129941664450634,
69.6514101080949));
#64229=CARTESIAN_POINT('Ctrl Pts',(-4.37895590169143,-0.00088472832512114,
68.848589891905));
#64230=CARTESIAN_POINT('Ctrl Pts',(-4.37908827342486,-0.0487245072402155,
68.8503391537513));
#64231=CARTESIAN_POINT('Ctrl Pts',(-4.35670634828455,-1.54372976222875,
68.9050086696796));
#64232=CARTESIAN_POINT('Ctrl Pts',(-2.65807841962993,-4.43132861441282,
69.0125984396897));
#64233=CARTESIAN_POINT('Ctrl Pts',(2.2811920004135,-4.63661700284439,69.1713592019357));
#64234=CARTESIAN_POINT('Ctrl Pts',(5.1326458217616,-0.598331882962418,69.3301199641815));
#64235=CARTESIAN_POINT('Ctrl Pts',(3.28654540832559,3.98756485249208,69.4888807264275));
#64236=CARTESIAN_POINT('Ctrl Pts',(-1.56750175164667,4.92392043319156,69.6476414886732));
#64237=CARTESIAN_POINT('Ctrl Pts',(-4.14999820818835,2.2275746797718,69.7675445438326));
#64238=CARTESIAN_POINT('Ctrl Pts',(-4.37399329599569,0.390456985212737,
69.8345273449097));
#64239=CARTESIAN_POINT('Ctrl Pts',(-4.3705809381838,0.00395105542623928,
69.848589891905));
#64240=CARTESIAN_POINT('Origin',(0.,0.,24.1514101080949));
#64241=CARTESIAN_POINT('',(-4.36727426748866,0.00308741741996557,67.6514101080949));
#64242=CARTESIAN_POINT('',(-4.36799009248299,-0.00339142969553563,67.8485898919049));
#64243=CARTESIAN_POINT('',(-4.372,3.82579154166093E-12,24.1514101080949));
#64244=CARTESIAN_POINT('Ctrl Pts',(-4.36727426748866,0.0030874174199657,
67.6514101080949));
#64245=CARTESIAN_POINT('Ctrl Pts',(-4.36112833884136,-0.939337788388386,
67.6856335622863));
#64246=CARTESIAN_POINT('Ctrl Pts',(-3.59904165290846,-3.34810943987296,
67.7727772705596));
#64247=CARTESIAN_POINT('Ctrl Pts',(0.370823889097725,-5.15408023407956,
67.9128412329148));
#64248=CARTESIAN_POINT('Ctrl Pts',(4.53122783943781,-2.48395404207855,68.0716019951608));
#64249=CARTESIAN_POINT('Ctrl Pts',(4.5445136629679,2.45956276259679,68.2303627574067));
#64250=CARTESIAN_POINT('Ctrl Pts',(0.398521768172548,5.15201259862078,68.3891235196525));
#64251=CARTESIAN_POINT('Ctrl Pts',(-3.58909538685354,3.36377270257325,68.5294726365487));
#64252=CARTESIAN_POINT('Ctrl Pts',(-4.36107028825353,0.947014381222592,
68.6169014993627));
#64253=CARTESIAN_POINT('Ctrl Pts',(-4.36744694438276,-0.0031687823068071,
68.6514101080949));
#64254=CARTESIAN_POINT('Ctrl Pts',(-4.36799009248299,-0.00339142969553514,
67.8485898919049));
#64255=CARTESIAN_POINT('Ctrl Pts',(-4.37149165529305,-0.486778408785156,
67.8661509625928));
#64256=CARTESIAN_POINT('Ctrl Pts',(-4.07455789488293,-2.42267137940883,
67.9366322873626));
#64257=CARTESIAN_POINT('Ctrl Pts',(-1.23961891643423,-5.01651264483955,
68.0600338662145));
#64258=CARTESIAN_POINT('Ctrl Pts',(3.54217356679019,-3.76232117137135,68.2187946284603));
#64259=CARTESIAN_POINT('Ctrl Pts',(5.08206060458778,0.935261559732356,68.3775553907062));
#64260=CARTESIAN_POINT('Ctrl Pts',(1.97069054350433,4.77686434343271,68.5363161529522));
#64261=CARTESIAN_POINT('Ctrl Pts',(-2.89016105242335,4.25237825733215,68.6933276533517));
#64262=CARTESIAN_POINT('Ctrl Pts',(-4.37508364382578,1.39856782394589,68.7974188996693));
#64263=CARTESIAN_POINT('Ctrl Pts',(-4.37895590169143,-0.00088472832512114,
68.848589891905));
#64264=CARTESIAN_POINT('Origin',(0.,0.,24.1514101080949));
#64265=CARTESIAN_POINT('',(-4.37860089698225,0.00143482616460942,66.6514101080949));
#64266=CARTESIAN_POINT('',(-4.36678925203502,0.00282595512297229,66.8485898919049));
#64267=CARTESIAN_POINT('',(-4.372,3.82579154166093E-12,24.1514101080949));
#64268=CARTESIAN_POINT('Ctrl Pts',(-4.37860089698225,0.00143482616460969,
66.6514101080949));
#64269=CARTESIAN_POINT('Ctrl Pts',(-4.37274293747686,-1.3672535432393,66.7014453711278));
#64270=CARTESIAN_POINT('Ctrl Pts',(-2.94545539126712,-4.19408159696058,
66.8044008882426));
#64271=CARTESIAN_POINT('Ctrl Pts',(1.86798369006022,-4.81795499664787,66.9602766594396));
#64272=CARTESIAN_POINT('Ctrl Pts',(5.06087547593053,-1.04383563513614,67.1190374216854));
#64273=CARTESIAN_POINT('Ctrl Pts',(3.62189943977487,3.68563398402679,67.2777981839313));
#64274=CARTESIAN_POINT('Ctrl Pts',(-1.13194959602156,5.04189880185246,67.4365589461772));
#64275=CARTESIAN_POINT('Ctrl Pts',(-4.04836008668961,2.48602916041319,67.5610962542317));
#64276=CARTESIAN_POINT('Ctrl Pts',(-4.37063188292449,0.517948815873062,
67.6327133082043));
#64277=CARTESIAN_POINT('Ctrl Pts',(-4.36727426748866,0.0030874174199657,
67.6514101080949));
#64278=CARTESIAN_POINT('Ctrl Pts',(-4.36678925203502,0.00282595512297222,
66.8485898919049));
#64279=CARTESIAN_POINT('Ctrl Pts',(-4.36134189412171,-0.916433051844979,
66.8819627714344));
#64280=CARTESIAN_POINT('Ctrl Pts',(-3.62832781641238,-3.30133069322053,
66.9682559050458));
#64281=CARTESIAN_POINT('Ctrl Pts',(0.288144638596748,-5.15936302667923,
67.1074692927391));
#64282=CARTESIAN_POINT('Ctrl Pts',(4.49082211047655,-2.55628068604989,67.266230054985));
#64283=CARTESIAN_POINT('Ctrl Pts',(4.58336201290063,2.38638782106256,67.4249908172308));
#64284=CARTESIAN_POINT('Ctrl Pts',(0.481069000502546,5.14496130117338,67.5837515794768));
#64285=CARTESIAN_POINT('Ctrl Pts',(-3.55904252406398,3.41043311335412,67.7249512710348));
#64286=CARTESIAN_POINT('Ctrl Pts',(-4.36093970223245,0.969907359868089,
67.8132307085108));
#64287=CARTESIAN_POINT('Ctrl Pts',(-4.36799009248299,-0.00339142969553514,
67.8485898919049));
#64288=CARTESIAN_POINT('Origin',(0.,0.,24.1514101080949));
#64289=CARTESIAN_POINT('',(-4.37150619923976,-0.00399650483370713,65.6514101080949));
#64290=CARTESIAN_POINT('',(-4.37824072692977,0.00182550535674644,65.8485898919049));
#64291=CARTESIAN_POINT('',(-4.372,3.82579154166093E-12,24.1514101080949));
#64292=CARTESIAN_POINT('Ctrl Pts',(-4.37150619923976,-0.00399650483370689,
65.6514101080949));
#64293=CARTESIAN_POINT('Ctrl Pts',(-4.37473632420811,-0.359095615586663,
65.6643369258874));
#64294=CARTESIAN_POINT('Ctrl Pts',(-4.17282222069464,-2.16428561428065,
65.7301839977619));
#64295=CARTESIAN_POINT('Ctrl Pts',(-1.67254574036732,-4.88923758498539,
65.8489513237183));
#64296=CARTESIAN_POINT('Ctrl Pts',(3.20043304382085,-4.05700403599433,66.0077120859643));
#64297=CARTESIAN_POINT('Ctrl Pts',(5.14427774780404,0.488323529540513,66.16647284821));
#64298=CARTESIAN_POINT('Ctrl Pts',(2.3799223229872,4.58672248480354,66.3252336104561));
#64299=CARTESIAN_POINT('Ctrl Pts',(-2.56261070750152,4.48721291871176,66.4839943727018));
#64300=CARTESIAN_POINT('Ctrl Pts',(-4.34124164729195,1.60654622778481,66.5927198719149));
#64301=CARTESIAN_POINT('Ctrl Pts',(-4.37893866198466,0.0803522427089276,
66.6485251170459));
#64302=CARTESIAN_POINT('Ctrl Pts',(-4.37860089698225,0.00143482616460969,
66.6514101080949));
#64303=CARTESIAN_POINT('Ctrl Pts',(-4.37824072692977,0.00182550535674642,
65.8485898919049));
#64304=CARTESIAN_POINT('Ctrl Pts',(-4.37114754505431,-1.34389016319695,
65.8977745802759));
#64305=CARTESIAN_POINT('Ctrl Pts',(-2.98610974303986,-4.15014526257514,
65.9998795227288));
#64306=CARTESIAN_POINT('Ctrl Pts',(1.79050088812788,-4.84728385216189,66.1549047192638));
#64307=CARTESIAN_POINT('Ctrl Pts',(5.04349004573647,-1.12483880283976,66.3136654815096));
#64308=CARTESIAN_POINT('Ctrl Pts',(3.68052305807757,3.62709307749002,66.4724262437556));
#64309=CARTESIAN_POINT('Ctrl Pts',(-1.05097105537457,5.05939858230018,66.6311870060014));
#64310=CARTESIAN_POINT('Ctrl Pts',(-4.02817917541877,2.53347937952348,66.7565748887179));
#64311=CARTESIAN_POINT('Ctrl Pts',(-4.36997991304344,0.541260167974116,
66.8290425173524));
#64312=CARTESIAN_POINT('Ctrl Pts',(-4.36678925203502,0.00282595512297222,
66.8485898919049));
#64313=CARTESIAN_POINT('Origin',(0.,0.,24.1514101080949));
#64314=CARTESIAN_POINT('',(-4.36505611781897,0.00102009982110932,64.6514101080949));
#64315=CARTESIAN_POINT('',(-4.37221209240493,-0.00398401159164008,64.848589891905));
#64316=CARTESIAN_POINT('',(-4.372,3.82579154166093E-12,24.1514101080949));
#64317=CARTESIAN_POINT('Ctrl Pts',(-4.36505611781897,0.00102009982110941,
64.6514101080949));
#64318=CARTESIAN_POINT('Ctrl Pts',(-4.36340207653842,-0.791374776421536,
64.680148734729));
#64319=CARTESIAN_POINT('Ctrl Pts',(-3.7780282066601,-3.04518855619851,64.7618076154451));
#64320=CARTESIAN_POINT('Ctrl Pts',(-0.163070050579303,-5.16482928804609,
64.8963867502428));
#64321=CARTESIAN_POINT('Ctrl Pts',(4.25068252576661,-2.93832460446375,65.0551475124889));
#64322=CARTESIAN_POINT('Ctrl Pts',(4.77408061574266,1.97742450941745,65.2139082747347));
#64323=CARTESIAN_POINT('Ctrl Pts',(0.928094299999949,5.08337431106172,65.3726690369806));
#64324=CARTESIAN_POINT('Ctrl Pts',(-3.38499698876322,3.66278651613716,65.518502981434));
#64325=CARTESIAN_POINT('Ctrl Pts',(-4.36151272681657,1.09462141415472,65.6114166718055));
#64326=CARTESIAN_POINT('Ctrl Pts',(-4.37150619923976,-0.00399650483370689,
65.6514101080949));
#64327=CARTESIAN_POINT('Ctrl Pts',(-4.37221209240492,-0.00398401159164036,
64.848589891905));
#64328=CARTESIAN_POINT('Ctrl Pts',(-4.37526481066381,-0.335581023561335,
64.8606661350355));
#64329=CARTESIAN_POINT('Ctrl Pts',(-4.18939334686749,-2.11690750379085,
64.925662632248));
#64330=CARTESIAN_POINT('Ctrl Pts',(-1.75071636731768,-4.86179456322688,
65.0435793835425));
#64331=CARTESIAN_POINT('Ctrl Pts',(3.1349787773885,-4.10779286711735,65.2023401457884));
#64332=CARTESIAN_POINT('Ctrl Pts',(5.15144558585509,0.405786335144852,65.3611009080343));
#64333=CARTESIAN_POINT('Ctrl Pts',(2.45315204119292,4.54797748857745,65.5198616702802));
#64334=CARTESIAN_POINT('Ctrl Pts',(-2.49034118407384,4.52772072468283,65.6786224325261));
#64335=CARTESIAN_POINT('Ctrl Pts',(-4.32920116011288,1.65362984026736,65.788198506401));
#64336=CARTESIAN_POINT('Ctrl Pts',(-4.37877945245337,0.104032299273348,
65.844854326194));
#64337=CARTESIAN_POINT('Ctrl Pts',(-4.37824072692977,0.00182550535674642,
65.8485898919049));
#64338=CARTESIAN_POINT('Origin',(0.,0.,24.1514101080949));
#64339=CARTESIAN_POINT('',(-4.37524640365158,0.00345929889477671,63.6514101080949));
#64340=CARTESIAN_POINT('',(-4.36492309298158,0.000643490633093768,63.848589891905));
#64341=CARTESIAN_POINT('',(-4.372,3.82579154166093E-12,24.1514101080949));
#64342=CARTESIAN_POINT('Ctrl Pts',(-4.37524640365158,0.00345929889477663,
63.6514101080949));
#64343=CARTESIAN_POINT('Ctrl Pts',(-4.36466684100657,-1.21764908937452,
63.6959605435705));
#64344=CARTESIAN_POINT('Ctrl Pts',(-3.19636598506899,-3.90702309781776,
63.7934312331281));
#64345=CARTESIAN_POINT('Ctrl Pts',(1.36078442693529,-4.98500944427043,63.9438221767676));
#64346=CARTESIAN_POINT('Ctrl Pts',(4.92612583383742,-1.56055685101642,64.1025829390136));
#64347=CARTESIAN_POINT('Ctrl Pts',(3.98292640713875,3.29216504011747,64.2613437012594));
#64348=CARTESIAN_POINT('Ctrl Pts',(-0.605568927444514,5.13179692604536,
64.4201044635054));
#64349=CARTESIAN_POINT('Ctrl Pts',(-3.90955357406592,2.79184753823524,64.5501265991171));
#64350=CARTESIAN_POINT('Ctrl Pts',(-4.36644788265656,0.667767259764548,
64.627228480647));
#64351=CARTESIAN_POINT('Ctrl Pts',(-4.36505611781897,0.00102009982110941,
64.6514101080949));
#64352=CARTESIAN_POINT('Ctrl Pts',(-4.36492309298158,0.000643490633093699,
63.8485898919049));
#64353=CARTESIAN_POINT('Ctrl Pts',(-4.36391231627522,-0.768357459497397,
63.876477943877));
#64354=CARTESIAN_POINT('Ctrl Pts',(-3.80373422012026,-2.9979881039429,63.9572862499311));
#64355=CARTESIAN_POINT('Ctrl Pts',(-0.245853021615901,-5.16155116855183,
64.0910148100673));
#64356=CARTESIAN_POINT('Ctrl Pts',(4.20302825930282,-3.00609507922124,64.249775572313));
#64357=CARTESIAN_POINT('Ctrl Pts',(4.80516969413782,1.90063104898239,64.408536334559));
#64358=CARTESIAN_POINT('Ctrl Pts',(1.00947304907845,5.06784158562605,64.5672970968048));
#64359=CARTESIAN_POINT('Ctrl Pts',(-3.35112485942778,3.70870379987186,64.7139816159202));
#64360=CARTESIAN_POINT('Ctrl Pts',(-4.36188725407156,1.11753630245885,64.8077458809536));
#64361=CARTESIAN_POINT('Ctrl Pts',(-4.37221209240492,-0.00398401159164036,
64.848589891905));
#64362=CARTESIAN_POINT('Origin',(0.,0.,24.1514101080949));
#64363=CARTESIAN_POINT('',(-4.37595036350582,-0.00321178070193251,62.6514101080949));
#64364=CARTESIAN_POINT('',(-4.37457294606715,0.00364650982632456,62.848589891905));
#64365=CARTESIAN_POINT('',(-4.372,3.82579154166093E-12,24.1514101080949));
#64366=CARTESIAN_POINT('Ctrl Pts',(-4.37595036350582,-0.00321178070193263,
62.6514101080949));
#64367=CARTESIAN_POINT('Ctrl Pts',(-4.37763091892069,-0.207108192738585,
62.6588520983301));
#64368=CARTESIAN_POINT('Ctrl Pts',(-4.27203828701875,-1.85916971844638,
62.7192143426473));
#64369=CARTESIAN_POINT('Ctrl Pts',(-2.16819641913028,-4.69051998227545,
62.8324968410464));
#64370=CARTESIAN_POINT('Ctrl Pts',(2.76465101981334,-4.3656337632353,62.9912576032923));
#64371=CARTESIAN_POINT('Ctrl Pts',(5.16720539805885,-0.0451861740625634,
63.1500183655382));
#64372=CARTESIAN_POINT('Ctrl Pts',(2.8405755616569,4.31661718184185,63.308779127784));
#64373=CARTESIAN_POINT('Ctrl Pts',(-2.08583579528372,4.72772064013601,63.46753989003));
#64374=CARTESIAN_POINT('Ctrl Pts',(-4.25650552345673,1.91071093035616,63.5817502168002));
#64375=CARTESIAN_POINT('Ctrl Pts',(-4.37723401655206,0.232872448270317,
63.6430402894885));
#64376=CARTESIAN_POINT('Ctrl Pts',(-4.37524640365158,0.00345929889477663,
63.6514101080949));
#64377=CARTESIAN_POINT('Ctrl Pts',(-4.37457294606715,0.00364650982632473,
62.848589891905));
#64378=CARTESIAN_POINT('Ctrl Pts',(-4.36385410668696,-1.19462603572661,
62.8922897527186));
#64379=CARTESIAN_POINT('Ctrl Pts',(-3.23292058066413,-3.86178527014851,
62.9889098676142));
#64380=CARTESIAN_POINT('Ctrl Pts',(1.28068854395033,-5.00618527695598,63.1384502365919));
#64381=CARTESIAN_POINT('Ctrl Pts',(4.90047350742458,-1.63933327204883,63.2972109988377));
#64382=CARTESIAN_POINT('Ctrl Pts',(4.03519542999152,3.22788661752423,63.4559717610837));
#64383=CARTESIAN_POINT('Ctrl Pts',(-0.523216761619089,5.14084607765855,
63.6147325233295));
#64384=CARTESIAN_POINT('Ctrl Pts',(-3.886148042221,2.83920884682887,63.7456052336033));
#64385=CARTESIAN_POINT('Ctrl Pts',(-4.3658303620453,0.690895618159912,63.8235576897951));
#64386=CARTESIAN_POINT('Ctrl Pts',(-4.36492309298158,0.000643490633093699,
63.8485898919049));
#64387=CARTESIAN_POINT('Origin',(0.,0.,24.1514101080949));
#64388=CARTESIAN_POINT('',(-4.36526954399882,-0.00142033253192601,61.6514101080949));
#64389=CARTESIAN_POINT('',(-4.37655926179451,-0.0029470014875782,61.848589891905));
#64390=CARTESIAN_POINT('',(-4.372,3.82579154166093E-12,24.1514101080949));
#64391=CARTESIAN_POINT('Ctrl Pts',(-4.36526954399882,-0.00142033253192606,
61.6514101080949));
#64392=CARTESIAN_POINT('Ctrl Pts',(-4.36713817680575,-0.642506710603713,
61.6746639071717));
#64393=CARTESIAN_POINT('Ctrl Pts',(-3.93449886856382,-2.74015675637768,
61.7508379603305));
#64394=CARTESIAN_POINT('Ctrl Pts',(-0.695222522116061,-5.12042176590928,
61.879932267571));
#64395=CARTESIAN_POINT('Ctrl Pts',(3.92474305071123,-3.3613160223265,62.038693029817));
#64396=CARTESIAN_POINT('Ctrl Pts',(4.95266390069012,1.47416881762428,62.1974537920629));
#64397=CARTESIAN_POINT('Ctrl Pts',(1.4477554676688,4.96044932661243,62.3562145543087));
#64398=CARTESIAN_POINT('Ctrl Pts',(-3.15577720759182,3.95616660035224,62.5075333263195));
#64399=CARTESIAN_POINT('Ctrl Pts',(-4.36568043030908,1.24280635839108,62.6059318442481));
#64400=CARTESIAN_POINT('Ctrl Pts',(-4.37595036350582,-0.00321178070193263,
62.6514101080949));
#64401=CARTESIAN_POINT('Ctrl Pts',(-4.37655926179451,-0.00294700148757761,
61.848589891905));
#64402=CARTESIAN_POINT('Ctrl Pts',(-4.37795768436782,-0.183473677232841,
61.8551813074782));
#64403=CARTESIAN_POINT('Ctrl Pts',(-4.28584228404936,-1.81194987404807,
61.9146929771335));
#64404=CARTESIAN_POINT('Ctrl Pts',(-2.24311745571471,-4.65515609337478,
62.0271249008706));
#64405=CARTESIAN_POINT('Ctrl Pts',(2.69430472161155,-4.40939635788372,62.1858856631165));
#64406=CARTESIAN_POINT('Ctrl Pts',(5.16581691910958,-0.128022388891978,
62.3446464253625));
#64407=CARTESIAN_POINT('Ctrl Pts',(2.90941568030617,4.27052158090844,62.5034071876082));
#64408=CARTESIAN_POINT('Ctrl Pts',(-2.00977165837252,4.76055375508134,62.6621679498542));
#64409=CARTESIAN_POINT('Ctrl Pts',(-4.24182569275328,1.95798917979278,62.7772288512864));
#64410=CARTESIAN_POINT('Ctrl Pts',(-4.37683455314381,0.256474411491908,
62.8393694986367));
#64411=CARTESIAN_POINT('Ctrl Pts',(-4.37457294606715,0.00364650982632473,
62.848589891905));
#64412=CARTESIAN_POINT('Origin',(0.,0.,24.1514101080949));
#64413=CARTESIAN_POINT('',(-4.37074823605818,0.00396461597538121,60.6514101080949));
#64414=CARTESIAN_POINT('',(-4.36552637203463,-0.001773948386046,60.848589891905));
#64415=CARTESIAN_POINT('',(-4.372,3.82579154166093E-12,24.1514101080949));
#64416=CARTESIAN_POINT('Ctrl Pts',(-4.37074823605818,0.00396461597538186,
60.6514101080949));
#64417=CARTESIAN_POINT('Ctrl Pts',(-4.36120638422482,-1.0696402047533,60.6904757160132));
#64418=CARTESIAN_POINT('Ctrl Pts',(-3.42125648388678,-3.61254525965742,
60.7824615780135));
#64419=CARTESIAN_POINT('Ctrl Pts',(0.839052987504236,-5.09882765939536,
60.9273676940957));
#64420=CARTESIAN_POINT('Ctrl Pts',(4.73876879287487,-2.06061246810993,61.0861284563416));
#64421=CARTESIAN_POINT('Ctrl Pts',(4.30141865142892,2.86353819621711,61.2448892185875));
#64422=CARTESIAN_POINT('Ctrl Pts',(-0.0727212283482856,5.16689123545314,
61.4036499808334));
#64423=CARTESIAN_POINT('Ctrl Pts',(-3.74936971792349,3.0966186529212,61.5391569440025));
#64424=CARTESIAN_POINT('Ctrl Pts',(-4.36288560187799,0.816457216282587,
61.6217436530897));
#64425=CARTESIAN_POINT('Ctrl Pts',(-4.36526954399882,-0.00142033253192606,
61.6514101080949));
#64426=CARTESIAN_POINT('Ctrl Pts',(-4.36552637203463,-0.00177394838604503,
60.848589891905));
#64427=CARTESIAN_POINT('Ctrl Pts',(-4.36778246279527,-0.619319994324535,
60.8709931163198));
#64428=CARTESIAN_POINT('Ctrl Pts',(-3.95683545179798,-2.6927488906017,60.9463165948165));
#64429=CARTESIAN_POINT('Ctrl Pts',(-0.777225152475865,-5.10861774222493,
61.0745603273954));
#64430=CARTESIAN_POINT('Ctrl Pts',(3.87034915924295,-3.42380658907068,61.2333210896411));
#64431=CARTESIAN_POINT('Ctrl Pts',(4.97566169906822,1.39457693593507,61.3920818518871));
#64432=CARTESIAN_POINT('Ctrl Pts',(1.52709666834069,4.93660105126586,61.550842614133));
#64433=CARTESIAN_POINT('Ctrl Pts',(-3.11790932935563,4.00102289357066,61.7030119608056));
#64434=CARTESIAN_POINT('Ctrl Pts',(-4.36673022084793,1.26591415802506,61.8022610533963));
#64435=CARTESIAN_POINT('Ctrl Pts',(-4.37655926179451,-0.00294700148757761,
61.848589891905));
#64436=CARTESIAN_POINT('Origin',(0.,0.,24.1514101080949));
#64437=CARTESIAN_POINT('',(-4.37890245970854,-0.00098741172007078,59.6514101080949));
#64438=CARTESIAN_POINT('',(-4.37007084553272,0.00389455484668386,59.848589891905));
#64439=CARTESIAN_POINT('',(-4.372,3.82579154166093E-12,24.1514101080949));
#64440=CARTESIAN_POINT('Ctrl Pts',(-4.37890245970854,-0.000987411720070989,
59.6514101080949));
#64441=CARTESIAN_POINT('Ctrl Pts',(-4.37906627500205,-0.054514724532804,
59.6533672707728));
#64442=CARTESIAN_POINT('Ctrl Pts',(-4.35392740184128,-1.55522413176342,
59.7082446875327));
#64443=CARTESIAN_POINT('Ctrl Pts',(-2.6406923556686,-4.44171107781315,59.8160423583745));
#64444=CARTESIAN_POINT('Ctrl Pts',(2.29934455736468,-4.62764173446609,59.9748031206204));
#64445=CARTESIAN_POINT('Ctrl Pts',(5.13495109710383,-0.578213322578349,
60.1335638828663));
#64446=CARTESIAN_POINT('Ctrl Pts',(3.27089354364999,4.00041358388897,60.2923246451122));
#64447=CARTESIAN_POINT('Ctrl Pts',(-1.58678569169648,4.91773978415717,60.451085407358));
#64448=CARTESIAN_POINT('Ctrl Pts',(-4.15423631088884,2.21598713963915,60.5707805616856));
#64449=CARTESIAN_POINT('Ctrl Pts',(-4.37413226072698,0.384719343814296,
60.6375554619313));
#64450=CARTESIAN_POINT('Ctrl Pts',(-4.37074823605818,0.00396461597538186,
60.6514101080949));
#64451=CARTESIAN_POINT('Ctrl Pts',(-4.37007084553272,0.00389455484668389,
59.848589891905));
#64452=CARTESIAN_POINT('Ctrl Pts',(-4.36101477584936,-1.0467484993519,59.8868049251613));
#64453=CARTESIAN_POINT('Ctrl Pts',(-3.45386988791881,-3.56635453916342,
59.9779402124996));
#64454=CARTESIAN_POINT('Ctrl Pts',(0.757199388556149,-5.11162432694214,
60.12199575392));
#64455=CARTESIAN_POINT('Ctrl Pts',(4.70512351821232,-2.13632086826434,60.2807565161658));
#64456=CARTESIAN_POINT('Ctrl Pts',(4.34677488413138,2.79420870381954,60.4395172784118));
#64457=CARTESIAN_POINT('Ctrl Pts',(0.0101251021257834,5.16739311995163,
60.5982780406576));
#64458=CARTESIAN_POINT('Ctrl Pts',(-3.72252569100569,3.14370820853236,60.7346355784887));
#64459=CARTESIAN_POINT('Ctrl Pts',(-4.36245318991586,0.839429561242695,
60.8180728622378));
#64460=CARTESIAN_POINT('Ctrl Pts',(-4.36552637203463,-0.00177394838604503,
60.848589891905));
#64461=CARTESIAN_POINT('Origin',(0.,0.,24.1514101080949));
#64462=CARTESIAN_POINT('',(-4.36785354673662,-0.00333986239341869,58.6514101080949));
#64463=CARTESIAN_POINT('',(-4.37908572622912,-0.000563059365845109,58.848589891905));
#64464=CARTESIAN_POINT('',(-4.372,3.82579154166093E-12,24.1514101080949));
#64465=CARTESIAN_POINT('Ctrl Pts',(-4.36785354673662,-0.00333986239341826,
58.6514101080949));
#64466=CARTESIAN_POINT('Ctrl Pts',(-4.3713354267805,-0.492488022383476,
58.6691790796144));
#64467=CARTESIAN_POINT('Ctrl Pts',(-4.0698257693161,-2.43426901092249,58.7398683052158));
#64468=CARTESIAN_POINT('Ctrl Pts',(-1.21995052871669,-5.02133190732686,
58.8634777848992));
#64469=CARTESIAN_POINT('Ctrl Pts',(3.55689020801282,-3.74841105859499,59.022238547145));
#64470=CARTESIAN_POINT('Ctrl Pts',(5.07835637974298,0.955170087669591,59.1809993093909));
#64471=CARTESIAN_POINT('Ctrl Pts',(1.95195567231696,4.78455039364876,59.3397600716368));
#64472=CARTESIAN_POINT('Ctrl Pts',(-2.90036961753982,4.24173919554959,59.4965636712048));
#64473=CARTESIAN_POINT('Ctrl Pts',(-4.37463682871597,1.39282484839483,59.6004470166909));
#64474=CARTESIAN_POINT('Ctrl Pts',(-4.37890245970854,-0.000987411720070989,
59.6514101080949));
#64475=CARTESIAN_POINT('Ctrl Pts',(-4.37908572622912,-0.000563059365844233,
58.848589891905));
#64476=CARTESIAN_POINT('Ctrl Pts',(-4.37914057971478,-0.0308242308936409,
58.8496964799209));
#64477=CARTESIAN_POINT('Ctrl Pts',(-4.36515029335745,-1.50821048731078,
58.9037233220189));
#64478=CARTESIAN_POINT('Ctrl Pts',(-2.71156370034918,-4.39880398208026,
59.0106704181988));
#64479=CARTESIAN_POINT('Ctrl Pts',(2.22485747409188,-4.66391074033302,59.1694311804446));
#64480=CARTESIAN_POINT('Ctrl Pts',(5.12502112908765,-0.660463928024547,
59.3281919426906));
#64481=CARTESIAN_POINT('Ctrl Pts',(3.33460890093368,3.94745964534539,59.4869527049363));
#64482=CARTESIAN_POINT('Ctrl Pts',(-1.5077392503099,4.94254757457034,59.6457134671823));
#64483=CARTESIAN_POINT('Ctrl Pts',(-4.13672535981933,2.2634000371691,59.7662591961718));
#64484=CARTESIAN_POINT('Ctrl Pts',(-4.37355563916387,0.408184092349566,
59.8338846710794));
#64485=CARTESIAN_POINT('Ctrl Pts',(-4.37007084553272,0.00389455484668389,
59.848589891905));
#64486=CARTESIAN_POINT('Origin',(0.,0.,24.1514101080949));
#64487=CARTESIAN_POINT('',(-4.36690348533115,0.0028923709500598,57.6514101080949));
#64488=CARTESIAN_POINT('',(-4.36842637263245,-0.00353866609716813,57.848589891905));
#64489=CARTESIAN_POINT('',(-4.372,3.82579154166093E-12,24.1514101080949));
#64490=CARTESIAN_POINT('Ctrl Pts',(-4.36690348533115,0.00289237095005987,
57.6514101080949));
#64491=CARTESIAN_POINT('Ctrl Pts',(-4.36128421030265,-0.922032505654121,
57.6849908884559));
#64492=CARTESIAN_POINT('Ctrl Pts',(-3.62122223271516,-3.31277225264101,
57.7714919228989));
#64493=CARTESIAN_POINT('Ctrl Pts',(0.308361079608735,-5.1581941472416,57.9109132114238));
#64494=CARTESIAN_POINT('Ctrl Pts',(4.50080518836808,-2.53866226040682,58.0696739736697));
#64495=CARTESIAN_POINT('Ctrl Pts',(4.57397490984839,2.40433087160068,58.2284347359156));
#64496=CARTESIAN_POINT('Ctrl Pts',(0.460903079952699,5.14680694867653,58.3871954981615));
#64497=CARTESIAN_POINT('Ctrl Pts',(-3.56644148611271,3.39903679271645,58.5281872888879));
#64498=CARTESIAN_POINT('Ctrl Pts',(-4.36096555385885,0.964312382866099,
58.6162588255324));
#64499=CARTESIAN_POINT('Ctrl Pts',(-4.36785354673662,-0.00333986239341826,
58.6514101080949));
#64500=CARTESIAN_POINT('Ctrl Pts',(-4.36842637263245,-0.00353866609716848,
57.848589891905));
#64501=CARTESIAN_POINT('Ctrl Pts',(-4.37197022738872,-0.469118111917197,
57.8655082887625));
#64502=CARTESIAN_POINT('Ctrl Pts',(-4.08900712877109,-2.3868217079302,57.935346939702));
#64503=CARTESIAN_POINT('Ctrl Pts',(-1.30029709065152,-5.00112803773905,
58.0581058447233));
#64504=CARTESIAN_POINT('Ctrl Pts',(3.49633757827368,-3.80495436405849,58.2168666069693));
#64505=CARTESIAN_POINT('Ctrl Pts',(5.09301729854088,0.873629767452735,58.3756273692151));
#64506=CARTESIAN_POINT('Ctrl Pts',(2.02841201894453,4.75264125042254,58.5343881314611));
#64507=CARTESIAN_POINT('Ctrl Pts',(-2.85835725119982,4.28517149950547,58.6920423056909));
#64508=CARTESIAN_POINT('Ctrl Pts',(-4.37651732665532,1.41635291451315,58.796776225839));
#64509=CARTESIAN_POINT('Ctrl Pts',(-4.37908572622912,-0.000563059365844233,
58.848589891905));
#64510=CARTESIAN_POINT('Origin',(0.,0.,24.1514101080949));
#64511=CARTESIAN_POINT('',(-4.37833561871486,0.00173199218209078,56.6514101080949));
#64512=CARTESIAN_POINT('',(-4.36645415447485,0.00261097933498017,56.848589891905));
#64513=CARTESIAN_POINT('',(-4.372,3.82579154166093E-12,24.1514101080949));
#64514=CARTESIAN_POINT('Ctrl Pts',(-4.37833561871486,0.00173199218209092,
56.6514101080949));
#64515=CARTESIAN_POINT('Ctrl Pts',(-4.3715252071243,-1.34959412873374,56.7008026972975));
#64516=CARTESIAN_POINT('Ctrl Pts',(-2.97623248528167,-4.16090558093235,
56.803115540582));
#64517=CARTESIAN_POINT('Ctrl Pts',(1.8094827870843,-4.8402298973603,56.9583486379485));
#64518=CARTESIAN_POINT('Ctrl Pts',(5.04785929713791,-1.10506557830443,57.1171094001944));
#64519=CARTESIAN_POINT('Ctrl Pts',(3.66628078958101,3.64148851268323,57.2758701624403));
#64520=CARTESIAN_POINT('Ctrl Pts',(-1.07078988460527,5.05524108614831,57.4346309246862));
#64521=CARTESIAN_POINT('Ctrl Pts',(-4.03315651405818,2.52188158975817,57.559810906571));
#64522=CARTESIAN_POINT('Ctrl Pts',(-4.37013967640761,0.535564934025079,
57.632070634374));
#64523=CARTESIAN_POINT('Ctrl Pts',(-4.36690348533115,0.00289237095005987,
57.6514101080949));
#64524=CARTESIAN_POINT('Ctrl Pts',(-4.36645415447485,0.00261097933498031,
56.848589891905));
#64525=CARTESIAN_POINT('Ctrl Pts',(-4.36154135054989,-0.899119064739272,
56.881320097604));
#64526=CARTESIAN_POINT('Ctrl Pts',(-3.65007828630307,-3.26593148213623,
56.9669705573851));
#64527=CARTESIAN_POINT('Ctrl Pts',(0.225623900899773,-5.162474990657,57.1055412712481));
#64528=CARTESIAN_POINT('Ctrl Pts',(4.45952627223033,-2.61049412968195,57.2643020334939));
#64529=CARTESIAN_POINT('Ctrl Pts',(4.61193398121205,2.33069069735948,57.4230627957398));
#64530=CARTESIAN_POINT('Ctrl Pts',(0.543358837230748,5.13875620630321,57.5818235579857));
#64531=CARTESIAN_POINT('Ctrl Pts',(-3.53595095853239,3.44562506237492,57.7236659233741));
#64532=CARTESIAN_POINT('Ctrl Pts',(-4.36088515262005,0.98720087478414,57.8125880346805));
#64533=CARTESIAN_POINT('Ctrl Pts',(-4.36842637263245,-0.00353866609716848,
57.848589891905));
#64534=CARTESIAN_POINT('Origin',(0.,0.,24.1514101080949));
#64535=CARTESIAN_POINT('',(-4.37203889039062,-0.00399078471529107,55.6514101080949));
#64536=CARTESIAN_POINT('',(-4.37792086111113,0.00210556704416318,55.848589891905));
#64537=CARTESIAN_POINT('',(-4.372,3.82579154166093E-12,24.1514101080949));
#64538=CARTESIAN_POINT('Ctrl Pts',(-4.37203889039062,-0.0039907847152907,
55.6514101080949));
#64539=CARTESIAN_POINT('Ctrl Pts',(-4.37513795036318,-0.341330640933386,
55.6636942520571));
#64540=CARTESIAN_POINT('Ctrl Pts',(-4.18538392269166,-2.12848606629693,
55.7288986501012));
#64541=CARTESIAN_POINT('Ctrl Pts',(-1.7316503614075,-4.86861791907028,55.8470233022273));
#64542=CARTESIAN_POINT('Ctrl Pts',(3.15105239533607,-4.09547582313724,56.0057840644731));
#64543=CARTESIAN_POINT('Ctrl Pts',(5.14981574971942,0.425970844068908,56.1645448267191));
#64544=CARTESIAN_POINT('Ctrl Pts',(2.43531042678924,4.55755598333432,56.3233055889649));
#64545=CARTESIAN_POINT('Ctrl Pts',(-2.50806538626398,4.517926674292,56.4820663512109));
#64546=CARTESIAN_POINT('Ctrl Pts',(-4.33218063910257,1.64211842271798,56.5914345242541));
#64547=CARTESIAN_POINT('Ctrl Pts',(-4.37882202467515,0.0982449665847532,
56.6478824432155));
#64548=CARTESIAN_POINT('Ctrl Pts',(-4.37833561871486,0.00173199218209092,
56.6514101080949));
#64549=CARTESIAN_POINT('Ctrl Pts',(-4.37792086111113,0.00210556704416347,
55.848589891905));
#64550=CARTESIAN_POINT('Ctrl Pts',(-4.37002924341455,-1.32628327647185,
55.8971319064456));
#64551=CARTESIAN_POINT('Ctrl Pts',(-3.01639925320847,-4.11679727890053,
55.9985941750683));
#64552=CARTESIAN_POINT('Ctrl Pts',(1.73165038597632,-4.86861798815274,56.1529766977727));
#64553=CARTESIAN_POINT('Ctrl Pts',(5.02949388480597,-1.18585219842773,56.3117374600186));
#64554=CARTESIAN_POINT('Ctrl Pts',(3.72419095237009,3.58224174562538,56.4704982222645));
#64555=CARTESIAN_POINT('Ctrl Pts',(-0.989605296568694,5.07175862308326,
56.6292589845104));
#64556=CARTESIAN_POINT('Ctrl Pts',(-4.01260884555851,2.56932936205486,56.7552895410572));
#64557=CARTESIAN_POINT('Ctrl Pts',(-4.36948468076768,0.558854755667328,
56.8283998435221));
#64558=CARTESIAN_POINT('Ctrl Pts',(-4.36645415447485,0.00261097933498031,
56.848589891905));
#64559=CARTESIAN_POINT('Origin',(0.,0.,24.1514101080949));
#64560=CARTESIAN_POINT('',(-4.36494997391578,0.000736207605459677,54.651410108095));
#64561=CARTESIAN_POINT('',(-4.37274842293649,-0.00394778047225652,54.848589891905));
#64562=CARTESIAN_POINT('',(-4.372,3.82579154166093E-12,24.1514101080949));
#64563=CARTESIAN_POINT('Ctrl Pts',(-4.36494997391578,0.000736207605459838,
54.651410108095));
#64564=CARTESIAN_POINT('Ctrl Pts',(-4.36378453680234,-0.773985575709198,
54.6795060608986));
#64565=CARTESIAN_POINT('Ctrl Pts',(-3.79750074957444,-3.0095293451424,54.7605222677843));
#64566=CARTESIAN_POINT('Ctrl Pts',(-0.22562389770033,-5.16247491740555,
54.8944587287519));
#64567=CARTESIAN_POINT('Ctrl Pts',(4.21477629650059,-2.98960100791253,55.0532194909978));
#64568=CARTESIAN_POINT('Ctrl Pts',(4.79768448212587,1.91944706257383,55.2119802532437));
#64569=CARTESIAN_POINT('Ctrl Pts',(0.989605282528937,5.07175855111871,55.3707410154895));
#64570=CARTESIAN_POINT('Ctrl Pts',(-3.35946002969715,3.69749334286384,55.5172176337734));
#64571=CARTESIAN_POINT('Ctrl Pts',(-4.36178715915881,1.11193390546508,55.6107739979751));
#64572=CARTESIAN_POINT('Ctrl Pts',(-4.37203889039062,-0.0039907847152907,
55.6514101080949));
#64573=CARTESIAN_POINT('Ctrl Pts',(-4.37274842293649,-0.00394778047225635,
54.848589891905));
#64574=CARTESIAN_POINT('Ctrl Pts',(-4.37564665776889,-0.317799192266558,
54.8600234612052));
#64575=CARTESIAN_POINT('Ctrl Pts',(-4.20162062889501,-2.08112280559727,
54.9243772845874));
#64576=CARTESIAN_POINT('Ctrl Pts',(-1.80948281276126,-4.84022996603858,
55.0416513620516));
#64577=CARTESIAN_POINT('Ctrl Pts',(3.08498768485217,-4.1454680264268,55.2004121242973));
#64578=CARTESIAN_POINT('Ctrl Pts',(5.15598322111311,0.34335287594041,55.3591728865433));
#64579=CARTESIAN_POINT('Ctrl Pts',(2.50806542185317,4.51792673839683,55.5179336487891));
#64580=CARTESIAN_POINT('Ctrl Pts',(-2.43531046134262,4.55755604800332,55.6766944110351));
#64581=CARTESIAN_POINT('Ctrl Pts',(-4.31984022389642,1.68922674479917,55.7869131587403));
#64582=CARTESIAN_POINT('Ctrl Pts',(-4.37863264435646,0.121919394632788,
55.8442116523636));
#64583=CARTESIAN_POINT('Ctrl Pts',(-4.37792086111113,0.00210556704416347,
55.848589891905));
#64584=CARTESIAN_POINT('Origin',(0.,0.,24.1514101080949));
#64585=CARTESIAN_POINT('',(-4.37473956626258,0.00360433591460132,53.6514101080949));
#64586=CARTESIAN_POINT('',(-4.36486283016371,0.00035491530368581,53.848589891905));
#64587=CARTESIAN_POINT('',(-4.372,3.82579154166093E-12,24.1514101080949));
#64588=CARTESIAN_POINT('Ctrl Pts',(-4.37473956626258,0.00360433591460166,
53.6514101080949));
#64589=CARTESIAN_POINT('Ctrl Pts',(-4.36404265119134,-1.20025020685171,
53.6953178697402));
#64590=CARTESIAN_POINT('Ctrl Pts',(-3.22404333927935,-3.87285840602707,
53.7921458854674));
#64591=CARTESIAN_POINT('Ctrl Pts',(1.30029707219943,-5.00112796677752,53.9418941552766));
#64592=CARTESIAN_POINT('Ctrl Pts',(4.90686007449561,-1.62011654684958,54.1006549175225));
#64593=CARTESIAN_POINT('Ctrl Pts',(4.02251485462088,3.2436750238594,54.2594156797684));
#64594=CARTESIAN_POINT('Ctrl Pts',(-0.543358829519001,5.13875613338857,
54.4181764420142));
#64595=CARTESIAN_POINT('Ctrl Pts',(-3.89191662696183,2.82763508414209,54.5488412514565));
#64596=CARTESIAN_POINT('Ctrl Pts',(-4.3659797009454,0.685245008222085,54.6265858068167));
#64597=CARTESIAN_POINT('Ctrl Pts',(-4.36494997391578,0.000736207605459838,
54.651410108095));
#64598=CARTESIAN_POINT('Ctrl Pts',(-4.36486283016371,0.000354915303685741,
53.848589891905));
#64599=CARTESIAN_POINT('Ctrl Pts',(-4.36431860610875,-0.750950458311704,
53.8758352700467));
#64600=CARTESIAN_POINT('Ctrl Pts',(-3.82280092431587,-2.96229440941745,
53.9560009022705));
#64601=CARTESIAN_POINT('Ctrl Pts',(-0.308361083986154,-5.15819422043212,
54.0890867885761));
#64602=CARTESIAN_POINT('Ctrl Pts',(4.16630456733569,-3.05678923480409,54.2478475508221));
#64603=CARTESIAN_POINT('Ctrl Pts',(4.82784101720183,1.84228262935957,54.4066083130679));
#64604=CARTESIAN_POINT('Ctrl Pts',(1.07078989980086,5.0552411578777,54.5653690753139));
#64605=CARTESIAN_POINT('Ctrl Pts',(-3.3251283689399,3.74330363517374,54.7126962682595));
#64606=CARTESIAN_POINT('Ctrl Pts',(-4.36223218327779,1.13486147913407,54.8071032071232));
#64607=CARTESIAN_POINT('Ctrl Pts',(-4.37274842293649,-0.00394778047225635,
54.848589891905));
#64608=CARTESIAN_POINT('Origin',(0.,0.,24.1514101080949));
#64609=CARTESIAN_POINT('',(-4.37641405919053,-0.00301495007056918,52.6514101080949));
#64610=CARTESIAN_POINT('',(-4.37405090679819,0.00376197565890995,52.848589891905));
#64611=CARTESIAN_POINT('',(-4.372,3.82579154166093E-12,24.1514101080949));
#64612=CARTESIAN_POINT('Ctrl Pts',(-4.37641405919053,-0.00301495007056837,
52.651410108095));
#64613=CARTESIAN_POINT('Ctrl Pts',(-4.37788112208874,-0.189251796122769,
52.6582094244998));
#64614=CARTESIAN_POINT('Ctrl Pts',(-4.28250642368832,-1.82348881026957,
52.7179289949866));
#64615=CARTESIAN_POINT('Ctrl Pts',(-2.22485744252472,-4.66391067415503,
52.8305688195554));
#64616=CARTESIAN_POINT('Ctrl Pts',(2.71156366187259,-4.39880391966578,52.9893295818012));
#64617=CARTESIAN_POINT('Ctrl Pts',(5.16627887713359,-0.107777454683187,
53.1480903440472));
#64618=CARTESIAN_POINT('Ctrl Pts',(2.89265785799892,4.28189022893068,53.306851106293));
#64619=CARTESIAN_POINT('Ctrl Pts',(-2.02841199016113,4.75264118298715,53.4656118685389));
#64620=CARTESIAN_POINT('Ctrl Pts',(-4.24545291415805,1.94643078465362,53.5804648691395));
#64621=CARTESIAN_POINT('Ctrl Pts',(-4.37693521146432,0.250707115811383,
53.6423976156582));
#64622=CARTESIAN_POINT('Ctrl Pts',(-4.37473956626258,0.00360433591460166,
53.6514101080949));
#64623=CARTESIAN_POINT('Ctrl Pts',(-4.37405090679819,0.00376197565890985,
52.848589891905));
#64624=CARTESIAN_POINT('Ctrl Pts',(-4.36331136726339,-1.17725226132736,
52.8916470788883));
#64625=CARTESIAN_POINT('Ctrl Pts',(-3.26012737634599,-3.8274917595608,52.9876245199536));
#64626=CARTESIAN_POINT('Ctrl Pts',(1.21995054602492,-5.021331978576,53.1365222151008));
#64627=CARTESIAN_POINT('Ctrl Pts',(4.88025534693686,-1.69857643999627,53.2952829773467));
#64628=CARTESIAN_POINT('Ctrl Pts',(4.07400138499168,3.17876814016096,53.4540437395925));
#64629=CARTESIAN_POINT('Ctrl Pts',(-0.460903086490536,5.14680702170578,
53.6128045018385));
#64630=CARTESIAN_POINT('Ctrl Pts',(-3.86811921206171,2.87497489714133,53.7443198859426));
#64631=CARTESIAN_POINT('Ctrl Pts',(-4.365375683574,0.708352879597865,53.8229150159648));
#64632=CARTESIAN_POINT('Ctrl Pts',(-4.36486283016371,0.000354915303685741,
53.848589891905));
#64633=CARTESIAN_POINT('Origin',(0.,0.,24.1514101080949));
#64634=CARTESIAN_POINT('',(-4.36545824626946,-0.00168887658937792,51.651410108095));
#64635=CARTESIAN_POINT('',(-4.37699111974124,-0.00272425946348631,51.848589891905));
#64636=CARTESIAN_POINT('',(-4.372,3.82579154166093E-12,24.1514101080949));
#64637=CARTESIAN_POINT('Ctrl Pts',(-4.36545824626946,-0.00168887658937779,
51.651410108095));
#64638=CARTESIAN_POINT('Ctrl Pts',(-4.36762412827266,-0.624989998325019,
51.6740212333413));
#64639=CARTESIAN_POINT('Ctrl Pts',(-3.95142248851676,-2.70433810681889,
51.7495526126697));
#64640=CARTESIAN_POINT('Ctrl Pts',(-0.757199377814005,-5.111624254412,51.87800424608));
#64641=CARTESIAN_POINT('Ctrl Pts',(3.88373669535471,-3.40861301664037,52.0367650083259));
#64642=CARTESIAN_POINT('Ctrl Pts',(4.97015831465276,1.41406497140078,52.1955257705718));
#64643=CARTESIAN_POINT('Ctrl Pts',(1.50773922891819,4.94254750443899,52.3542865328176));
#64644=CARTESIAN_POINT('Ctrl Pts',(-3.12722350039883,3.99007665346195,52.5062479786588));
#64645=CARTESIAN_POINT('Ctrl Pts',(-4.36646271813384,1.26026174695854,52.6052891704178));
#64646=CARTESIAN_POINT('Ctrl Pts',(-4.37641405919053,-0.00301495007056837,
52.651410108095));
#64647=CARTESIAN_POINT('Ctrl Pts',(-4.37699111974124,-0.00272425946348602,
51.848589891905));
#64648=CARTESIAN_POINT('Ctrl Pts',(-4.37818018489292,-0.165607164620367,
51.8545386336479));
#64649=CARTESIAN_POINT('Ctrl Pts',(-4.29599872620153,-1.77629134844302,
51.9134076294728));
#64650=CARTESIAN_POINT('Ctrl Pts',(-2.2993445899923,-4.62764180012773,52.0251968793796));
#64651=CARTESIAN_POINT('Ctrl Pts',(2.64069239313623,-4.44171114083851,52.1839576416255));
#64652=CARTESIAN_POINT('Ctrl Pts',(5.16388703706709,-0.190590771620509,
52.3427184038713));
#64653=CARTESIAN_POINT('Ctrl Pts',(2.96093453169081,4.23496409345547,52.5014791661172));
#64654=CARTESIAN_POINT('Ctrl Pts',(-1.95195570001178,4.78455046153847,52.6602399283632));
#64655=CARTESIAN_POINT('Ctrl Pts',(-4.23045159262607,1.99372864599193,52.7759435036257));
#64656=CARTESIAN_POINT('Ctrl Pts',(-4.37651100246309,0.274295735060812,
52.8387268248063));
#64657=CARTESIAN_POINT('Ctrl Pts',(-4.37405090679819,0.00376197565890985,
52.848589891905));
#64658=CARTESIAN_POINT('Origin',(0.,0.,24.1514101080949));
#64659=CARTESIAN_POINT('',(-4.3702345064702,0.00391522497022664,50.651410108095));
#64660=CARTESIAN_POINT('',(-4.36575804463348,-0.0020306512688445,50.848589891905));
#64661=CARTESIAN_POINT('',(-4.372,3.82579154166093E-12,24.1514101080949));
#64662=CARTESIAN_POINT('Ctrl Pts',(-4.3702345064702,0.00391522497022637,
50.651410108095));
#64663=CARTESIAN_POINT('Ctrl Pts',(-4.36105392339508,-1.0523431449496,50.6898330421829));
#64664=CARTESIAN_POINT('Ctrl Pts',(-3.44595349118066,-3.57765592823792,
50.7811762303528));
#64665=CARTESIAN_POINT('Ctrl Pts',(0.777225141445664,-5.10861766973804,
50.9254396726047));
#64666=CARTESIAN_POINT('Ctrl Pts',(4.71345919711634,-2.11786586288516,51.0842004348506));
#64667=CARTESIAN_POINT('Ctrl Pts',(4.33579142110028,2.81122147273531,51.2429611970965));
#64668=CARTESIAN_POINT('Ctrl Pts',(-0.0101251019801382,5.16739304663044,
51.4017219593423));
#64669=CARTESIAN_POINT('Ctrl Pts',(-3.72913776533524,3.13220382459871,51.5378715963418));
#64670=CARTESIAN_POINT('Ctrl Pts',(-4.36255498533209,0.833816380056773,
51.6211009792594));
#64671=CARTESIAN_POINT('Ctrl Pts',(-4.36545824626946,-0.00168887658937779,
51.651410108095));
#64672=CARTESIAN_POINT('Ctrl Pts',(-4.36575804463348,-0.00203065126884408,
50.848589891905));
#64673=CARTESIAN_POINT('Ctrl Pts',(-4.36827427270984,-0.601781773597835,
50.8703504424894));
#64674=CARTESIAN_POINT('Ctrl Pts',(-3.97337829241374,-2.65691780935309,
50.9450312471558));
#64675=CARTESIAN_POINT('Ctrl Pts',(-0.839052999411725,-5.09882773174331,
51.0726323059043));
#64676=CARTESIAN_POINT('Ctrl Pts',(3.82858979556074,-3.47044008032763,51.2313930681501));
#64677=CARTESIAN_POINT('Ctrl Pts',(4.99219026383802,1.33420033857639,51.390153830396));
#64678=CARTESIAN_POINT('Ctrl Pts',(1.58678571421362,4.91773985393535,51.548914592642));
#64679=CARTESIAN_POINT('Ctrl Pts',(-3.08887708143298,4.03478571508497,51.7017266131449));
#64680=CARTESIAN_POINT('Ctrl Pts',(-4.36760221182464,1.28340593748707,51.8016183795659));
#64681=CARTESIAN_POINT('Ctrl Pts',(-4.37699111974124,-0.00272425946348602,
51.848589891905));
#64682=CARTESIAN_POINT('Origin',(0.,0.,24.1514101080949));
#64683=CARTESIAN_POINT('',(-4.3790496246733,-0.000667733410364872,49.651410108095));
#64684=CARTESIAN_POINT('',(-4.36957357182231,0.00381643768188569,49.848589891905));
#64685=CARTESIAN_POINT('',(-4.372,3.82579154166093E-12,24.1514101080949));
#64686=CARTESIAN_POINT('Ctrl Pts',(-4.3790496246733,-0.000667733410364751,
49.651410108095));
#64687=CARTESIAN_POINT('Ctrl Pts',(-4.37912616480055,-0.0366150338825652,
49.6527245969425));
#64688=CARTESIAN_POINT('Ctrl Pts',(-4.36244279655587,-1.51969860268292,
49.706959339872));
#64689=CARTESIAN_POINT('Ctrl Pts',(-2.69430468338317,-4.40939629531691,
49.8141143368835));
#64690=CARTESIAN_POINT('Ctrl Pts',(2.2431174238849,-4.6551560273227,49.9728750991294));
#64691=CARTESIAN_POINT('Ctrl Pts',(5.12756994789964,-0.640374769530455,
50.1316358613752));
#64692=CARTESIAN_POINT('Ctrl Pts',(3.31911383193326,3.96049703783808,50.2903966236212));
#64693=CARTESIAN_POINT('Ctrl Pts',(-1.52709664667054,4.93660098122003,50.4491573858669));
#64694=CARTESIAN_POINT('Ctrl Pts',(-4.14104743841719,2.25180987009099,50.569495214025));
#64695=CARTESIAN_POINT('Ctrl Pts',(-4.37369842336595,0.402451046051582,
50.636912788101));
#64696=CARTESIAN_POINT('Ctrl Pts',(-4.3702345064702,0.00391522497022637,
50.651410108095));
#64697=CARTESIAN_POINT('Ctrl Pts',(-4.36957357182231,0.00381643768188559,
49.848589891905));
#64698=CARTESIAN_POINT('Ctrl Pts',(-4.36092390126923,-1.02945575440987,
49.886162251331));
#64699=CARTESIAN_POINT('Ctrl Pts',(-3.47811671755736,-3.53137427358546,
49.976654864839));
#64700=CARTESIAN_POINT('Ctrl Pts',(0.695222531978707,-5.12042183856424,
50.1200677324289));
#64701=CARTESIAN_POINT('Ctrl Pts',(4.67889927324325,-2.19316113513354,50.2788284946747));
#64702=CARTESIAN_POINT('Ctrl Pts',(4.38030448079635,2.74134763015048,50.4375892569207));
#64703=CARTESIAN_POINT('Ctrl Pts',(0.0727212293821569,5.16689130876717,
50.5963500191666));
#64704=CARTESIAN_POINT('Ctrl Pts',(-3.70187703653703,3.1792474229629,50.733350230828));
#64705=CARTESIAN_POINT('Ctrl Pts',(-4.36215496848489,0.85677423381658,50.8174301884075));
#64706=CARTESIAN_POINT('Ctrl Pts',(-4.36575804463348,-0.00203065126884408,
50.848589891905));
#64707=CARTESIAN_POINT('Origin',(0.,0.,24.1514101080949));
#64708=CARTESIAN_POINT('',(-4.36828286829859,-0.0034930826256922,48.651410108095));
#64709=CARTESIAN_POINT('',(-4.37915940465982,-0.00023684953408154,48.848589891905));
#64710=CARTESIAN_POINT('',(-4.372,3.82579154166093E-12,24.1514101080949));
#64711=CARTESIAN_POINT('Ctrl Pts',(-4.36828286829859,-0.00349308262569223,
48.651410108095));
#64712=CARTESIAN_POINT('Ctrl Pts',(-4.37181608551705,-0.47483281190334,
48.6685364057841));
#64713=CARTESIAN_POINT('Ctrl Pts',(-4.08436231910608,-2.39841849396994,
48.7385829575551));
#64714=CARTESIAN_POINT('Ctrl Pts',(-1.2806885257803,-5.00618520592171,48.8615497634081));
#64715=CARTESIAN_POINT('Ctrl Pts',(3.51122164426531,-3.79122354667958,49.020310525654));
#64716=CARTESIAN_POINT('Ctrl Pts',(5.0895545138177,0.893581706914796,49.1790712878999));
#64717=CARTESIAN_POINT('Ctrl Pts',(2.00977162985725,4.76055368753214,49.3378320501457));
#64718=CARTESIAN_POINT('Ctrl Pts',(-2.86868632585708,4.274578831514,49.4952783235442));
#64719=CARTESIAN_POINT('Ctrl Pts',(-4.37604472140215,1.41059410609646,49.5998043428605));
#64720=CARTESIAN_POINT('Ctrl Pts',(-4.3790496246733,-0.000667733410364751,
49.651410108095));
#64721=CARTESIAN_POINT('Ctrl Pts',(-4.37915940465982,-0.000236849534081855,
48.848589891905));
#64722=CARTESIAN_POINT('Ctrl Pts',(-4.37916937864932,-0.0129226461636581,
48.8490538060906));
#64723=CARTESIAN_POINT('Ctrl Pts',(-4.37337449519616,-1.47271062880396,
48.9024379743582));
#64724=CARTESIAN_POINT('Ctrl Pts',(-2.76465105904324,-4.36563382517906,
49.0087423967076));
#64725=CARTESIAN_POINT('Ctrl Pts',(2.16819644989342,-4.69052004883103,49.1675031589536));
#64726=CARTESIAN_POINT('Ctrl Pts',(5.11664433946473,-0.72249904999246,49.3262639211995));
#64727=CARTESIAN_POINT('Ctrl Pts',(3.38218303962157,3.90677514842007,49.4850246834453));
#64728=CARTESIAN_POINT('Ctrl Pts',(-1.44775548820939,4.96044939699782,49.6437854456913));
#64729=CARTESIAN_POINT('Ctrl Pts',(-4.12319150304179,2.29923281750856,49.7649738485111));
#64730=CARTESIAN_POINT('Ctrl Pts',(-4.37310686689576,0.425896738132308,
49.833241997249));
#64731=CARTESIAN_POINT('Ctrl Pts',(-4.36957357182231,0.00381643768188559,
49.848589891905));
#64732=CARTESIAN_POINT('Origin',(0.,0.,24.1514101080949));
#64733=CARTESIAN_POINT('',(-4.36655943089002,0.00268207779483023,47.651410108095));
#64734=CARTESIAN_POINT('',(-4.36888289277856,-0.00366680700230215,47.848589891905));
#64735=CARTESIAN_POINT('',(-4.372,3.82579154166093E-12,24.1514101080949));
#64736=CARTESIAN_POINT('Ctrl Pts',(-4.36655943089002,0.00268207779483047,
47.651410108095));
#64737=CARTESIAN_POINT('Ctrl Pts',(-4.36147330371707,-0.90472081724388,
47.6843482146256));
#64738=CARTESIAN_POINT('Ctrl Pts',(-3.64307749349284,-3.2773877690834,47.7702065752383));
#64739=CARTESIAN_POINT('Ctrl Pts',(0.245853018125491,-5.16155109531365,
47.9089851899327));
#64740=CARTESIAN_POINT('Ctrl Pts',(4.46972204405066,-2.59299792999961,48.0677459521787));
#64741=CARTESIAN_POINT('Ctrl Pts',(4.60276492582317,2.34874614500311,48.2265067144246));
#64742=CARTESIAN_POINT('Ctrl Pts',(0.523216754197009,5.14084600471386,48.3852674766704));
#64743=CARTESIAN_POINT('Ctrl Pts',(-3.54345722553092,3.4342468351364,48.5269019412272));
#64744=CARTESIAN_POINT('Ctrl Pts',(-4.36089844550389,0.981606792564894,
48.6156161517021));
#64745=CARTESIAN_POINT('Ctrl Pts',(-4.36828286829859,-0.00349308262569223,
48.651410108095));
#64746=CARTESIAN_POINT('Ctrl Pts',(-4.36888289277856,-0.00366680700230278,
47.848589891905));
#64747=CARTESIAN_POINT('Ctrl Pts',(-4.37244155465394,-0.451442255901039,
47.8648656149322));
#64748=CARTESIAN_POINT('Ctrl Pts',(-4.10318789366455,-2.35097548418382,
47.9340615920413));
#64749=CARTESIAN_POINT('Ctrl Pts',(-1.36078444624568,-4.98500951500319,
48.0561778232324));
#64750=CARTESIAN_POINT('Ctrl Pts',(3.44998850215064,-3.84702917961962,48.2149385854782));
#64751=CARTESIAN_POINT('Ctrl Pts',(5.10322659210776,0.811869769988193,48.3736993477241));
#64752=CARTESIAN_POINT('Ctrl Pts',(2.08583582488191,4.72772070721777,48.53246010997));
#64753=CARTESIAN_POINT('Ctrl Pts',(-2.82618015492052,4.31781852687336,48.6907569580302));
#64754=CARTESIAN_POINT('Ctrl Pts',(-4.37803161206443,1.43418891395024,48.7961335520086));
#64755=CARTESIAN_POINT('Ctrl Pts',(-4.37915940465982,-0.000236849534081855,
48.848589891905));
#64756=CARTESIAN_POINT('Origin',(0.,0.,24.1514101080949));
#64757=CARTESIAN_POINT('',(-4.37802849378088,0.00201652107500087,46.651410108095));
#64758=CARTESIAN_POINT('',(-4.36614763918315,0.00238232933584437,46.848589891905));
#64759=CARTESIAN_POINT('',(-4.372,3.82579154166093E-12,24.1514101080949));
#64760=CARTESIAN_POINT('Ctrl Pts',(-4.37802849378088,0.00201652107500106,
46.651410108095));
#64761=CARTESIAN_POINT('Ctrl Pts',(-4.37038284048536,-1.33197484216078,
46.7001600234672));
#64762=CARTESIAN_POINT('Ctrl Pts',(-3.00664095593531,-4.12759897737828,
46.8018301929213));
#64763=CARTESIAN_POINT('Ctrl Pts',(1.75071634247466,-4.86179449424254,46.9564206164574));
#64764=CARTESIAN_POINT('Ctrl Pts',(5.03410234489664,-1.16613335307792,47.1151813787034));
#64765=CARTESIAN_POINT('Ctrl Pts',(3.71012411261097,3.59680865283067,47.2739421409492));
#64766=CARTESIAN_POINT('Ctrl Pts',(-1.00947303475291,5.06784151371782,47.4327029031951));
#64767=CARTESIAN_POINT('Ctrl Pts',(-4.01767618670528,2.55773240591479,47.5585255589103));
#64768=CARTESIAN_POINT('Ctrl Pts',(-4.36964496780575,0.553164799693178,
47.6314279605436));
#64769=CARTESIAN_POINT('Ctrl Pts',(-4.36655943089002,0.00268207779483047,
47.651410108095));
#64770=CARTESIAN_POINT('Ctrl Pts',(-4.36614763918315,0.00238232933584499,
46.848589891905));
#64771=CARTESIAN_POINT('Ctrl Pts',(-4.36177165814571,-0.881797305075611,
46.8806774237737));
#64772=CARTESIAN_POINT('Ctrl Pts',(-3.67150621186276,-3.23048848803606,
46.9656852097244));
#64773=CARTESIAN_POINT('Ctrl Pts',(0.163070052891163,-5.16482936133098,
47.103613249757));
#64774=CARTESIAN_POINT('Ctrl Pts',(4.42757599841828,-2.66432448325026,47.2623740120029));
#64775=CARTESIAN_POINT('Ctrl Pts',(4.63982914812316,2.27465154475207,47.4211347742487));
#64776=CARTESIAN_POINT('Ctrl Pts',(0.605568936039063,5.13179699886122,47.5798955364947));
#64777=CARTESIAN_POINT('Ctrl Pts',(-3.51252635231322,3.4807591641629,47.7223805757134));
#64778=CARTESIAN_POINT('Ctrl Pts',(-4.36087062227061,1.00449248124495,47.8119453608502));
#64779=CARTESIAN_POINT('Ctrl Pts',(-4.36888289277856,-0.00366680700230278,
47.848589891905));
#64780=CARTESIAN_POINT('Origin',(0.,0.,24.1514101080949));
#64781=CARTESIAN_POINT('',(-4.37257478030532,-0.00396203305634906,45.651410108095));
#64782=CARTESIAN_POINT('',(-4.37756404870526,0.00237073416934012,45.848589891905));
#64783=CARTESIAN_POINT('',(-4.372,3.82579154166093E-12,24.1514101080949));
#64784=CARTESIAN_POINT('Ctrl Pts',(-4.37257478030532,-0.00396203305634935,
45.651410108095));
#64785=CARTESIAN_POINT('Ctrl Pts',(-4.3755247754399,-0.323552849206446,
45.6630515782267));
#64786=CARTESIAN_POINT('Ctrl Pts',(-4.19769260696374,-2.0926975991144,45.7276133024405));
#64787=CARTESIAN_POINT('Ctrl Pts',(-1.79050086272392,-4.84728378338218,
45.8450952807362));
#64788=CARTESIAN_POINT('Ctrl Pts',(3.1012093298518,-4.13334659912459,46.0038560429821));
#64789=CARTESIAN_POINT('Ctrl Pts',(5.15459801607478,0.363555647367575,46.162616805228));
#64790=CARTESIAN_POINT('Ctrl Pts',(2.49034114873962,4.52772066043712,46.3213775674739));
#64791=CARTESIAN_POINT('Ctrl Pts',(-2.45315200638293,4.54797742404625,46.4801383297198));
#64792=CARTESIAN_POINT('Ctrl Pts',(-4.32289330486948,1.67770933141668,46.5901491765935));
#64793=CARTESIAN_POINT('Ctrl Pts',(-4.37868254545781,0.116133556522668,
46.6472397693852));
#64794=CARTESIAN_POINT('Ctrl Pts',(-4.37802849378088,0.00201652107500106,
46.651410108095));
#64795=CARTESIAN_POINT('Ctrl Pts',(-4.37756404870526,0.00237073416934035,
45.848589891905));
#64796=CARTESIAN_POINT('Ctrl Pts',(-4.36898434288233,-1.30871296070451,
45.8964892326153));
#64797=CARTESIAN_POINT('Ctrl Pts',(-3.04632193268225,-4.08332402648612,
45.9973088274075));
#64798=CARTESIAN_POINT('Ctrl Pts',(1.67254576409749,-4.88923765436041,46.1510486762816));
#64799=CARTESIAN_POINT('Ctrl Pts',(5.01475964555148,-1.2466915701828,46.3098094385276));
#64800=CARTESIAN_POINT('Ctrl Pts',(3.76731232156889,3.53686471971598,46.4685702007735));
#64801=CARTESIAN_POINT('Ctrl Pts',(-0.928094313166731,5.08337438319113,
46.6273309630193));
#64802=CARTESIAN_POINT('Ctrl Pts',(-3.99675882839479,2.60517577302872,46.7540041933965));
#64803=CARTESIAN_POINT('Ctrl Pts',(-4.36898873016318,0.576432985076398,
46.8277571696918));
#64804=CARTESIAN_POINT('Ctrl Pts',(-4.36614763918315,0.00238232933584499,
46.848589891905));
#64805=CARTESIAN_POINT('Origin',(0.,0.,24.1514101080949));
#64806=CARTESIAN_POINT('',(-4.36487844624636,0.000448538275869127,44.651410108095));
#64807=CARTESIAN_POINT('',(-4.37328422903404,-0.00388840045026428,44.848589891905));
#64808=CARTESIAN_POINT('',(-4.372,3.82579154166093E-12,24.1514101080949));
#64809=CARTESIAN_POINT('Ctrl Pts',(-4.36487844624636,0.00044853827586927,
44.651410108095));
#64810=CARTESIAN_POINT('Ctrl Pts',(-4.36418527448618,-0.756583014477848,
44.6788633870683));
#64811=CARTESIAN_POINT('Ctrl Pts',(-3.8166662948363,-2.9738437257919,44.7592369201236));
#64812=CARTESIAN_POINT('Ctrl Pts',(-0.288144634510089,-5.15936295347187,
44.8925307072609));
#64813=CARTESIAN_POINT('Ctrl Pts',(4.17825154873217,-3.04043868735616,45.0512914695067));
#64814=CARTESIAN_POINT('Ctrl Pts',(4.8205842882194,1.86118793683688,45.2100522317526));
#64815=CARTESIAN_POINT('Ctrl Pts',(1.05097104046387,5.05939851051103,45.3688129939986));
#64816=CARTESIAN_POINT('Ctrl Pts',(-3.33357615425217,3.73211986818334,45.5159322861126));
#64817=CARTESIAN_POINT('Ctrl Pts',(-4.36211457120495,1.12925568798617,45.6101313241448));
#64818=CARTESIAN_POINT('Ctrl Pts',(-4.37257478030532,-0.00396203305634935,
45.651410108095));
#64819=CARTESIAN_POINT('Ctrl Pts',(-4.37328422903404,-0.00388840045026397,
44.848589891905));
#64820=CARTESIAN_POINT('Ctrl Pts',(-4.37601255181714,-0.300005218706897,
44.8593807873749));
#64821=CARTESIAN_POINT('Ctrl Pts',(-4.21359764945945,-2.04535030654532,
44.9230919369267));
#64822=CARTESIAN_POINT('Ctrl Pts',(-1.8679837165673,-4.81795506501003,45.0397233405604));
#64823=CARTESIAN_POINT('Ctrl Pts',(3.03454387031403,-4.18253483822383,45.1984841028063));
#64824=CARTESIAN_POINT('Ctrl Pts',(5.15976421573454,0.280869029694986,45.3572448650522));
#64825=CARTESIAN_POINT('Ctrl Pts',(2.56261074386464,4.4872129823807,45.5160056272982));
#64826=CARTESIAN_POINT('Ctrl Pts',(-2.37992235675453,4.58672254988638,45.6747663895439));
#64827=CARTESIAN_POINT('Ctrl Pts',(-4.31025055648257,1.72484198053187,45.7856278110796));
#64828=CARTESIAN_POINT('Ctrl Pts',(-4.37846339218375,0.139801386813307,
45.8435689785333));
#64829=CARTESIAN_POINT('Ctrl Pts',(-4.37756404870526,0.00237073416934035,
45.848589891905));
#64830=CARTESIAN_POINT('Origin',(0.,0.,24.1514101080949));
#64831=CARTESIAN_POINT('',(-4.37422072754471,0.00372710199133062,43.651410108095));
#64832=CARTESIAN_POINT('',(-4.36483752583336,6.45211600033835E-5,43.848589891905));
#64833=CARTESIAN_POINT('',(-4.372,3.82579154166093E-12,24.1514101080949));
#64834=CARTESIAN_POINT('Ctrl Pts',(-4.37422072754471,0.00372710199133028,
43.651410108095));
#64835=CARTESIAN_POINT('Ctrl Pts',(-4.36348027804383,-1.18287063932153,
43.6946751959099));
#64836=CARTESIAN_POINT('Ctrl Pts',(-3.25136487986307,-3.83859580238497,
43.7908605378067));
#64837=CARTESIAN_POINT('Ctrl Pts',(1.23961889884326,-5.01651257365967,43.9399661337855));
#64838=CARTESIAN_POINT('Ctrl Pts',(4.88687423334376,-1.67943849054845,44.0987268960314));
#64839=CARTESIAN_POINT('Ctrl Pts',(4.06151299797099,3.19470899822934,44.2574876582773));
#64840=CARTESIAN_POINT('Ctrl Pts',(-0.481068993674721,5.1449612281707,44.4162484205232));
#64841=CARTESIAN_POINT('Ctrl Pts',(-3.87398394218857,2.8634067002645,44.5475559037957));
#64842=CARTESIAN_POINT('Ctrl Pts',(-4.36552146553668,0.702707227634927,
44.6259431329863));
#64843=CARTESIAN_POINT('Ctrl Pts',(-4.36487844624636,0.00044853827586927,
44.651410108095));
#64844=CARTESIAN_POINT('Ctrl Pts',(-4.36483752583336,6.45211600032447E-5,
43.848589891905));
#64845=CARTESIAN_POINT('Ctrl Pts',(-4.36474095456816,-0.733529397636361,
43.8751925962164));
#64846=CARTESIAN_POINT('Ctrl Pts',(-3.84156354313547,-2.92657717231582,
43.9547155546098));
#64847=CARTESIAN_POINT('Ctrl Pts',(-0.370823894361365,-5.15408030721166,
44.0871587670851));
#64848=CARTESIAN_POINT('Ctrl Pts',(4.12896947009338,-3.10703480650815,44.245919529331));
#64849=CARTESIAN_POINT('Ctrl Pts',(4.84980385450403,1.78366385472551,44.4046802915768));
#64850=CARTESIAN_POINT('Ctrl Pts',(1.13194961208497,5.04189887339256,44.5634410538228));
#64851=CARTESIAN_POINT('Ctrl Pts',(-3.29878256966109,3.77781872906067,44.7114109205989));
#64852=CARTESIAN_POINT('Ctrl Pts',(-4.36263242638615,1.15219838236422,44.8064605332929));
#64853=CARTESIAN_POINT('Ctrl Pts',(-4.37328422903404,-0.00388840045026397,
44.848589891905));
#64854=CARTESIAN_POINT('Origin',(0.,0.,24.1514101080949));
#64855=CARTESIAN_POINT('',(-4.37685426135052,-0.00279837449763291,42.651410108095));
#64856=CARTESIAN_POINT('',(-4.37352103895722,0.00385464862035001,42.848589891905));
#64857=CARTESIAN_POINT('',(-4.372,3.82579154166093E-12,24.1514101080949));
#64858=CARTESIAN_POINT('Ctrl Pts',(-4.37685426135052,-0.00279837449763325,
42.651410108095));
#64859=CARTESIAN_POINT('Ctrl Pts',(-4.37811047462212,-0.171387646022154,
42.6575667506695));
#64860=CARTESIAN_POINT('Ctrl Pts',(-4.29273874071207,-1.78782473877565,
42.7166436473259));
#64861=CARTESIAN_POINT('Ctrl Pts',(-2.28119196804685,-4.63661693705371,
42.8286407980642));
#64862=CARTESIAN_POINT('Ctrl Pts',(2.65807838191241,-4.43132855153674,42.9874015603103));
#64863=CARTESIAN_POINT('Ctrl Pts',(5.1645942046841,-0.170352918960309,43.146162322556));
#64864=CARTESIAN_POINT('Ctrl Pts',(2.94431565674484,4.24653490854626,43.304923084802));
#64865=CARTESIAN_POINT('Ctrl Pts',(-1.97069051554003,4.77686427565358,43.4636838470478));
#64866=CARTESIAN_POINT('Ctrl Pts',(-4.23415771881522,1.98216556151801,43.5791795214788));
#64867=CARTESIAN_POINT('Ctrl Pts',(-4.37661759834636,0.26853179933828,43.6417549418279));
#64868=CARTESIAN_POINT('Ctrl Pts',(-4.37422072754471,0.00372710199133028,
43.651410108095));
#64869=CARTESIAN_POINT('Ctrl Pts',(-4.37352103895722,0.00385464862035015,
42.848589891905));
#64870=CARTESIAN_POINT('Ctrl Pts',(-4.36282818723577,-1.15989502481933,
42.891004405058));
#64871=CARTESIAN_POINT('Ctrl Pts',(-3.28698059005484,-3.79310505340026,
42.9863391722929));
#64872=CARTESIAN_POINT('Ctrl Pts',(1.15903352033341,-5.0357417996319,43.1345941936098));
#64873=CARTESIAN_POINT('Ctrl Pts',(4.85932100888344,-1.75757034181863,43.2933549558556));
#64874=CARTESIAN_POINT('Ctrl Pts',(4.11220948021047,3.12918317851219,43.4521157181016));
#64875=CARTESIAN_POINT('Ctrl Pts',(-0.398521773825228,5.15201267172389,
43.6108764803474));
#64876=CARTESIAN_POINT('Ctrl Pts',(-3.84979170382512,2.91072243457703,43.7430345382819));
#64877=CARTESIAN_POINT('Ctrl Pts',(-4.36493306195062,0.725795042513237,
43.8222723421345));
#64878=CARTESIAN_POINT('Ctrl Pts',(-4.36483752583336,6.45211600032447E-5,
43.848589891905));
#64879=CARTESIAN_POINT('Origin',(0.,0.,24.1514101080949));
#64880=CARTESIAN_POINT('',(-4.36567955402809,-0.00194869704108157,41.651410108095));
#64881=CARTESIAN_POINT('',(-4.37739485101806,-0.00248321819134589,41.848589891905));
#64882=CARTESIAN_POINT('',(-4.372,3.82579154166093E-12,24.1514101080949));
#64883=CARTESIAN_POINT('Ctrl Pts',(-4.3656795540281,-0.00194869704108112,
41.651410108095));
#64884=CARTESIAN_POINT('Ctrl Pts',(-4.36811474531132,-0.607457052316279,
41.673378559511));
#64885=CARTESIAN_POINT('Ctrl Pts',(-3.96805804018506,-2.66850978845469,
41.748267265009));
#64886=CARTESIAN_POINT('Ctrl Pts',(-0.819065114488867,-5.10207661195736,
41.8760762245889));
#64887=CARTESIAN_POINT('Ctrl Pts',(3.8421604015636,-3.45540979692878,42.0348369868349));
#64888=CARTESIAN_POINT('Ctrl Pts',(4.98692335778749,1.35375361111553,42.1935977490807));
#64889=CARTESIAN_POINT('Ctrl Pts',(1.56750172940691,4.92392036332446,42.3523585113267));
#64890=CARTESIAN_POINT('Ctrl Pts',(-3.09830846639719,4.02387607629251,42.504962630998));
#64891=CARTESIAN_POINT('Ctrl Pts',(-4.36731252351321,1.27774424309386,42.6046464965875));
#64892=CARTESIAN_POINT('Ctrl Pts',(-4.37685426135052,-0.00279837449763325,
42.651410108095));
#64893=CARTESIAN_POINT('Ctrl Pts',(-4.37739485101806,-0.00248321819134518,
41.8485898919051));
#64894=CARTESIAN_POINT('Ctrl Pts',(-4.37838119777137,-0.1477338083412,41.8538959598176));
#64895=CARTESIAN_POINT('Ctrl Pts',(-4.30592187837124,-1.74065025431473,
41.9121222818121));
#64896=CARTESIAN_POINT('Ctrl Pts',(-2.35523429540729,-4.59944840035779,
42.0232688578885));
#64897=CARTESIAN_POINT('Ctrl Pts',(2.58669254300161,-4.47337410259821,42.1820296201345));
#64898=CARTESIAN_POINT('Ctrl Pts',(5.16119935450289,-0.253131185149624,
42.3407903823802));
#64899=CARTESIAN_POINT('Ctrl Pts',(3.01201886587614,4.19878512494061,42.4995511446263));
#64900=CARTESIAN_POINT('Ctrl Pts',(-1.89385329211466,4.80784503512363,42.6583119068721));
#64901=CARTESIAN_POINT('Ctrl Pts',(-4.21883224032928,2.02948215439444,42.774658155965));
#64902=CARTESIAN_POINT('Ctrl Pts',(-4.37616957413132,0.292106279171763,
42.838084150976));
#64903=CARTESIAN_POINT('Ctrl Pts',(-4.37352103895722,0.00385464862035015,
42.848589891905));
#64904=CARTESIAN_POINT('Origin',(0.,0.,24.1514101080949));
#64905=CARTESIAN_POINT('',(-4.36973282931957,0.00384403733829788,40.651410108095));
#64906=CARTESIAN_POINT('',(-4.36602112377814,-0.00227682230535847,40.848589891905));
#64907=CARTESIAN_POINT('',(-4.372,3.82579154166093E-12,24.1514101080949));
#64908=CARTESIAN_POINT('Ctrl Pts',(-4.36973282931958,0.00384403733829777,
40.651410108095));
#64909=CARTESIAN_POINT('Ctrl Pts',(-4.36094828703741,-1.03504959539527,
40.6891903683526));
#64910=CARTESIAN_POINT('Ctrl Pts',(-3.47031004267523,-3.54269738683393,
40.7798908826921));
#64911=CARTESIAN_POINT('Ctrl Pts',(0.715283237582617,-5.11765799033974,
40.9235116511136));
#64912=CARTESIAN_POINT('Ctrl Pts',(4.6874579011302,-2.17480846080452,41.0822724133595));
#64913=CARTESIAN_POINT('Ctrl Pts',(4.36952791329752,2.75849220244841,41.2410331756054));
#64914=CARTESIAN_POINT('Ctrl Pts',(0.052472510246957,5.16713654277911,41.3997939378513));
#64915=CARTESIAN_POINT('Ctrl Pts',(-3.70859131189293,3.16775466245737,41.5365862486812));
#64916=CARTESIAN_POINT('Ctrl Pts',(-4.36224856298441,0.851164468294318,
41.620458305429));
#64917=CARTESIAN_POINT('Ctrl Pts',(-4.3656795540281,-0.00194869704108112,
41.651410108095));
#64918=CARTESIAN_POINT('Ctrl Pts',(-4.36602112377814,-0.00227682230535861,
40.848589891905));
#64919=CARTESIAN_POINT('Ctrl Pts',(-4.36876880712171,-0.584227201261346,
40.8697077686591));
#64920=CARTESIAN_POINT('Ctrl Pts',(-3.98963601281,-2.62107929020566,40.9437458994952));
#64921=CARTESIAN_POINT('Ctrl Pts',(-0.90075771530386,-5.08828946819429,
41.0707042844132));
#64922=CARTESIAN_POINT('Ctrl Pts',(3.78626858625262,-3.51656428443629,41.2294650466591));
#64923=CARTESIAN_POINT('Ctrl Pts',(5.00798622459088,1.27362794729248,41.3882258089049));
#64924=CARTESIAN_POINT('Ctrl Pts',(1.64624189925253,4.89815697818699,41.5469865711509));
#64925=CARTESIAN_POINT('Ctrl Pts',(-3.0594815075565,4.0684328488748,41.7004412654842));
#64926=CARTESIAN_POINT('Ctrl Pts',(-4.36854383389695,1.30092803749072,41.8009757057356));
#64927=CARTESIAN_POINT('Ctrl Pts',(-4.37739485101806,-0.00248321819134518,
41.8485898919051));
#64928=CARTESIAN_POINT('Origin',(0.,0.,24.1514101080949));
#64929=CARTESIAN_POINT('',(-4.37914188721017,-0.000342719191574727,39.651410108095));
#64930=CARTESIAN_POINT('',(-4.36909141260198,0.00371732487008336,39.848589891905));
#64931=CARTESIAN_POINT('',(-4.372,3.82579154166093E-12,24.1514101080949));
#64932=CARTESIAN_POINT('Ctrl Pts',(-4.37914188721017,-0.000342719191574457,
39.651410108095));
#64933=CARTESIAN_POINT('Ctrl Pts',(-4.37916257714185,-0.0187137896541573,
39.6520819231122));
#64934=CARTESIAN_POINT('Ctrl Pts',(-4.37073789868075,-1.48419245149001,
39.7056739922113));
#64935=CARTESIAN_POINT('Ctrl Pts',(-2.74752162183386,-4.3764344338297,39.8121863153924));
#64936=CARTESIAN_POINT('Ctrl Pts',(2.18656111288008,-4.68198717594309,39.9709470776383));
#64937=CARTESIAN_POINT('Ctrl Pts',(5.11943632770732,-0.702442241472902,
40.1297078398842));
#64938=CARTESIAN_POINT('Ctrl Pts',(3.36684704019806,3.9199992887709,40.2884686021301));
#64939=CARTESIAN_POINT('Ctrl Pts',(-1.46718350018236,4.95473773199425,40.4472293643759));
#64940=CARTESIAN_POINT('Ctrl Pts',(-4.12759825135317,2.28764036559584,40.5682098663642));
#64941=CARTESIAN_POINT('Ctrl Pts',(-4.37325313105903,0.420168410874277,
40.6362701142706));
#64942=CARTESIAN_POINT('Ctrl Pts',(-4.36973282931958,0.00384403733829777,
40.651410108095));
#64943=CARTESIAN_POINT('Ctrl Pts',(-4.36909141260198,0.0037173248700835,
39.848589891905));
#64944=CARTESIAN_POINT('Ctrl Pts',(-4.36087746473157,-1.01216450930882,
39.8855195775007));
#64945=CARTESIAN_POINT('Ctrl Pts',(-3.50202565789313,-3.49632888214117,
39.9753695171783));
#64946=CARTESIAN_POINT('Ctrl Pts',(0.6331436514814,-5.12846792818335,40.1181397109379));
#64947=CARTESIAN_POINT('Ctrl Pts',(4.65198839971611,-2.2496795555641,40.2769004731838));
#64948=CARTESIAN_POINT('Ctrl Pts',(4.41319126769477,2.68808426366416,40.4356612354296));
#64949=CARTESIAN_POINT('Ctrl Pts',(0.135306684796697,5.16563125618407,40.5944219976755));
#64950=CARTESIAN_POINT('Ctrl Pts',(-3.68091103301737,3.21474907678104,40.7320648831673));
#64951=CARTESIAN_POINT('Ctrl Pts',(-4.36188326164895,0.874108893605594,
40.8167875145772));
#64952=CARTESIAN_POINT('Ctrl Pts',(-4.36602112377814,-0.00227682230535861,
40.848589891905));
#64953=CARTESIAN_POINT('Origin',(0.,0.,24.1514101080949));
#64954=CARTESIAN_POINT('',(-4.36873305544013,-0.00362749675167218,38.651410108095));
#64955=CARTESIAN_POINT('',(-4.37917310725098,9.13219796030052E-5,38.848589891905));
#64956=CARTESIAN_POINT('',(-4.372,3.82579154166093E-12,24.1514101080949));
#64957=CARTESIAN_POINT('Ctrl Pts',(-4.36873305544013,-0.00362749675167234,
38.651410108095));
#64958=CARTESIAN_POINT('Ctrl Pts',(-4.37228988643661,-0.457161961038693,
38.6678937319537));
#64959=CARTESIAN_POINT('Ctrl Pts',(-4.0986296928328,-2.36257101965516,38.7372976098944));
#64960=CARTESIAN_POINT('Ctrl Pts',(-1.34123858177823,-4.99030384674165,
38.8596217419171));
#64961=CARTESIAN_POINT('Ctrl Pts',(3.46503780867414,-3.83347967263602,39.0183825041629));
#64962=CARTESIAN_POINT('Ctrl Pts',(5.10000575566994,0.831862193027325,39.1771432664089));
#64963=CARTESIAN_POINT('Ctrl Pts',(2.06729265337245,4.73585837007054,39.3359040286547));
#64964=CARTESIAN_POINT('Ctrl Pts',(-2.83663011433148,4.30727362250648,39.4939929758834));
#64965=CARTESIAN_POINT('Ctrl Pts',(-4.37753278856417,1.42841330898948,39.5991616690302));
#64966=CARTESIAN_POINT('Ctrl Pts',(-4.37914188721017,-0.000342719191574457,
39.651410108095));
#64967=CARTESIAN_POINT('Ctrl Pts',(-4.37917310725098,9.13219796029981E-5,
38.848589891905));
#64968=CARTESIAN_POINT('Ctrl Pts',(-4.37872965626048,-1.44211984317019,
38.9013313863422));
#64969=CARTESIAN_POINT('Ctrl Pts',(-2.81178331229755,-4.33225607926283,
39.0069931348614));
#64970=CARTESIAN_POINT('Ctrl Pts',(2.11121724282438,-4.71644102342194,39.1655751374625));
#64971=CARTESIAN_POINT('Ctrl Pts',(5.10751668218689,-0.784428145210908,
39.3243358997084));
#64972=CARTESIAN_POINT('Ctrl Pts',(3.42926084288352,3.86551733216684,39.4830966619543));
#64973=CARTESIAN_POINT('Ctrl Pts',(-1.38755926796319,4.97762327338117,39.6418574242002));
#64974=CARTESIAN_POINT('Ctrl Pts',(-4.1093944849834,2.33507192947434,39.7636885008504));
#64975=CARTESIAN_POINT('Ctrl Pts',(-4.37264805528242,0.443594561337992,
39.8325993234187));
#64976=CARTESIAN_POINT('Ctrl Pts',(-4.36909141260198,0.0037173248700835,
39.848589891905));
#64977=CARTESIAN_POINT('Origin',(0.,0.,24.1514101080949));
#64978=CARTESIAN_POINT('',(-4.36624352627694,0.00245771687439172,37.651410108095));
#64979=CARTESIAN_POINT('',(-4.36935764006,-0.00377501215838794,37.848589891905));
#64980=CARTESIAN_POINT('',(-4.372,3.82579154166093E-12,24.1514101080949));
#64981=CARTESIAN_POINT('Ctrl Pts',(-4.36624352627694,0.00245771687439181,
37.651410108095));
#64982=CARTESIAN_POINT('Ctrl Pts',(-4.36169382655995,-0.887401680305794,
37.6837055407953));
#64983=CARTESIAN_POINT('Ctrl Pts',(-3.66460952904662,-3.24195865307006,
37.7689212275775));
#64984=CARTESIAN_POINT('Ctrl Pts',(0.183308877707052,-5.16415058566349,
37.9070571684418));
#64985=CARTESIAN_POINT('Ctrl Pts',(4.43798296793759,-2.64695307709652,38.0658179306876));
#64986=CARTESIAN_POINT('Ctrl Pts',(4.63087948595682,2.29281673986369,38.2245786929335));
#64987=CARTESIAN_POINT('Ctrl Pts',(0.585453646372677,5.13413064150142,38.3833394551794));
#64988=CARTESIAN_POINT('Ctrl Pts',(-3.52014057613125,3.46939996827985,38.5256165935665));
#64989=CARTESIAN_POINT('Ctrl Pts',(-4.36087077121817,0.99889887186349,38.6149734778717));
#64990=CARTESIAN_POINT('Ctrl Pts',(-4.36873305544013,-0.00362749675167234,
38.651410108095));
#64991=CARTESIAN_POINT('Ctrl Pts',(-4.36935764006,-0.00377501215838787,
37.848589891905));
#64992=CARTESIAN_POINT('Ctrl Pts',(-4.37290446571934,-0.43375111631892,
37.8642229411018));
#64993=CARTESIAN_POINT('Ctrl Pts',(-4.11710236903147,-2.31513392579321,
37.9327762443806));
#64994=CARTESIAN_POINT('Ctrl Pts',(-1.42107210669624,-4.96815944202542,
38.0542498017413));
#64995=CARTESIAN_POINT('Ctrl Pts',(3.40313314014881,-3.88853944357485,38.2130105639872));
#64996=CARTESIAN_POINT('Ctrl Pts',(5.11268698707437,0.749990630619295,38.3717713262331));
#64997=CARTESIAN_POINT('Ctrl Pts',(2.14295353437204,4.70210637090854,38.5305320884789));
#64998=CARTESIAN_POINT('Ctrl Pts',(-2.78807645035559,4.35071073283309,38.6892928507248));
#64999=CARTESIAN_POINT('Ctrl Pts',(-4.37695363416618,1.45696557727882,38.7953121185335));
#65000=CARTESIAN_POINT('Ctrl Pts',(-4.37917461026378,0.0049794875180062,
38.8484111322603));
#65001=CARTESIAN_POINT('Ctrl Pts',(-4.37917310725098,9.13219796029981E-5,
38.848589891905));
#65002=CARTESIAN_POINT('Origin',(0.,0.,24.1514101080949));
#65003=CARTESIAN_POINT('',(-4.37768323182342,0.00228667983145002,36.651410108095));
#65004=CARTESIAN_POINT('',(-4.36587095680509,0.00214125659340675,36.848589891905));
#65005=CARTESIAN_POINT('',(-4.372,3.82579154166093E-12,24.1514101080949));
#65006=CARTESIAN_POINT('Ctrl Pts',(-4.37768323182342,0.00228667983144982,
36.651410108095));
#65007=CARTESIAN_POINT('Ctrl Pts',(-4.36931436006514,-1.31439298482965,
36.6995173496368));
#65008=CARTESIAN_POINT('Ctrl Pts',(-3.03668215072675,-4.09416581339981,
36.8005448452606));
#65009=CARTESIAN_POINT('Ctrl Pts',(1.69169298020808,-4.88264562268956,36.9544925949664));
#65010=CARTESIAN_POINT('Ctrl Pts',(5.01960663803976,-1.22702999775959,37.1132533572123));
#65011=CARTESIAN_POINT('Ctrl Pts',(3.75342297485632,3.55160096123927,37.2720141194582));
#65012=CARTESIAN_POINT('Ctrl Pts',(-0.94800804471325,5.07969823544803,37.430774881704));
#65013=CARTESIAN_POINT('Ctrl Pts',(-4.00191688963235,2.59358013793749,37.5572402112497));
#65014=CARTESIAN_POINT('Ctrl Pts',(-4.36914909948521,0.570748326013101,
37.6307852867133));
#65015=CARTESIAN_POINT('Ctrl Pts',(-4.36624352627694,0.00245771687439181,
37.651410108095));
#65016=CARTESIAN_POINT('Ctrl Pts',(-4.36587095680509,0.00214125659340626,
36.848589891905));
#65017=CARTESIAN_POINT('Ctrl Pts',(-4.36203103509102,-0.864466812036311,
36.8800347499434));
#65018=CARTESIAN_POINT('Ctrl Pts',(-3.6926137083843,-3.19500429871341,36.9643998620637));
#65019=CARTESIAN_POINT('Ctrl Pts',(0.100492274349119,-5.16642579319712,
37.101685228266));
#65020=CARTESIAN_POINT('Ctrl Pts',(4.39497597774354,-2.71776384714963,37.2604459905118));
#65021=CARTESIAN_POINT('Ctrl Pts',(4.66704342001788,2.21827858698683,37.4192067527577));
#65022=CARTESIAN_POINT('Ctrl Pts',(0.66769016759438,5.12408470011126,37.5779675150036));
#65023=CARTESIAN_POINT('Ctrl Pts',(-3.48876670478196,3.51583248140767,37.7210952280527));
#65024=CARTESIAN_POINT('Ctrl Pts',(-4.36089792030941,1.02178352666142,37.8113026870198));
#65025=CARTESIAN_POINT('Ctrl Pts',(-4.36935764006,-0.00377501215838787,
37.848589891905));
#65026=CARTESIAN_POINT('Origin',(0.,0.,24.1514101080949));
#65027=CARTESIAN_POINT('',(-4.37311107145795,-0.00391014173522758,35.651410108095));
#65028=CARTESIAN_POINT('',(-4.3771739373938,0.00261949572194539,35.848589891905));
#65029=CARTESIAN_POINT('',(-4.372,3.82579154166093E-12,24.1514101080949));
#65030=CARTESIAN_POINT('Ctrl Pts',(-4.37311107145795,-0.00391014173522778,
35.651410108095));
#65031=CARTESIAN_POINT('Ctrl Pts',(-4.3758959220056,-0.305762745961795,
35.6624089043964));
#65032=CARTESIAN_POINT('Ctrl Pts',(-4.20975035875682,-2.05692106559916,
35.7263279547798));
#65033=CARTESIAN_POINT('Ctrl Pts',(-1.84908860800444,-4.8252383087059,35.8431672592452));
#65034=CARTESIAN_POINT('Ctrl Pts',(3.05091116183891,-4.17061080641931,36.0019280214911));
#65035=CARTESIAN_POINT('Ctrl Pts',(5.15862384507246,0.301087098868051,36.1606887837369));
#65036=CARTESIAN_POINT('Ctrl Pts',(2.54500641307862,4.49722089444621,36.3194495459828));
#65037=CARTESIAN_POINT('Ctrl Pts',(-2.39787862639785,4.5773607580263,36.4782103082287));
#65038=CARTESIAN_POINT('Ctrl Pts',(-4.31337783157312,1.71331867151843,36.5888638289328));
#65039=CARTESIAN_POINT('Ctrl Pts',(-4.37852051709334,0.134017278681583,
36.6465970955549));
#65040=CARTESIAN_POINT('Ctrl Pts',(-4.37768323182342,0.00228667983144982,
36.651410108095));
#65041=CARTESIAN_POINT('Ctrl Pts',(-4.3771739373938,0.00261949572194524,
35.848589891905));
#65042=CARTESIAN_POINT('Ctrl Pts',(-4.36801132265503,-1.29117660831409,
35.8958465587849));
#65043=CARTESIAN_POINT('Ctrl Pts',(-3.07587918570516,-4.04972946385307,
35.9960234797468));
#65044=CARTESIAN_POINT('Ctrl Pts',(1.61319569609569,-4.90913982484862,36.1491206547906));
#65045=CARTESIAN_POINT('Ctrl Pts',(4.99928949022287,-1.30734798992603,36.3078814170365));
#65046=CARTESIAN_POINT('Ctrl Pts',(3.80988083761225,3.49096865884117,36.4666421792824));
#65047=CARTESIAN_POINT('Ctrl Pts',(-0.866447131906533,5.09424415801081,
36.6254029415283));
#65048=CARTESIAN_POINT('Ctrl Pts',(-3.9806269029927,2.64101706972627,36.7527188457358));
#65049=CARTESIAN_POINT('Ctrl Pts',(-4.36849344724489,0.59399482660225,36.8271144958614));
#65050=CARTESIAN_POINT('Ctrl Pts',(-4.36587095680509,0.00214125659340626,
36.848589891905));
#65051=CARTESIAN_POINT('Origin',(0.,0.,24.1514101080949));
#65052=CARTESIAN_POINT('',(-4.36484181559087,0.000158569877717519,34.651410108095));
#65053=CARTESIAN_POINT('',(-4.37381658707025,-0.00380592486605935,34.848589891905));
#65054=CARTESIAN_POINT('',(-4.372,3.82579154166093E-12,24.1514101080949));
#65055=CARTESIAN_POINT('Ctrl Pts',(-4.36484181559087,0.000158569877717965,
34.651410108095));
#65056=CARTESIAN_POINT('Ctrl Pts',(-4.36460260997581,-0.739166555623858,
34.6782207132379));
#65057=CARTESIAN_POINT('Ctrl Pts',(-3.83552704168218,-2.93813387262851,
34.7579515724629));
#65058=CARTESIAN_POINT('Ctrl Pts',(-0.350623086089188,-5.15549385292585,
34.8906026857698));
#65059=CARTESIAN_POINT('Ctrl Pts',(4.14111364246891,-3.09083018236409,35.0493634480157));
#65060=CARTESIAN_POINT('Ctrl Pts',(4.84277667347619,1.80265568173448,35.2081242102616));
#65061=CARTESIAN_POINT('Ctrl Pts',(1.11218256837853,5.0462960030749,35.3668849725075));
#65062=CARTESIAN_POINT('Ctrl Pts',(-3.30734354987895,3.76666274637145,35.5146469384519));
#65063=CARTESIAN_POINT('Ctrl Pts',(-4.36249672862818,1.14658859078299,35.6094886503144));
#65064=CARTESIAN_POINT('Ctrl Pts',(-4.37311107145795,-0.00391014173522778,
35.651410108095));
#65065=CARTESIAN_POINT('Ctrl Pts',(-4.37381658707025,-0.00380592486605963,
34.848589891905));
#65066=CARTESIAN_POINT('Ctrl Pts',(-4.37636167316891,-0.282199643018631,
34.8587381135445));
#65067=CARTESIAN_POINT('Ctrl Pts',(-4.22532647145104,-2.00959079533273,
34.921806589266));
#65068=CARTESIAN_POINT('Ctrl Pts',(-1.92621049372714,-4.7949731289833,35.0377953190694));
#65069=CARTESIAN_POINT('Ctrl Pts',(2.98365473640471,-4.21898786295316,35.1965560813153));
#65070=CARTESIAN_POINT('Ctrl Pts',(5.16278801485838,0.21834396591395,35.3553168435612));
#65071=CARTESIAN_POINT('Ctrl Pts',(2.61678000270041,4.45584072777334,35.514077605807));
#65072=CARTESIAN_POINT('Ctrl Pts',(-2.32418499851494,4.61521595014736,35.672838368053));
#65073=CARTESIAN_POINT('Ctrl Pts',(-4.30043031041834,1.76047520998047,35.7843424634189));
#65074=CARTESIAN_POINT('Ctrl Pts',(-4.37827205266511,0.157677555053939,
35.842926304703));
#65075=CARTESIAN_POINT('Ctrl Pts',(-4.3771739373938,0.00261949572194524,
35.848589891905));
#65076=CARTESIAN_POINT('Origin',(0.,0.,24.1514101080949));
#65077=CARTESIAN_POINT('',(-4.37369305382679,0.00382718076316987,33.651410108095));
#65078=CARTESIAN_POINT('',(-4.36484727915486,-0.000226203520788115,33.848589891905));
#65079=CARTESIAN_POINT('',(-4.372,3.82579154166093E-12,24.1514101080949));
#65080=CARTESIAN_POINT('Ctrl Pts',(-4.37369305382679,0.00382718076316957,
33.651410108095));
#65081=CARTESIAN_POINT('Ctrl Pts',(-4.36297801900768,-1.16550827733193,
33.6940325220795));
#65082=CARTESIAN_POINT('Ctrl Pts',(-3.27833228748252,-3.80423885928109,
33.789575190146));
#65083=CARTESIAN_POINT('Ctrl Pts',(1.17875881138994,-5.0311610072254,33.9380381122944));
#65084=CARTESIAN_POINT('Ctrl Pts',(4.86617124330449,-1.73851397661661,34.0967988745404));
#65085=CARTESIAN_POINT('Ctrl Pts',(4.09991511421076,3.14527414899259,34.2555596367862));
#65086=CARTESIAN_POINT('Ctrl Pts',(-0.418708560946466,5.15041129979394,
34.4143203990322));
#65087=CARTESIAN_POINT('Ctrl Pts',(-3.85575329743435,2.89916044399897,34.5462705561351));
#65088=CARTESIAN_POINT('Ctrl Pts',(-4.36507476723817,0.720154234863851,
34.625300459156));
#65089=CARTESIAN_POINT('Ctrl Pts',(-4.36484181559087,0.000158569877717965,
34.651410108095));
#65090=CARTESIAN_POINT('Ctrl Pts',(-4.36484727915486,-0.000226203520787838,
33.848589891905));
#65091=CARTESIAN_POINT('Ctrl Pts',(-4.36517770844991,-0.716093813355663,
33.8745499223861));
#65092=CARTESIAN_POINT('Ctrl Pts',(-3.86002428520416,-2.89083849180258,
33.9534302069491));
#65093=CARTESIAN_POINT('Ctrl Pts',(-0.433232286323001,-5.1492100326073,
34.085230745594));
#65094=CARTESIAN_POINT('Ctrl Pts',(4.0910284465022,-3.15682442079478,34.24399150784));
#65095=CARTESIAN_POINT('Ctrl Pts',(4.87105498299758,1.72478332738662,34.4027522700858));
#65096=CARTESIAN_POINT('Ctrl Pts',(1.1929432107418,5.02781669015105,34.5615130323318));
#65097=CARTESIAN_POINT('Ctrl Pts',(-3.27208568972255,3.81224566198089,34.7101255729381));
#65098=CARTESIAN_POINT('Ctrl Pts',(-4.36308973176021,1.16954893154173,34.8058178594626));
#65099=CARTESIAN_POINT('Ctrl Pts',(-4.37381658707025,-0.00380592486605963,
34.848589891905));
#65100=CARTESIAN_POINT('Origin',(0.,0.,24.1514101080949));
#65101=CARTESIAN_POINT('',(-4.37726747931578,-0.00256312102853162,32.651410108095));
#65102=CARTESIAN_POINT('',(-4.37298639645094,0.00392429018828133,32.848589891905));
#65103=CARTESIAN_POINT('',(-4.372,3.82579154166093E-12,24.1514101080949));
#65104=CARTESIAN_POINT('Ctrl Pts',(-4.37726747931578,-0.0025631210285324,
32.651410108095));
#65105=CARTESIAN_POINT('Ctrl Pts',(-4.37831848753371,-0.153516427525766,
32.6569240768391));
#65106=CARTESIAN_POINT('Ctrl Pts',(-4.30273715326605,-1.7521779604483,32.7153582996652));
#65107=CARTESIAN_POINT('Ctrl Pts',(-2.33719172860392,-4.60864277632799,
32.8267127765732));
#65108=CARTESIAN_POINT('Ctrl Pts',(2.60420302889879,-4.4632028858578,32.9854735388192));
#65109=CARTESIAN_POINT('Ctrl Pts',(5.16215162793603,-0.232903383943239,
33.144234301065));
#65110=CARTESIAN_POINT('Ctrl Pts',(2.99554137711165,4.21055640908263,33.302995063311));
#65111=CARTESIAN_POINT('Ctrl Pts',(-1.91267984204806,4.80038636339596,33.4617558255568));
#65112=CARTESIAN_POINT('Ctrl Pts',(-4.22261792613804,2.01791460332865,33.5778941738182));
#65113=CARTESIAN_POINT('Ctrl Pts',(-4.37628187282812,0.286345894322504,
33.6411122679975));
#65114=CARTESIAN_POINT('Ctrl Pts',(-4.37369305382679,0.00382718076316957,
33.651410108095));
#65115=CARTESIAN_POINT('Ctrl Pts',(-4.37298639645094,0.00392429018828126,
32.848589891905));
#65116=CARTESIAN_POINT('Ctrl Pts',(-4.36240284050621,-1.14255230782506,
32.8903617312276));
#65117=CARTESIAN_POINT('Ctrl Pts',(-3.31348194711132,-3.75862865123049,
32.9850538246322));
#65118=CARTESIAN_POINT('Ctrl Pts',(1.09794640645064,-5.04941262548215,33.1326661721187));
#65119=CARTESIAN_POINT('Ctrl Pts',(4.83767356537879,-1.81630632015957,33.2914269343646));
#65120=CARTESIAN_POINT('Ctrl Pts',(4.14981410860918,3.07913900917197,33.4501876966104));
#65121=CARTESIAN_POINT('Ctrl Pts',(-0.336081978081961,5.15646226378366,
33.6089484588564));
#65122=CARTESIAN_POINT('Ctrl Pts',(-3.83116330074657,2.94644944182165,33.7417491906212));
#65123=CARTESIAN_POINT('Ctrl Pts',(-4.36450411901545,0.743222493270702,
33.8216296683041));
#65124=CARTESIAN_POINT('Ctrl Pts',(-4.36484727915486,-0.000226203520787838,
33.848589891905));
#65125=CARTESIAN_POINT('Origin',(0.,0.,24.1514101080949));
#65126=CARTESIAN_POINT('',(-4.36593258301536,-0.00219842154078257,31.651410108095));
#65127=CARTESIAN_POINT('',(-4.37776688532802,-0.00222515354369623,31.848589891905));
#65128=CARTESIAN_POINT('',(-4.372,3.82579154166093E-12,24.1514101080949));
#65129=CARTESIAN_POINT('Ctrl Pts',(-4.36593258301536,-0.00219842154078276,
31.651410108095));
#65130=CARTESIAN_POINT('Ctrl Pts',(-4.36860855649085,-0.589907775928666,
31.6727358856806));
#65131=CARTESIAN_POINT('Ctrl Pts',(-3.98440775127391,-2.63267349583233,
31.7469819173483));
#65132=CARTESIAN_POINT('Ctrl Pts',(-0.880810653343035,-5.09178023966167,
31.8741482030979));
#65133=CARTESIAN_POINT('Ctrl Pts',(3.80002027066033,-3.5016994957634,32.0329089653438));
#65134=CARTESIAN_POINT('Ctrl Pts',(5.00295656982363,1.29324358746212,32.1916697275897));
#65135=CARTESIAN_POINT('Ctrl Pts',(1.62703419898677,4.90457063680218,32.3504304898356));
#65136=CARTESIAN_POINT('Ctrl Pts',(-3.06903058869073,4.05756105615878,32.5036772833373));
#65137=CARTESIAN_POINT('Ctrl Pts',(-4.36823144777778,1.29525626325957,32.6040038227571));
#65138=CARTESIAN_POINT('Ctrl Pts',(-4.37726747931578,-0.0025631210285324,
32.651410108095));
#65139=CARTESIAN_POINT('Ctrl Pts',(-4.37776688532802,-0.00222515354369674,
31.848589891905));
#65140=CARTESIAN_POINT('Ctrl Pts',(-4.37856029699079,-0.129854311945594,
31.8532532859872));
#65141=CARTESIAN_POINT('Ctrl Pts',(-4.31561362407578,-1.70502699061033,
31.9108369341514));
#65142=CARTESIAN_POINT('Ctrl Pts',(-2.41077837014428,-4.57058003144683,
32.0213408363975));
#65143=CARTESIAN_POINT('Ctrl Pts',(2.53231309568674,-4.50438059662262,32.1801015986434));
#65144=CARTESIAN_POINT('Ctrl Pts',(5.15775426583447,-0.31563445167244,32.3388623608893));
#65145=CARTESIAN_POINT('Ctrl Pts',(3.06266118623515,4.16198998462816,32.4976231231351));
#65146=CARTESIAN_POINT('Ctrl Pts',(-1.83547296121064,4.83043405735769,32.6563838853811));
#65147=CARTESIAN_POINT('Ctrl Pts',(-4.20696559908301,2.06524898522119,32.7733728083043));
#65148=CARTESIAN_POINT('Ctrl Pts',(-4.37581102359723,0.309905468748449,
32.8374414771457));
#65149=CARTESIAN_POINT('Ctrl Pts',(-4.37298639645094,0.00392429018828126,
32.848589891905));
#65150=CARTESIAN_POINT('Origin',(0.,0.,24.1514101080949));
#65151=CARTESIAN_POINT('',(-4.36924553642194,0.00375164274966603,30.651410108095));
#65152=CARTESIAN_POINT('',(-4.36631454878401,-0.00251114173366096,30.848589891905));
#65153=CARTESIAN_POINT('',(-4.372,3.82579154166093E-12,24.1514101080949));
#65154=CARTESIAN_POINT('Ctrl Pts',(-4.36924553642194,0.00375164274966585,
30.651410108095));
#65155=CARTESIAN_POINT('Ctrl Pts',(-4.36088767272676,-1.01775802631581,
30.6885476945222));
#65156=CARTESIAN_POINT('Ctrl Pts',(-3.49432807348169,-3.50767273053874,
30.7786055350314));
#65157=CARTESIAN_POINT('Ctrl Pts',(0.653236365857992,-5.12594729451212,
30.9215836296226));
#65158=CARTESIAN_POINT('Ctrl Pts',(4.6607687206244,-2.23143190555148,31.0803443918685));
#65159=CARTESIAN_POINT('Ctrl Pts',(4.4026231771807,2.70535812338375,31.2391051541143));
#65160=CARTESIAN_POINT('Ctrl Pts',(0.115062422136807,5.16612176153803,31.3978659163603));
#65161=CARTESIAN_POINT('Ctrl Pts',(-3.68772820349694,3.20326873769824,31.5353009010205));
#65162=CARTESIAN_POINT('Ctrl Pts',(-4.36196808602404,0.868502274330174,
31.6198156315987));
#65163=CARTESIAN_POINT('Ctrl Pts',(-4.36593258301536,-0.00219842154078276,
31.651410108095));
#65164=CARTESIAN_POINT('Ctrl Pts',(-4.36631454878401,-0.0025111417336611,
30.848589891905));
#65165=CARTESIAN_POINT('Ctrl Pts',(-4.36926463444175,-0.566656242129838,
30.8690650948288));
#65166=CARTESIAN_POINT('Ctrl Pts',(-4.00561083840711,-2.58523495481153,
30.9424605518345));
#65167=CARTESIAN_POINT('Ctrl Pts',(-0.962330244988123,-5.07700449806455,
31.0687762629221));
#65168=CARTESIAN_POINT('Ctrl Pts',(3.74339174195905,-3.56217243267071,31.2275370251681));
#65169=CARTESIAN_POINT('Ctrl Pts',(5.02304726326813,1.21286865108392,31.3862977874139));
#65170=CARTESIAN_POINT('Ctrl Pts',(1.70545649826175,4.87785529780762,31.5450585496599));
#65171=CARTESIAN_POINT('Ctrl Pts',(-3.02972114369421,4.10196041210765,31.6991559178235));
#65172=CARTESIAN_POINT('Ctrl Pts',(-4.36955665156738,1.31848296597982,31.8003330319052));
#65173=CARTESIAN_POINT('Ctrl Pts',(-4.37776688532802,-0.00222515354369674,
31.848589891905));
#65174=CARTESIAN_POINT('Origin',(0.,0.,24.1514101080949));
#65175=CARTESIAN_POINT('',(-4.37917542201394,-1.48878467067329E-5,29.651410108095));
#65176=CARTESIAN_POINT('',(-4.36862654983539,0.00359793095617206,29.848589891905));
#65177=CARTESIAN_POINT('',(-4.372,3.82579154166093E-12,24.1514101080949));
#65178=CARTESIAN_POINT('Ctrl Pts',(-4.3791753974872,-1.48877958181532E-5,
29.651410108095));
#65179=CARTESIAN_POINT('Ctrl Pts',(-4.37917543773958,-0.000811749618496727,
29.6514392492818));
#65180=CARTESIAN_POINT('Ctrl Pts',(-4.37881439934298,-1.44870578249893,
29.7043886445506));
#65181=CARTESIAN_POINT('Ctrl Pts',(-2.80033535833003,-4.34283033250174,
29.8102582939013));
#65182=CARTESIAN_POINT('Ctrl Pts',(2.12968392236957,-4.70813124181331,29.9690190561473));
#65183=CARTESIAN_POINT('Ctrl Pts',(5.11055143098187,-0.764406630547101,
30.1277798183931));
#65184=CARTESIAN_POINT('Ctrl Pts',(3.41408616315334,3.87892628001712,30.286540580639));
#65185=CARTESIAN_POINT('Ctrl Pts',(-1.4070550442568,4.97214737476293,30.4453013428849));
#65186=CARTESIAN_POINT('Ctrl Pts',(-4.11388660080008,2.32347755138503,30.5669245187036));
#65187=CARTESIAN_POINT('Ctrl Pts',(-4.37279744697119,0.437871066329566,
30.6356274404402));
#65188=CARTESIAN_POINT('Ctrl Pts',(-4.36924553642194,0.00375164274966585,
30.651410108095));
#65189=CARTESIAN_POINT('Ctrl Pts',(-4.36862654983539,0.0035979309561724,
29.848589891905));
#65190=CARTESIAN_POINT('Ctrl Pts',(-4.36087365922317,-0.994873321808196,
29.8848769036703));
#65191=CARTESIAN_POINT('Ctrl Pts',(-3.52559867611562,-3.46122138486278,
29.9740841695176));
#65192=CARTESIAN_POINT('Ctrl Pts',(0.570971856938151,-5.13576141485164,
30.1162116894468));
#65193=CARTESIAN_POINT('Ctrl Pts',(4.62439484690811,-2.30586783557282,30.2749724516927));
#65194=CARTESIAN_POINT('Ctrl Pts',(4.44543041863472,2.63442642081081,30.4337332139386));
#65195=CARTESIAN_POINT('Ctrl Pts',(0.1978722839815,5.16361314708889,30.5924939761844));
#65196=CARTESIAN_POINT('Ctrl Pts',(-3.65962554388572,3.25021066517935,30.7307795355066));
#65197=CARTESIAN_POINT('Ctrl Pts',(-4.361639836624,0.891434413344724,30.8161448407468));
#65198=CARTESIAN_POINT('Ctrl Pts',(-4.36631454878401,-0.0025111417336611,
30.848589891905));
#65199=CARTESIAN_POINT('Origin',(0.,0.,24.1514101080949));
#65200=CARTESIAN_POINT('',(-4.36920210772109,-0.00374225457618444,28.651410108095));
#65201=CARTESIAN_POINT('',(-4.379125585284,0.000418740495046069,28.848589891905));
#65202=CARTESIAN_POINT('',(-4.372,3.82579154166093E-12,24.1514101080949));
#65203=CARTESIAN_POINT('Ctrl Pts',(-4.36920210772109,-0.00374225457618473,
28.651410108095));
#65204=CARTESIAN_POINT('Ctrl Pts',(-4.37275566211042,-0.439475723050513,
28.6672510581234));
#65205=CARTESIAN_POINT('Ctrl Pts',(-4.11263026215736,-2.3267277008933,28.7360122622337));
#65206=CARTESIAN_POINT('Ctrl Pts',(-1.40159165779937,-4.9736902589037,28.857693720426));
#65207=CARTESIAN_POINT('Ctrl Pts',(3.41834539873403,-3.87517318393326,29.0164544826719));
#65208=CARTESIAN_POINT('Ctrl Pts',(5.10970861334159,0.770020576487015,29.1752152449178));
#65209=CARTESIAN_POINT('Ctrl Pts',(2.12451027984608,4.71046807932676,29.3339760071637));
#65210=CARTESIAN_POINT('Ctrl Pts',(-2.80419982800075,4.33981931003669,29.4927076282227));
#65211=CARTESIAN_POINT('Ctrl Pts',(-4.37910233962271,1.44628545901738,29.5985189951998));
#65212=CARTESIAN_POINT('Ctrl Pts',(-4.3791753974872,-1.48877958181532E-5,
29.651410108095));
#65213=CARTESIAN_POINT('Ctrl Pts',(-4.379125585284,0.000418740495045835,
28.848589891905));
#65214=CARTESIAN_POINT('Ctrl Pts',(-4.37717920749743,-1.42426027511931,
28.9006887125119));
#65215=CARTESIAN_POINT('Ctrl Pts',(-2.84412638479826,-4.2996753084771,29.0057077872007));
#65216=CARTESIAN_POINT('Ctrl Pts',(2.05392820456428,-4.74166985111631,29.1636471159715));
#65217=CARTESIAN_POINT('Ctrl Pts',(5.09763950196961,-0.846242130327758,
29.3224078782173));
#65218=CARTESIAN_POINT('Ctrl Pts',(3.47583539931961,3.82369225364773,29.4811686404633));
#65219=CARTESIAN_POINT('Ctrl Pts',(-1.32715942194175,4.9940666821606,29.6399294027091));
#65220=CARTESIAN_POINT('Ctrl Pts',(-4.09533214146315,2.37091623060187,29.7624031531897));
#65221=CARTESIAN_POINT('Ctrl Pts',(-4.37218032023241,0.461277235079317,
29.8319566495884));
#65222=CARTESIAN_POINT('Ctrl Pts',(-4.36862654983539,0.0035979309561724,
29.848589891905));
#65223=CARTESIAN_POINT('Origin',(0.,0.,24.1514101080949));
#65224=CARTESIAN_POINT('',(-4.36594998909341,0.00221597220681413,27.651410108095));
#65225=CARTESIAN_POINT('',(-4.36984836444492,-0.00386263586949487,27.848589891905));
#65226=CARTESIAN_POINT('',(-4.372,3.82579154166093E-12,24.1514101080949));
#65227=CARTESIAN_POINT('Ctrl Pts',(-4.36594998909341,0.00221597220681394,
27.651410108095));
#65228=CARTESIAN_POINT('Ctrl Pts',(-4.36193991209169,-0.870076739562532,
27.6830628669649));
#65229=CARTESIAN_POINT('Ctrl Pts',(-3.68583197785541,-3.20648009630763,
27.7676358799168));
#65230=CARTESIAN_POINT('Ctrl Pts',(0.12074539761077,-5.16599709979471,27.9051291469506));
#65231=CARTESIAN_POINT('Ctrl Pts',(4.40558866999103,-2.70051724468854,28.0638899091966));
#65232=CARTESIAN_POINT('Ctrl Pts',(4.65831652566081,2.23654953809766,28.2226506714425));
#65233=CARTESIAN_POINT('Ctrl Pts',(0.647603546994949,5.12666253671564,28.3814114336883));
#65234=CARTESIAN_POINT('Ctrl Pts',(-3.49648913171247,3.50449301705117,28.5243312459059));
#65235=CARTESIAN_POINT('Ctrl Pts',(-4.36088421495349,1.0161898665986,28.6143308040414));
#65236=CARTESIAN_POINT('Ctrl Pts',(-4.36920210772109,-0.00374225457618473,
28.651410108095));
#65237=CARTESIAN_POINT('Ctrl Pts',(-4.36984836444492,-0.00386263586949508,
27.848589891905));
#65238=CARTESIAN_POINT('Ctrl Pts',(-4.37335795381477,-0.41604489030568,
27.8635802672715));
#65239=CARTESIAN_POINT('Ctrl Pts',(-4.13075387899131,-2.27929715120676,
27.9314908967199));
#65240=CARTESIAN_POINT('Ctrl Pts',(-1.48115027726835,-4.95058115072351,
28.0523217802503));
#65241=CARTESIAN_POINT('Ctrl Pts',(3.35577787359124,-3.92947861571792,28.2110825424961));
#65242=CARTESIAN_POINT('Ctrl Pts',(5.12139735341277,0.688001195909337,28.369843304742));
#65243=CARTESIAN_POINT('Ctrl Pts',(2.1997566305386,4.67580212267651,28.5286040669879));
#65244=CARTESIAN_POINT('Ctrl Pts',(-2.7351680780718,4.38416569184913,28.6873648292338));
#65245=CARTESIAN_POINT('Ctrl Pts',(-4.36882639464741,1.49245678983841,28.7940267708728));
#65246=CARTESIAN_POINT('Ctrl Pts',(-4.37915627350017,0.0228814185571984,
28.8477684584299));
#65247=CARTESIAN_POINT('Ctrl Pts',(-4.379125585284,0.000418740495045835,
28.848589891905));
#65248=CARTESIAN_POINT('Origin',(0.,0.,24.1514101080949));
#65249=CARTESIAN_POINT('',(-4.37688026104952,0.00226901643694793,26.651410108095));
#65250=CARTESIAN_POINT('',(-4.36558297706963,0.00185075076461538,26.848589891905));
#65251=CARTESIAN_POINT('',(-4.372,3.82579154166093E-12,24.1514101080949));
#65252=CARTESIAN_POINT('Ctrl Pts',(-4.37688026104952,0.00226901643694839,
26.651410108095));
#65253=CARTESIAN_POINT('Ctrl Pts',(-4.36778028862692,-1.29719233300268,
26.6988746758065));
#65254=CARTESIAN_POINT('Ctrl Pts',(-3.06703503858937,-4.06017418671544,
26.7992594975999));
#65255=CARTESIAN_POINT('Ctrl Pts',(1.63279456941769,-4.90302026906412,26.9525645734753));
#65256=CARTESIAN_POINT('Ctrl Pts',(5.00417945325775,-1.28762125191842,27.1113253357213));
#65257=CARTESIAN_POINT('Ctrl Pts',(3.79627275763131,3.50580663842047,27.2700860979671));
#65258=CARTESIAN_POINT('Ctrl Pts',(-0.886457053099411,5.09084367591115,
27.428846860213));
#65259=CARTESIAN_POINT('Ctrl Pts',(-3.98586478860146,2.62941579049566,27.5559548635889));
#65260=CARTESIAN_POINT('Ctrl Pts',(-4.3686443606578,0.588309625125352,27.6301426128829));
#65261=CARTESIAN_POINT('Ctrl Pts',(-4.36594998909341,0.00221597220681394,
27.651410108095));
#65262=CARTESIAN_POINT('Ctrl Pts',(-4.36558297706963,0.00185075076461511,
26.848589891905));
#65263=CARTESIAN_POINT('Ctrl Pts',(-4.36229437398082,-0.847147845875526,
26.879392076113));
#65264=CARTESIAN_POINT('Ctrl Pts',(-3.7134735047561,-3.15941742864277,26.963114514403));
#65265=CARTESIAN_POINT('Ctrl Pts',(0.037946527963305,-5.16730646950401,
27.0997572067749));
#65266=CARTESIAN_POINT('Ctrl Pts',(4.36170657063856,-2.77078223288025,27.2585179690208));
#65267=CARTESIAN_POINT('Ctrl Pts',(4.69358555482947,2.16156853417802,27.4172787312667));
#65268=CARTESIAN_POINT('Ctrl Pts',(0.729706757950081,5.11562647870316,27.5760394935125));
#65269=CARTESIAN_POINT('Ctrl Pts',(-3.46466751885718,3.55083973542589,27.719809880392));
#65270=CARTESIAN_POINT('Ctrl Pts',(-4.36096811322469,1.03907475143884,27.8106600131895));
#65271=CARTESIAN_POINT('Ctrl Pts',(-4.36984836444492,-0.00386263586949508,
27.848589891905));
#65272=CARTESIAN_POINT('Ctrl Pts',(-1.91898364243938,3.92834389788497,25.6709103465619));
#65273=CARTESIAN_POINT('Ctrl Pts',(-2.57208606313318,3.60930541889036,25.6973704736029));
#65274=CARTESIAN_POINT('Ctrl Pts',(-3.70615701990389,2.63929385761509,25.7502907276849));
#65275=CARTESIAN_POINT('Ctrl Pts',(-4.81803798679934,-0.15958129715831,
25.8561312358487));
#65276=CARTESIAN_POINT('Ctrl Pts',(-3.30234769881301,-3.97407004593024,
25.9884318710537));
#65277=CARTESIAN_POINT('Ctrl Pts',(1.55593458522165,-4.93043777696371,26.1471926332996));
#65278=CARTESIAN_POINT('Ctrl Pts',(4.98187809541805,-1.36671674862893,26.3059533955455));
#65279=CARTESIAN_POINT('Ctrl Pts',(3.85252000415521,3.44398917781397,26.4647141577913));
#65280=CARTESIAN_POINT('Ctrl Pts',(-0.805001512196143,5.10466442465425,
26.6234749200372));
#65281=CARTESIAN_POINT('Ctrl Pts',(-4.72460311480109,2.09234479401288,26.7822356822831));
#65282=CARTESIAN_POINT('Ctrl Pts',(-4.32070810303542,-2.83440458431113,
26.940996444529));
#65283=CARTESIAN_POINT('Ctrl Pts',(0.037946527963305,-5.16730646950401,
27.0997572067749));
#65284=CARTESIAN_POINT('Ctrl Pts',(4.36170657063856,-2.77078223288025,27.2585179690208));
#65285=CARTESIAN_POINT('Ctrl Pts',(4.69358555482947,2.16156853417802,27.4172787312667));
#65286=CARTESIAN_POINT('Ctrl Pts',(0.729706757950081,5.11562647870316,27.5760394935125));
#65287=CARTESIAN_POINT('Ctrl Pts',(-3.90199850336257,3.38768554797952,27.7348002557585));
#65288=CARTESIAN_POINT('Ctrl Pts',(-4.96248778940575,-1.44075757294651,
27.8935610180043));
#65289=CARTESIAN_POINT('Ctrl Pts',(-1.48115027726835,-4.95058115072351,
28.0523217802503));
#65290=CARTESIAN_POINT('Ctrl Pts',(3.35577787359124,-3.92947861571792,28.2110825424961));
#65291=CARTESIAN_POINT('Ctrl Pts',(5.12139735341277,0.688001195909337,28.369843304742));
#65292=CARTESIAN_POINT('Ctrl Pts',(2.1997566305386,4.67580212267651,28.5286040669879));
#65293=CARTESIAN_POINT('Ctrl Pts',(-2.7351680780718,4.38416569184913,28.6873648292338));
#65294=CARTESIAN_POINT('Ctrl Pts',(-5.16678366281907,0.0800071286185968,
28.8461255914797));
#65295=CARTESIAN_POINT('Ctrl Pts',(-2.86960088841888,-4.29737651997417,
29.0048863537256));
#65296=CARTESIAN_POINT('Ctrl Pts',(2.05392820456428,-4.74166985111631,29.1636471159715));
#65297=CARTESIAN_POINT('Ctrl Pts',(5.09763950196961,-0.846242130327758,
29.3224078782173));
#65298=CARTESIAN_POINT('Ctrl Pts',(3.47583539931961,3.82369225364773,29.4811686404633));
#65299=CARTESIAN_POINT('Ctrl Pts',(-1.32715942194175,4.9940666821606,29.6399294027091));
#65300=CARTESIAN_POINT('Ctrl Pts',(-4.9154974066526,1.59371874196162,29.798690164955));
#65301=CARTESIAN_POINT('Ctrl Pts',(-4.00502201634919,-3.26524927403143,
29.9574509272009));
#65302=CARTESIAN_POINT('Ctrl Pts',(0.570971856938151,-5.13576141485164,
30.1162116894468));
#65303=CARTESIAN_POINT('Ctrl Pts',(4.62439484690811,-2.30586783557282,30.2749724516927));
#65304=CARTESIAN_POINT('Ctrl Pts',(4.44543041863472,2.63442642081081,30.4337332139386));
#65305=CARTESIAN_POINT('Ctrl Pts',(0.1978722839815,5.16361314708889,30.5924939761844));
#65306=CARTESIAN_POINT('Ctrl Pts',(-4.23078460916092,2.96690339662622,30.7512547384304));
#65307=CARTESIAN_POINT('Ctrl Pts',(-4.7872981969476,-1.94520696772118,30.9100155006763));
#65308=CARTESIAN_POINT('Ctrl Pts',(-0.962330244988123,-5.07700449806455,
31.0687762629221));
#65309=CARTESIAN_POINT('Ctrl Pts',(3.74339174195905,-3.56217243267071,31.2275370251681));
#65310=CARTESIAN_POINT('Ctrl Pts',(5.02304726326813,1.21286865108392,31.3862977874139));
#65311=CARTESIAN_POINT('Ctrl Pts',(1.70545649826175,4.87785529780762,31.5450585496599));
#65312=CARTESIAN_POINT('Ctrl Pts',(-3.17302014780288,4.07847977994959,31.7038193119056));
#65313=CARTESIAN_POINT('Ctrl Pts',(-5.14745183343486,-0.453645011306304,
31.8625800741516));
#65314=CARTESIAN_POINT('Ctrl Pts',(-2.41077837014428,-4.57058003144683,
32.0213408363975));
#65315=CARTESIAN_POINT('Ctrl Pts',(2.53231309568674,-4.50438059662262,32.1801015986434));
#65316=CARTESIAN_POINT('Ctrl Pts',(5.15775426583447,-0.31563445167244,32.3388623608893));
#65317=CARTESIAN_POINT('Ctrl Pts',(3.06266118623515,4.16198998462816,32.4976231231351));
#65318=CARTESIAN_POINT('Ctrl Pts',(-1.83547296121064,4.83043405735769,32.6563838853811));
#65319=CARTESIAN_POINT('Ctrl Pts',(-5.05372618930481,1.07791733326401,32.8151446476269));
#65320=CARTESIAN_POINT('Ctrl Pts',(-3.64665484087083,-3.66114225964655,
32.9739054098729));
#65321=CARTESIAN_POINT('Ctrl Pts',(1.09794640645064,-5.04941262548215,33.1326661721187));
#65322=CARTESIAN_POINT('Ctrl Pts',(4.83767356537879,-1.81630632015957,33.2914269343646));
#65323=CARTESIAN_POINT('Ctrl Pts',(4.14981410860918,3.07913900917197,33.4501876966104));
#65324=CARTESIAN_POINT('Ctrl Pts',(-0.336081978081961,5.15646226378366,
33.6089484588564));
#65325=CARTESIAN_POINT('Ctrl Pts',(-4.51438557267483,2.51443374838985,33.7677092211023));
#65326=CARTESIAN_POINT('Ctrl Pts',(-4.56098559745287,-2.42888133790924,
33.9264699833482));
#65327=CARTESIAN_POINT('Ctrl Pts',(-0.433232286323001,-5.1492100326073,
34.085230745594));
#65328=CARTESIAN_POINT('Ctrl Pts',(4.0910284465022,-3.15682442079478,34.24399150784));
#65329=CARTESIAN_POINT('Ctrl Pts',(4.87105498299758,1.72478332738662,34.4027522700858));
#65330=CARTESIAN_POINT('Ctrl Pts',(1.1929432107418,5.02781669015105,34.5615130323318));
#65331=CARTESIAN_POINT('Ctrl Pts',(-3.5769866269097,3.72923864142877,34.7202737945776));
#65332=CARTESIAN_POINT('Ctrl Pts',(-5.07314904313429,-0.982452523006609,
34.8790345568235));
#65333=CARTESIAN_POINT('Ctrl Pts',(-1.92621049372714,-4.7949731289833,35.0377953190694));
#65334=CARTESIAN_POINT('Ctrl Pts',(2.98365473640471,-4.21898786295316,35.1965560813153));
#65335=CARTESIAN_POINT('Ctrl Pts',(5.16278801485838,0.21834396591395,35.3553168435612));
#65336=CARTESIAN_POINT('Ctrl Pts',(2.61678000270041,4.45584072777334,35.514077605807));
#65337=CARTESIAN_POINT('Ctrl Pts',(-2.32418499851494,4.61521595014736,35.672838368053));
#65338=CARTESIAN_POINT('Ctrl Pts',(-5.13798489593422,0.55060456133973,35.8315991302988));
#65339=CARTESIAN_POINT('Ctrl Pts',(-3.24934407480239,-4.01793694044132,
35.9903598925447));
#65340=CARTESIAN_POINT('Ctrl Pts',(1.61319569609569,-4.90913982484862,36.1491206547906));
#65341=CARTESIAN_POINT('Ctrl Pts',(4.99928949022287,-1.30734798992603,36.3078814170365));
#65342=CARTESIAN_POINT('Ctrl Pts',(3.80988083761225,3.49096865884117,36.4666421792824));
#65343=CARTESIAN_POINT('Ctrl Pts',(-0.866447131906533,5.09424415801081,
36.6254029415283));
#65344=CARTESIAN_POINT('Ctrl Pts',(-4.74977622033223,2.03511179805508,36.7841637037742));
#65345=CARTESIAN_POINT('Ctrl Pts',(-4.28596502810612,-2.88661704277997,
36.94292446602));
#65346=CARTESIAN_POINT('Ctrl Pts',(0.100492274349119,-5.16642579319712,
37.101685228266));
#65347=CARTESIAN_POINT('Ctrl Pts',(4.39497597774354,-2.71776384714963,37.2604459905118));
#65348=CARTESIAN_POINT('Ctrl Pts',(4.66704342001788,2.21827858698683,37.4192067527577));
#65349=CARTESIAN_POINT('Ctrl Pts',(0.66769016759438,5.12408470011126,37.5779675150036));
#65350=CARTESIAN_POINT('Ctrl Pts',(-3.9427535210732,3.34017197848871,37.7367282772495));
#65351=CARTESIAN_POINT('Ctrl Pts',(-4.94466875428017,-1.50076816472822,
37.8954890394954));
#65352=CARTESIAN_POINT('Ctrl Pts',(-1.42107210669624,-4.96815944202542,
38.0542498017413));
#65353=CARTESIAN_POINT('Ctrl Pts',(3.40313314014881,-3.88853944357485,38.2130105639872));
#65354=CARTESIAN_POINT('Ctrl Pts',(5.11268698707437,0.749990630619295,38.3717713262331));
#65355=CARTESIAN_POINT('Ctrl Pts',(2.14295353437204,4.70210637090854,38.5305320884789));
#65356=CARTESIAN_POINT('Ctrl Pts',(-2.78807645035559,4.35071073283309,38.6892928507248));
#65357=CARTESIAN_POINT('Ctrl Pts',(-5.16737370481374,0.0174117378790549,
38.8480536129707));
#65358=CARTESIAN_POINT('Ctrl Pts',(-2.81733270514135,-4.33182301143032,
39.0068143752166));
#65359=CARTESIAN_POINT('Ctrl Pts',(2.11121724282438,-4.71644102342194,39.1655751374625));
#65360=CARTESIAN_POINT('Ctrl Pts',(5.10751668218689,-0.784428145210908,
39.3243358997084));
#65361=CARTESIAN_POINT('Ctrl Pts',(3.42926084288352,3.86551733216684,39.4830966619543));
#65362=CARTESIAN_POINT('Ctrl Pts',(-1.38755926796319,4.97762327338117,39.6418574242002));
#65363=CARTESIAN_POINT('Ctrl Pts',(-4.93444275322028,1.53405635131447,39.8006181864461));
#65364=CARTESIAN_POINT('Ctrl Pts',(-3.96517350621375,-3.31352580183661,
39.959378948692));
#65365=CARTESIAN_POINT('Ctrl Pts',(0.6331436514814,-5.12846792818335,40.1181397109379));
#65366=CARTESIAN_POINT('Ctrl Pts',(4.65198839971611,-2.2496795555641,40.2769004731838));
#65367=CARTESIAN_POINT('Ctrl Pts',(4.41319126769477,2.68808426366416,40.4356612354296));
#65368=CARTESIAN_POINT('Ctrl Pts',(0.135306684796697,5.16563125618407,40.5944219976755));
#65369=CARTESIAN_POINT('Ctrl Pts',(-4.26641470902384,2.91543473678309,40.7531827599214));
#65370=CARTESIAN_POINT('Ctrl Pts',(-4.7633830418116,-2.00305670683536,40.9119435221673));
#65371=CARTESIAN_POINT('Ctrl Pts',(-0.90075771530386,-5.08828946819429,
41.0707042844132));
#65372=CARTESIAN_POINT('Ctrl Pts',(3.78626858625262,-3.51656428443629,41.2294650466591));
#65373=CARTESIAN_POINT('Ctrl Pts',(5.00798622459088,1.27362794729248,41.3882258089049));
#65374=CARTESIAN_POINT('Ctrl Pts',(1.64624189925253,4.89815697818699,41.5469865711509));
#65375=CARTESIAN_POINT('Ctrl Pts',(-3.22219329739529,4.03974312649174,41.7057473333967));
#65376=CARTESIAN_POINT('Ctrl Pts',(-5.14157876509112,-0.515967030129218,
41.8645080956427));
#65377=CARTESIAN_POINT('Ctrl Pts',(-2.35523429540729,-4.59944840035779,
42.0232688578885));
#65378=CARTESIAN_POINT('Ctrl Pts',(2.58669254300161,-4.47337410259821,42.1820296201345));
#65379=CARTESIAN_POINT('Ctrl Pts',(5.16119935450289,-0.253131185149624,
42.3407903823802));
#65380=CARTESIAN_POINT('Ctrl Pts',(3.01201886587614,4.19878512494061,42.4995511446263));
#65381=CARTESIAN_POINT('Ctrl Pts',(-1.89385329211466,4.80784503512363,42.6583119068721));
#65382=CARTESIAN_POINT('Ctrl Pts',(-5.0664130686601,1.01661831162269,42.817072669118));
#65383=CARTESIAN_POINT('Ctrl Pts',(-3.6020368491656,-3.70504854368597,42.9758334313639));
#65384=CARTESIAN_POINT('Ctrl Pts',(1.15903352033341,-5.0357417996319,43.1345941936098));
#65385=CARTESIAN_POINT('Ctrl Pts',(4.85932100888344,-1.75757034181863,43.2933549558556));
#65386=CARTESIAN_POINT('Ctrl Pts',(4.11220948021047,3.12918317851219,43.4521157181016));
#65387=CARTESIAN_POINT('Ctrl Pts',(-0.398521773825228,5.15201267172389,
43.6108764803474));
#65388=CARTESIAN_POINT('Ctrl Pts',(-4.54451372744996,2.45956279749778,43.7696372425933));
#65389=CARTESIAN_POINT('Ctrl Pts',(-4.53122790373328,-2.48395407732217,
43.9283980048393));
#65390=CARTESIAN_POINT('Ctrl Pts',(-0.370823894361365,-5.15408030721166,
44.0871587670851));
#65391=CARTESIAN_POINT('Ctrl Pts',(4.12896947009338,-3.10703480650815,44.245919529331));
#65392=CARTESIAN_POINT('Ctrl Pts',(4.84980385450403,1.78366385472551,44.4046802915768));
#65393=CARTESIAN_POINT('Ctrl Pts',(1.13194961208497,5.04189887339256,44.5634410538228));
#65394=CARTESIAN_POINT('Ctrl Pts',(-3.62189949116538,3.68563403632435,44.7222018160687));
#65395=CARTESIAN_POINT('Ctrl Pts',(-5.06087554774066,-1.0438356499454,44.8809625783145));
#65396=CARTESIAN_POINT('Ctrl Pts',(-1.8679837165673,-4.81795506501003,45.0397233405604));
#65397=CARTESIAN_POINT('Ctrl Pts',(3.03454387031403,-4.18253483822383,45.1984841028063));
#65398=CARTESIAN_POINT('Ctrl Pts',(5.15976421573454,0.280869029694986,45.3572448650522));
#65399=CARTESIAN_POINT('Ctrl Pts',(2.56261074386464,4.4872129823807,45.5160056272982));
#65400=CARTESIAN_POINT('Ctrl Pts',(-2.37992235675453,4.58672254988638,45.6747663895439));
#65401=CARTESIAN_POINT('Ctrl Pts',(-5.14427782079704,0.488323536471552,
45.8335271517899));
#65402=CARTESIAN_POINT('Ctrl Pts',(-3.20043308923407,-4.05700409355871,
45.9922879140358));
#65403=CARTESIAN_POINT('Ctrl Pts',(1.67254576409749,-4.88923765436041,46.1510486762816));
#65404=CARTESIAN_POINT('Ctrl Pts',(5.01475964555148,-1.2466915701828,46.3098094385276));
#65405=CARTESIAN_POINT('Ctrl Pts',(3.76731232156889,3.53686471971598,46.4685702007735));
#65406=CARTESIAN_POINT('Ctrl Pts',(-0.928094313166731,5.08337438319113,
46.6273309630193));
#65407=CARTESIAN_POINT('Ctrl Pts',(-4.77408068348225,1.97742453747749,46.7860917252652));
#65408=CARTESIAN_POINT('Ctrl Pts',(-4.25068258608159,-2.93832464615453,
46.9448524875111));
#65409=CARTESIAN_POINT('Ctrl Pts',(0.163070052891163,-5.16482936133098,
47.103613249757));
#65410=CARTESIAN_POINT('Ctrl Pts',(4.42757599841828,-2.66432448325026,47.2623740120029));
#65411=CARTESIAN_POINT('Ctrl Pts',(4.63982914812316,2.27465154475207,47.4211347742487));
#65412=CARTESIAN_POINT('Ctrl Pts',(0.605568936039063,5.13179699886122,47.5798955364947));
#65413=CARTESIAN_POINT('Ctrl Pts',(-3.982926463652,3.29216508683222,47.7386562987406));
#65414=CARTESIAN_POINT('Ctrl Pts',(-4.92612590373581,-1.56055687315755,
47.8974170609864));
#65415=CARTESIAN_POINT('Ctrl Pts',(-1.36078444624568,-4.98500951500319,
48.0561778232324));
#65416=CARTESIAN_POINT('Ctrl Pts',(3.44998850215064,-3.84702917961962,48.2149385854782));
#65417=CARTESIAN_POINT('Ctrl Pts',(5.10322659210776,0.811869769988193,48.3736993477241));
#65418=CARTESIAN_POINT('Ctrl Pts',(2.08583582488191,4.72772070721777,48.53246010997));
#65419=CARTESIAN_POINT('Ctrl Pts',(-2.8405756019607,4.31661724309231,48.6912208722158));
#65420=CARTESIAN_POINT('Ctrl Pts',(-5.16720547137737,-0.0451861747017031,
48.8499816344618));
#65421=CARTESIAN_POINT('Ctrl Pts',(-2.76465105904324,-4.36563382517906,
49.0087423967076));
#65422=CARTESIAN_POINT('Ctrl Pts',(2.16819644989342,-4.69052004883103,49.1675031589536));
#65423=CARTESIAN_POINT('Ctrl Pts',(5.11664433946473,-0.72249904999246,49.3262639211995));
#65424=CARTESIAN_POINT('Ctrl Pts',(3.38218303962157,3.90677514842007,49.4850246834453));
#65425=CARTESIAN_POINT('Ctrl Pts',(-1.44775548820939,4.96044939699782,49.6437854456913));
#65426=CARTESIAN_POINT('Ctrl Pts',(-4.95266397096391,1.47416883854343,49.8025462079371));
#65427=CARTESIAN_POINT('Ctrl Pts',(-3.92474310640146,-3.36131607001936,
49.961306970183));
#65428=CARTESIAN_POINT('Ctrl Pts',(0.695222531978707,-5.12042183856424,
50.1200677324289));
#65429=CARTESIAN_POINT('Ctrl Pts',(4.67889927324325,-2.19316113513354,50.2788284946747));
#65430=CARTESIAN_POINT('Ctrl Pts',(4.38030448079635,2.74134763015048,50.4375892569207));
#65431=CARTESIAN_POINT('Ctrl Pts',(0.0727212293821569,5.16689130876717,
50.5963500191666));
#65432=CARTESIAN_POINT('Ctrl Pts',(-4.30141871246148,2.86353823685011,50.7551107814125));
#65433=CARTESIAN_POINT('Ctrl Pts',(-4.73876886011502,-2.06061249734653,
50.9138715436583));
#65434=CARTESIAN_POINT('Ctrl Pts',(-0.839052999411725,-5.09882773174331,
51.0726323059043));
#65435=CARTESIAN_POINT('Ctrl Pts',(3.82858979556074,-3.47044008032763,51.2313930681501));
#65436=CARTESIAN_POINT('Ctrl Pts',(4.99219026383802,1.33420033857639,51.390153830396));
#65437=CARTESIAN_POINT('Ctrl Pts',(1.58678571421362,4.91773985393535,51.548914592642));
#65438=CARTESIAN_POINT('Ctrl Pts',(-3.27089359005984,4.00041364065291,51.7076753548878));
#65439=CARTESIAN_POINT('Ctrl Pts',(-5.1349511699649,-0.578213330780779,
51.8664361171337));
#65440=CARTESIAN_POINT('Ctrl Pts',(-2.2993445899923,-4.62764180012773,52.0251968793796));
#65441=CARTESIAN_POINT('Ctrl Pts',(2.64069239313623,-4.44171114083851,52.1839576416255));
#65442=CARTESIAN_POINT('Ctrl Pts',(5.16388703706709,-0.190590771620509,
52.3427184038713));
#65443=CARTESIAN_POINT('Ctrl Pts',(2.96093453169081,4.23496409345547,52.5014791661172));
#65444=CARTESIAN_POINT('Ctrl Pts',(-1.95195570001178,4.78455046153847,52.6602399283632));
#65445=CARTESIAN_POINT('Ctrl Pts',(-5.07835645180041,0.955170101224678,
52.819000690609));
#65446=CARTESIAN_POINT('Ctrl Pts',(-3.5568902584837,-3.7484111117806,52.9777614528549));
#65447=CARTESIAN_POINT('Ctrl Pts',(1.21995054602492,-5.021331978576,53.1365222151008));
#65448=CARTESIAN_POINT('Ctrl Pts',(4.88025534693686,-1.69857643999627,53.2952829773467));
#65449=CARTESIAN_POINT('Ctrl Pts',(4.07400138499168,3.17876814016096,53.4540437395925));
#65450=CARTESIAN_POINT('Ctrl Pts',(-0.460903086490536,5.14680702170578,
53.6128045018385));
#65451=CARTESIAN_POINT('Ctrl Pts',(-4.57397497474849,2.404330905718,53.7715652640843));
#65452=CARTESIAN_POINT('Ctrl Pts',(-4.5008052522319,-2.53866229642665,53.9303260263303));
#65453=CARTESIAN_POINT('Ctrl Pts',(-0.308361083986154,-5.15819422043212,
54.0890867885761));
#65454=CARTESIAN_POINT('Ctrl Pts',(4.16630456733569,-3.05678923480409,54.2478475508221));
#65455=CARTESIAN_POINT('Ctrl Pts',(4.82784101720183,1.84228262935957,54.4066083130679));
#65456=CARTESIAN_POINT('Ctrl Pts',(1.07078989980086,5.0552411578777,54.5653690753139));
#65457=CARTESIAN_POINT('Ctrl Pts',(-3.66628084160122,3.64148856435446,54.7241298375597));
#65458=CARTESIAN_POINT('Ctrl Pts',(-5.04785936876341,-1.10506559398251,
54.8828905998056));
#65459=CARTESIAN_POINT('Ctrl Pts',(-1.80948281276126,-4.84022996603858,
55.0416513620516));
#65460=CARTESIAN_POINT('Ctrl Pts',(3.08498768485217,-4.1454680264268,55.2004121242973));
#65461=CARTESIAN_POINT('Ctrl Pts',(5.15598322111311,0.34335287594041,55.3591728865433));
#65462=CARTESIAN_POINT('Ctrl Pts',(2.50806542185317,4.51792673839683,55.5179336487891));
#65463=CARTESIAN_POINT('Ctrl Pts',(-2.43531046134262,4.55755604800332,55.6766944110351));
#65464=CARTESIAN_POINT('Ctrl Pts',(-5.14981582279099,0.425970850115064,
55.8354551732808));
#65465=CARTESIAN_POINT('Ctrl Pts',(-3.15105244004859,-4.09547588124754,
55.9942159355269));
#65466=CARTESIAN_POINT('Ctrl Pts',(1.73165038597632,-4.86861798815274,56.1529766977727));
#65467=CARTESIAN_POINT('Ctrl Pts',(5.02949388480597,-1.18585219842773,56.3117374600186));
#65468=CARTESIAN_POINT('Ctrl Pts',(3.72419095237009,3.58224174562538,56.4704982222645));
#65469=CARTESIAN_POINT('Ctrl Pts',(-0.989605296568694,5.07175862308326,
56.6292589845104));
#65470=CARTESIAN_POINT('Ctrl Pts',(-4.79768455020047,1.91944708981109,56.7880197467563));
#65471=CARTESIAN_POINT('Ctrl Pts',(-4.21477635630603,-2.98960105033098,
56.9467805090022));
#65472=CARTESIAN_POINT('Ctrl Pts',(0.225623900899773,-5.162474990657,57.1055412712481));
#65473=CARTESIAN_POINT('Ctrl Pts',(4.45952627223033,-2.61049412968195,57.2643020334939));
#65474=CARTESIAN_POINT('Ctrl Pts',(4.61193398121205,2.33069069735948,57.4230627957398));
#65475=CARTESIAN_POINT('Ctrl Pts',(0.543358837230748,5.13875620630321,57.5818235579857));
#65476=CARTESIAN_POINT('Ctrl Pts',(-4.02251491169591,3.24367506988608,57.7405843202316));
#65477=CARTESIAN_POINT('Ctrl Pts',(-4.90686014412063,-1.62011656983585,
57.8993450824775));
#65478=CARTESIAN_POINT('Ctrl Pts',(-1.30029709065152,-5.00112803773905,
58.0581058447233));
#65479=CARTESIAN_POINT('Ctrl Pts',(3.49633757827368,-3.80495436405849,58.2168666069693));
#65480=CARTESIAN_POINT('Ctrl Pts',(5.09301729854088,0.873629767452735,58.3756273692151));
#65481=CARTESIAN_POINT('Ctrl Pts',(2.02841201894453,4.75264125042254,58.5343881314611));
#65482=CARTESIAN_POINT('Ctrl Pts',(-2.89265789904175,4.2818902896884,58.6931488937069));
#65483=CARTESIAN_POINT('Ctrl Pts',(-5.16627895043901,-0.107777456210482,
58.8519096559528));
#65484=CARTESIAN_POINT('Ctrl Pts',(-2.71156370034918,-4.39880398208026,
59.0106704181988));
#65485=CARTESIAN_POINT('Ctrl Pts',(2.22485747409188,-4.66391074033302,59.1694311804446));
#65486=CARTESIAN_POINT('Ctrl Pts',(5.12502112908765,-0.660463928024547,
59.3281919426906));
#65487=CARTESIAN_POINT('Ctrl Pts',(3.33460890093368,3.94745964534539,59.4869527049363));
#65488=CARTESIAN_POINT('Ctrl Pts',(-1.5077392503099,4.94254757457034,59.6457134671823));
#65489=CARTESIAN_POINT('Ctrl Pts',(-4.97015838517481,1.41406499146713,59.8044742294282));
#65490=CARTESIAN_POINT('Ctrl Pts',(-3.88373675046313,-3.40861306500439,
59.963234991674));
#65491=CARTESIAN_POINT('Ctrl Pts',(0.757199388556149,-5.11162432694214,
60.12199575392));
#65492=CARTESIAN_POINT('Ctrl Pts',(4.70512351821232,-2.13632086826434,60.2807565161658));
#65493=CARTESIAN_POINT('Ctrl Pts',(4.34677488413138,2.79420870381954,60.4395172784118));
#65494=CARTESIAN_POINT('Ctrl Pts',(0.0101251021257834,5.16739311995163,
60.5982780406576));
#65495=CARTESIAN_POINT('Ctrl Pts',(-4.33579148262063,2.81122151262594,60.7570388029036));
#65496=CARTESIAN_POINT('Ctrl Pts',(-4.71345926399734,-2.11786589293417,
60.9157995651493));
#65497=CARTESIAN_POINT('Ctrl Pts',(-0.777225152475865,-5.10861774222493,
61.0745603273954));
#65498=CARTESIAN_POINT('Ctrl Pts',(3.87034915924295,-3.42380658907068,61.2333210896411));
#65499=CARTESIAN_POINT('Ctrl Pts',(4.97566169906822,1.39457693593507,61.3920818518871));
#65500=CARTESIAN_POINT('Ctrl Pts',(1.52709666834069,4.93660105126586,61.550842614133));
#65501=CARTESIAN_POINT('Ctrl Pts',(-3.3191138790273,3.96049709403562,61.7096033763789));
#65502=CARTESIAN_POINT('Ctrl Pts',(-5.12757002065602,-0.640374778614905,
61.8683641386248));
#65503=CARTESIAN_POINT('Ctrl Pts',(-2.24311745571471,-4.65515609337478,
62.0271249008706));
#65504=CARTESIAN_POINT('Ctrl Pts',(2.69430472161155,-4.40939635788372,62.1858856631165));
#65505=CARTESIAN_POINT('Ctrl Pts',(5.16581691910958,-0.128022388891978,
62.3446464253625));
#65506=CARTESIAN_POINT('Ctrl Pts',(2.90941568030617,4.27052158090844,62.5034071876082));
#65507=CARTESIAN_POINT('Ctrl Pts',(-2.00977165837252,4.76055375508134,62.6621679498542));
#65508=CARTESIAN_POINT('Ctrl Pts',(-5.08955458603407,0.893581719595941,
62.8209287121001));
#65509=CARTESIAN_POINT('Ctrl Pts',(-3.51122169408817,-3.79122360047265,
62.9796894743459));
#65510=CARTESIAN_POINT('Ctrl Pts',(1.28068854395033,-5.00618527695598,63.1384502365919));
#65511=CARTESIAN_POINT('Ctrl Pts',(4.90047350742458,-1.63933327204883,63.2972109988377));
#65512=CARTESIAN_POINT('Ctrl Pts',(4.03519542999152,3.22788661752423,63.4559717610837));
#65513=CARTESIAN_POINT('Ctrl Pts',(-0.523216761619089,5.14084607765855,
63.6147325233295));
#65514=CARTESIAN_POINT('Ctrl Pts',(-4.60276499113179,2.34874617833169,63.7734932855755));
#65515=CARTESIAN_POINT('Ctrl Pts',(-4.46972210747346,-2.59299796679048,
63.9322540478212));
#65516=CARTESIAN_POINT('Ctrl Pts',(-0.245853021615901,-5.16155116855183,
64.0910148100673));
#65517=CARTESIAN_POINT('Ctrl Pts',(4.20302825930282,-3.00609507922124,64.249775572313));
#65518=CARTESIAN_POINT('Ctrl Pts',(4.80516969413782,1.90063104898239,64.408536334559));
#65519=CARTESIAN_POINT('Ctrl Pts',(1.00947304907845,5.06784158562605,64.5672970968048));
#65520=CARTESIAN_POINT('Ctrl Pts',(-3.71012416525332,3.59680870386789,64.7260578590508));
#65521=CARTESIAN_POINT('Ctrl Pts',(-5.03410241632698,-1.16613336962256,
64.8848186212966));
#65522=CARTESIAN_POINT('Ctrl Pts',(-1.75071636731768,-4.86179456322688,
65.0435793835425));
#65523=CARTESIAN_POINT('Ctrl Pts',(3.1349787773885,-4.10779286711735,65.2023401457884));
#65524=CARTESIAN_POINT('Ctrl Pts',(5.15144558585509,0.405786335144852,65.3611009080343));
#65525=CARTESIAN_POINT('Ctrl Pts',(2.45315204119292,4.54797748857745,65.5198616702802));
#65526=CARTESIAN_POINT('Ctrl Pts',(-2.49034118407384,4.52772072468283,65.6786224325261));
#65527=CARTESIAN_POINT('Ctrl Pts',(-5.15459808921429,0.363555652528053,
65.837383194772));
#65528=CARTESIAN_POINT('Ctrl Pts',(-3.10120937385697,-4.13334665777235,
65.9961439570178));
#65529=CARTESIAN_POINT('Ctrl Pts',(1.79050088812788,-4.84728385216189,66.1549047192638));
#65530=CARTESIAN_POINT('Ctrl Pts',(5.04349004573647,-1.12483880283976,66.3136654815096));
#65531=CARTESIAN_POINT('Ctrl Pts',(3.68052305807757,3.62709307749002,66.4724262437556));
#65532=CARTESIAN_POINT('Ctrl Pts',(-1.05097105537457,5.05939858230018,66.6311870060014));
#65533=CARTESIAN_POINT('Ctrl Pts',(-4.82058435661895,1.86118796324735,66.7899477682473));
#65534=CARTESIAN_POINT('Ctrl Pts',(-4.17825160801934,-3.04043873049599,
66.9487085304932));
#65535=CARTESIAN_POINT('Ctrl Pts',(0.288144638596748,-5.15936302667923,
67.1074692927391));
#65536=CARTESIAN_POINT('Ctrl Pts',(4.49082211047655,-2.55628068604989,67.266230054985));
#65537=CARTESIAN_POINT('Ctrl Pts',(4.58336201290063,2.38638782106256,67.4249908172308));
#65538=CARTESIAN_POINT('Ctrl Pts',(0.481069000502546,5.14496130117338,67.5837515794768));
#65539=CARTESIAN_POINT('Ctrl Pts',(-4.06151305559941,3.19470904356121,67.7425123417227));
#65540=CARTESIAN_POINT('Ctrl Pts',(-4.88687430268524,-1.67943851437657,
67.9012731039685));
#65541=CARTESIAN_POINT('Ctrl Pts',(-1.23961891643423,-5.01651264483955,
68.0600338662145));
#65542=CARTESIAN_POINT('Ctrl Pts',(3.54217356679019,-3.76232117137135,68.2187946284603));
#65543=CARTESIAN_POINT('Ctrl Pts',(5.08206060458778,0.935261559732356,68.3775553907062));
#65544=CARTESIAN_POINT('Ctrl Pts',(1.97069054350433,4.77686434343271,68.5363161529522));
#65545=CARTESIAN_POINT('Ctrl Pts',(-2.9443156985208,4.2465349688023,68.695076915198));
#65546=CARTESIAN_POINT('Ctrl Pts',(-5.16459427796565,-0.170352921375672,
68.8538376774439));
#65547=CARTESIAN_POINT('Ctrl Pts',(-2.65807841962993,-4.43132861441282,
69.0125984396897));
#65548=CARTESIAN_POINT('Ctrl Pts',(2.2811920004135,-4.63661700284439,69.1713592019357));
#65549=CARTESIAN_POINT('Ctrl Pts',(5.1326458217616,-0.598331882962418,69.3301199641815));
#65550=CARTESIAN_POINT('Ctrl Pts',(3.28654540832559,3.98756485249208,69.4888807264275));
#65551=CARTESIAN_POINT('Ctrl Pts',(-1.56750175164667,4.92392043319156,69.6476414886732));
#65552=CARTESIAN_POINT('Ctrl Pts',(-4.98692342854749,1.35375363032602,69.8064022509193));
#65553=CARTESIAN_POINT('Ctrl Pts',(-3.84216045608199,-3.45540984595692,
69.965163013165));
#65554=CARTESIAN_POINT('Ctrl Pts',(0.819065126108891,-5.102076684352,70.1239237754111));
#65555=CARTESIAN_POINT('Ctrl Pts',(4.73065728621489,-2.07916709626671,70.2826845376568));
#65556=CARTESIAN_POINT('Ctrl Pts',(4.31260739816882,2.84665972730784,70.4414452999028));
#65557=CARTESIAN_POINT('Ctrl Pts',(-0.0524725109896868,5.16713661609669,
70.6002060621488));
#65558=CARTESIAN_POINT('Ctrl Pts',(-4.36952797529665,2.75849224159072,70.7589668243945));
#65559=CARTESIAN_POINT('Ctrl Pts',(-4.68745796764224,-2.17480849166161,
70.9177275866405));
#65560=CARTESIAN_POINT('Ctrl Pts',(-0.715283247733823,-5.11765806295492,
71.0764883488864));
#65561=CARTESIAN_POINT('Ctrl Pts',(3.91154054911197,-3.37667065413102,71.2352491111322));
#65562=CARTESIAN_POINT('Ctrl Pts',(4.95840295584866,1.45474887910182,71.3940098733782));
#65563=CARTESIAN_POINT('Ctrl Pts',(1.46718352100222,4.95473780229749,71.552770635624));
#65564=CARTESIAN_POINT('Ctrl Pts',(-3.36684708796952,3.91999934439373,71.7115313978699));
#65565=CARTESIAN_POINT('Ctrl Pts',(-5.11943640034826,-0.702442251438138,
71.8702921601158));
#65566=CARTESIAN_POINT('Ctrl Pts',(-2.18656114390733,-4.68198724237597,
72.0290529223616));
#65567=CARTESIAN_POINT('Ctrl Pts',(2.74752166081747,-4.3764344959288,72.1878136846077));
#65568=CARTESIAN_POINT('Ctrl Pts',(5.16698871742013,-0.0654352188752399,
72.3465744468534));
#65569=CARTESIAN_POINT('Ctrl Pts',(2.85746987211454,4.30545236923763,72.5053352090995));
#65570=CARTESIAN_POINT('Ctrl Pts',(-2.06729268270395,4.73585843726931,72.6640959713451));
#65571=CARTESIAN_POINT('Ctrl Pts',(-5.10000582803462,0.831862204832684,
72.8228567335913));
#65572=CARTESIAN_POINT('Ctrl Pts',(-3.46503785784167,-3.83347972702879,
72.9816174958369));
#65573=CARTESIAN_POINT('Ctrl Pts',(1.34123860080759,-4.99030391755056,73.140378258083));
#65574=CARTESIAN_POINT('Ctrl Pts',(4.91997252333115,-1.57984953191204,73.2991390203287));
#65575=CARTESIAN_POINT('Ctrl Pts',(3.99579730998455,3.27653140246455,73.4578997825747));
#65576=CARTESIAN_POINT('Ctrl Pts',(-0.585453654677876,5.13413071435083,
73.6166605448206));
#65577=CARTESIAN_POINT('Ctrl Pts',(-4.63087955166449,2.29281677239862,73.7754213070665));
#65578=CARTESIAN_POINT('Ctrl Pts',(-4.43798303090997,-2.64695311465312,
73.9341820693124));
#65579=CARTESIAN_POINT('Ctrl Pts',(-0.183308880309829,-5.16415065893858,
74.0929428315583));
#65580=CARTESIAN_POINT('Ctrl Pts',(4.23913515679244,-2.95495977912772,74.2517035938041));
#65581=CARTESIAN_POINT('Ctrl Pts',(4.78179321232898,1.95870055096247,74.4104643560501));
#65582=CARTESIAN_POINT('Ctrl Pts',(0.948008058166557,5.07969830752458,74.5692251182959));
#65583=CARTESIAN_POINT('Ctrl Pts',(-3.75342302811316,3.55160101163497,74.7279858805418));
#65584=CARTESIAN_POINT('Ctrl Pts',(-5.01960670926438,-1.22703001516843,
74.8867466427878));
#65585=CARTESIAN_POINT('Ctrl Pts',(-1.69169300421356,-4.88264569196979,
75.0455074050335));
#65586=CARTESIAN_POINT('Ctrl Pts',(3.18450981172911,-4.06951488912588,75.2042681672795));
#65587=CARTESIAN_POINT('Ctrl Pts',(5.14615197585861,0.468160245196775,75.3630289295254));
#65588=CARTESIAN_POINT('Ctrl Pts',(2.39787866042351,4.57736082297456,75.5217896917712));
#65589=CARTESIAN_POINT('Ctrl Pts',(-2.54500644918866,4.49722095825909,75.6805504540172));
#65590=CARTESIAN_POINT('Ctrl Pts',(-5.15862391826907,0.301087103142032,
75.839311216263));
#65591=CARTESIAN_POINT('Ctrl Pts',(-3.05091120513038,-4.17061086559584,
75.9980719785089));
#65592=CARTESIAN_POINT('Ctrl Pts',(1.84908863423975,-4.82523837717284,76.1568327407549));
#65593=CARTESIAN_POINT('Ctrl Pts',(5.05674607440601,-1.06366033713594,76.3155935030006));
#65594=CARTESIAN_POINT('Ctrl Pts',(3.63631504695578,3.6714121333759,76.4743542652466));
#65595=CARTESIAN_POINT('Ctrl Pts',(-1.11218258415778,5.04629607467818,76.6331150274925));
#65596=CARTESIAN_POINT('Ctrl Pts',(-4.84277674219067,1.80265570731443,76.7918757897383));
#65597=CARTESIAN_POINT('Ctrl Pts',(-4.1411137012291,-3.09083022621898,76.9506365519843));
#65598=CARTESIAN_POINT('Ctrl Pts',(0.350623091062388,-5.15549392607834,
77.1093973142301));
#65599=CARTESIAN_POINT('Ctrl Pts',(4.52145892049186,-2.50169210817825,77.268158076476));
#65600=CARTESIAN_POINT('Ctrl Pts',(4.55411743612604,2.44173474230699,77.4269188387219));
#65601=CARTESIAN_POINT('Ctrl Pts',(0.4187085668894,5.15041137287398,77.5856796009678));
#65602=CARTESIAN_POINT('Ctrl Pts',(-4.09991517238411,3.14527419362299,77.7444403632137));
#65603=CARTESIAN_POINT('Ctrl Pts',(-4.86617131235222,-1.738514001283,77.9032011254596));
#65604=CARTESIAN_POINT('Ctrl Pts',(-1.17875882811733,-5.03116107861318,
78.0619618877055));
#65605=CARTESIAN_POINT('Ctrl Pts',(3.58748974126774,-3.71913585798031,78.2207226499514));
#65606=CARTESIAN_POINT('Ctrl Pts',(5.07035811814355,0.996756102360001,78.3794834121972));
#65607=CARTESIAN_POINT('Ctrl Pts',(1.91267986918918,4.80038643150889,78.5382441744432));
#65608=CARTESIAN_POINT('Ctrl Pts',(-2.99554141961442,4.21055646882815,78.697004936689));
#65609=CARTESIAN_POINT('Ctrl Pts',(-5.16215170118294,-0.232903387246084,
78.855765698935));
#65610=CARTESIAN_POINT('Ctrl Pts',(-2.60420306585193,-4.46320294918618,
79.0145264611808));
#65611=CARTESIAN_POINT('Ctrl Pts',(2.33719176176521,-4.60864284172174,79.1732872234268));
#65612=CARTESIAN_POINT('Ctrl Pts',(5.13951729856278,-0.536112032685121,
79.3320479856725));
#65613=CARTESIAN_POINT('Ctrl Pts',(3.23799961511593,4.02708488442023,79.4908087479186));
#65614=CARTESIAN_POINT('Ctrl Pts',(-1.62703422207133,4.90457070639472,79.6495695101643));
#65615=CARTESIAN_POINT('Ctrl Pts',(-5.00295664081116,1.29324360581397,79.8083302724103));
#65616=CARTESIAN_POINT('Ctrl Pts',(-3.80002032458076,-3.5016995454484,79.9670910346561));
#65617=CARTESIAN_POINT('Ctrl Pts',(0.880810665839244,-5.09178031191025,
80.125851796902));
#65618=CARTESIAN_POINT('Ctrl Pts',(4.75549683016874,-2.02170820645871,80.2846125591479));
#65619=CARTESIAN_POINT('Ctrl Pts',(4.27780703699033,2.89869300342805,80.4433733213939));
#65620=CARTESIAN_POINT('Ctrl Pts',(-0.11506242376767,5.16612183484124,80.6021340836397));
#65621=CARTESIAN_POINT('Ctrl Pts',(-4.40262323964949,2.70535816177208,80.7608948458856));
#65622=CARTESIAN_POINT('Ctrl Pts',(-4.66076878675771,-2.23143193721207,
80.9196556081315));
#65623=CARTESIAN_POINT('Ctrl Pts',(-0.653236375128765,-5.12594736724498,
81.0784163703773));
#65624=CARTESIAN_POINT('Ctrl Pts',(3.95215792026738,-3.32903919274863,81.2371771326234));
#65625=CARTESIAN_POINT('Ctrl Pts',(4.94041656702063,1.51470733791976,81.3959378948691));
#65626=CARTESIAN_POINT('Ctrl Pts',(1.40705506422376,4.97214744531344,81.5546986571151));
#65627=CARTESIAN_POINT('Ctrl Pts',(-3.41408621159557,3.87892633505682,81.713459419361));
#65628=CARTESIAN_POINT('Ctrl Pts',(-5.11055150349599,-0.76440664139103,
81.8722201816067));
#65629=CARTESIAN_POINT('Ctrl Pts',(-2.12968395259116,-4.7081313086182,82.0309809438528));
#65630=CARTESIAN_POINT('Ctrl Pts',(2.80033539806548,-4.3428303941221,82.1897417060986));
#65631=CARTESIAN_POINT('Ctrl Pts',(5.16740226597732,-0.00283844241944707,
82.3485024683445));
#65632=CARTESIAN_POINT('Ctrl Pts',(2.80510471878759,4.33975132503298,82.5072632305904));
#65633=CARTESIAN_POINT('Ctrl Pts',(-2.12451031000386,4.71046814615349,82.6660239928362));
#65634=CARTESIAN_POINT('Ctrl Pts',(-5.10970868581842,0.770020587436124,
82.8247847550823));
#65635=CARTESIAN_POINT('Ctrl Pts',(-3.41834544728425,-3.87517323895607,
82.983545517328));
#65636=CARTESIAN_POINT('Ctrl Pts',(1.40159167776471,-4.9736903294079,83.142306279574));
#65637=CARTESIAN_POINT('Ctrl Pts',(4.93874982643145,-1.52013376024582,83.3010670418199));
#65638=CARTESIAN_POINT('Ctrl Pts',(3.95581224496304,3.32469499516411,83.4598278040656));
#65639=CARTESIAN_POINT('Ctrl Pts',(-0.647603556591826,5.12666260907039,
83.6185885663118));
#65640=CARTESIAN_POINT('Ctrl Pts',(-4.65831659106839,2.23654957051732,83.7773493285574));
#65641=CARTESIAN_POINT('Ctrl Pts',(-4.40558873364168,-2.70051728419629,
83.9361100908035));
#65642=CARTESIAN_POINT('Ctrl Pts',(-0.120745397495975,-5.1659971710397,
84.0948708530492));
#65643=CARTESIAN_POINT('Ctrl Pts',(4.27463443926266,-2.90338152834273,84.2536316152952));
#65644=CARTESIAN_POINT('Ctrl Pts',(4.75768727179541,2.01646478129229,84.412392377541));
#65645=CARTESIAN_POINT('Ctrl Pts',(0.886457060193665,5.09084373843816,84.571153139787));
#65646=CARTESIAN_POINT('Ctrl Pts',(-3.79627280569434,3.50580670373394,84.7299139020329));
#65647=CARTESIAN_POINT('Ctrl Pts',(-5.00417952636703,-1.28762129421282,
84.8886746642788));
#65648=CARTESIAN_POINT('Ctrl Pts',(-1.63279460579437,-4.90302030367583,
85.0474354265246));
#65649=CARTESIAN_POINT('Ctrl Pts',(3.23428855022947,-4.03017982392474,85.2061961887705));
#65650=CARTESIAN_POINT('Ctrl Pts',(5.13873193725801,0.529582954402255,85.3649569510164));
#65651=CARTESIAN_POINT('Ctrl Pts',(2.34489518331184,4.6077777382683,85.5237177132623));
#65652=CARTESIAN_POINT('Ctrl Pts',(-2.60449736313211,4.46265913321349,85.6824784755082));
#65653=CARTESIAN_POINT('Ctrl Pts',(-4.72633661207834,0.94905134843793,85.8147791107131));
#65654=CARTESIAN_POINT('Ctrl Pts',(-4.08944266318188,-1.99447502555823,
85.9206196188771));
#65655=CARTESIAN_POINT('Ctrl Pts',(-3.130164636136,-3.13763950664809,85.973539872959));
#65656=CARTESIAN_POINT('Ctrl Pts',(-2.53835875722777,-3.5596515025498,86.));
#65657=CARTESIAN_POINT('Ctrl Pts',(-2.00237954638818,4.09906332620103,25.7806068977079));
#65658=CARTESIAN_POINT('Ctrl Pts',(-2.68386473467845,3.76615995447791,25.8070670247489));
#65659=CARTESIAN_POINT('Ctrl Pts',(-3.86722056834447,2.75399327045732,25.8599872788309));
#65660=CARTESIAN_POINT('Ctrl Pts',(-5.02742207131257,-0.166516440447624,
25.9658277869948));
#65661=CARTESIAN_POINT('Ctrl Pts',(-3.44586235178049,-4.14677665817345,
26.0981284221997));
#65662=CARTESIAN_POINT('Ctrl Pts',(1.62355296838563,-5.14470657330929,26.2568891844456));
#65663=CARTESIAN_POINT('Ctrl Pts',(5.19838240423087,-1.42611203276403,26.4156499466915));
#65664=CARTESIAN_POINT('Ctrl Pts',(4.01994424953236,3.59365933878956,26.5744107089374));
#65665=CARTESIAN_POINT('Ctrl Pts',(-0.839985566934964,5.3265048273725,26.7331714711833));
#65666=CARTESIAN_POINT('Ctrl Pts',(-4.92992667194028,2.18327469128225,26.8919322334291));
#65667=CARTESIAN_POINT('Ctrl Pts',(-4.50847904072441,-2.95758319158922,
27.050692995675));
#65668=CARTESIAN_POINT('Ctrl Pts',(0.0395956222711487,-5.39186919347605,
27.2094537579209));
#65669=CARTESIAN_POINT('Ctrl Pts',(4.55125923496193,-2.89119591637671,27.3682145201668));
#65670=CARTESIAN_POINT('Ctrl Pts',(4.89756113932563,2.25550678246132,27.5269752824127));
#65671=CARTESIAN_POINT('Ctrl Pts',(0.761418625289898,5.33794327443822,27.6857360446586));
#65672=CARTESIAN_POINT('Ctrl Pts',(-4.07157300373756,3.53490884489523,27.8444968069045));
#65673=CARTESIAN_POINT('Ctrl Pts',(-5.17814942709716,-1.503370550728,28.0032575691504));
#65674=CARTESIAN_POINT('Ctrl Pts',(-1.54551865619794,-5.1657253452884,28.1620183313962));
#65675=CARTESIAN_POINT('Ctrl Pts',(3.50161451494142,-4.10024735702302,28.3207790936422));
#65676=CARTESIAN_POINT('Ctrl Pts',(5.34396494196453,0.717900607442646,28.479539855888));
#65677=CARTESIAN_POINT('Ctrl Pts',(2.29535447129834,4.8790048681726,28.6383006181339));
#65678=CARTESIAN_POINT('Ctrl Pts',(-2.85403402839988,4.57469439300441,28.7970613803798));
#65679=CARTESIAN_POINT('Ctrl Pts',(-5.391323666464,0.0834841081329312,28.9558221426257));
#65680=CARTESIAN_POINT('Ctrl Pts',(-2.99430906975439,-4.48413350506007,
29.1145829048716));
#65681=CARTESIAN_POINT('Ctrl Pts',(2.14318857941972,-4.94773510082165,29.2733436671175));
#65682=CARTESIAN_POINT('Ctrl Pts',(5.31917461298845,-0.88301843516797,29.4321044293634));
#65683=CARTESIAN_POINT('Ctrl Pts',(3.62688954521853,3.98986369193538,29.5908651916093));
#65684=CARTESIAN_POINT('Ctrl Pts',(-1.3848356090803,5.21110068710349,29.7496259538552));
#65685=CARTESIAN_POINT('Ctrl Pts',(-5.12911691883564,1.66297916304394,29.9083867161011));
#65686=CARTESIAN_POINT('Ctrl Pts',(-4.17907375081987,-3.40715168987467,
30.0671474783469));
#65687=CARTESIAN_POINT('Ctrl Pts',(0.595785363987352,-5.35895324212101,
30.2259082405928));
#65688=CARTESIAN_POINT('Ctrl Pts',(4.82536351591838,-2.40607709649645,30.3846690028387));
#65689=CARTESIAN_POINT('Ctrl Pts',(4.63862158504372,2.74891430277669,30.5434297650846));
#65690=CARTESIAN_POINT('Ctrl Pts',(0.206471491199163,5.38801536528353,30.7021905273305));
#65691=CARTESIAN_POINT('Ctrl Pts',(-4.41464761825083,3.09584018650688,30.8609512895764));
#65692=CARTESIAN_POINT('Ctrl Pts',(-4.99534638025495,-2.02974249468088,
31.0197120518223));
#65693=CARTESIAN_POINT('Ctrl Pts',(-1.00415155023673,-5.29764284541871,
31.1784728140681));
#65694=CARTESIAN_POINT('Ctrl Pts',(3.90607345078174,-3.71697864543531,31.3372335763141));
#65695=CARTESIAN_POINT('Ctrl Pts',(5.24134071706976,1.26557794744869,31.4959943385599));
#65696=CARTESIAN_POINT('Ctrl Pts',(1.77957286026287,5.08983894524214,31.6547551008058));
#65697=CARTESIAN_POINT('Ctrl Pts',(-3.31091443601954,4.25572386919705,31.8135158630518));
#65698=CARTESIAN_POINT('Ctrl Pts',(-5.37115170725749,-0.473359684716424,
31.9722766252976));
#65699=CARTESIAN_POINT('Ctrl Pts',(-2.51554687204882,-4.76920999621703,
32.1310373875435));
#65700=CARTESIAN_POINT('Ctrl Pts',(2.6423632988389,-4.70013364176394,32.2897981497894));
#65701=CARTESIAN_POINT('Ctrl Pts',(5.38190186659124,-0.329351410916935,
32.4485589120353));
#65702=CARTESIAN_POINT('Ctrl Pts',(3.19575945370633,4.34286329137105,32.6073196742812));
#65703=CARTESIAN_POINT('Ctrl Pts',(-1.91523962695419,5.04035685490976,32.7660804365271));
#65704=CARTESIAN_POINT('Ctrl Pts',(-5.27335289927007,1.12476186513028,32.9248411987729));
#65705=CARTESIAN_POINT('Ctrl Pts',(-3.80513252151237,-3.82024953991496,
33.0836019610189));
#65706=CARTESIAN_POINT('Ctrl Pts',(1.14566136921973,-5.26885187498842,33.2423627232647));
#65707=CARTESIAN_POINT('Ctrl Pts',(5.04791098015974,-1.89524003489642,33.4011234855106));
#65708=CARTESIAN_POINT('Ctrl Pts',(4.330158271609,3.21295337599341,33.5598842477565));
#65709=CARTESIAN_POINT('Ctrl Pts',(-0.350687553524876,5.38055371623537,
33.7186450100024));
#65710=CARTESIAN_POINT('Ctrl Pts',(-4.71057341778202,2.62370694422547,33.8774057722483));
#65711=CARTESIAN_POINT('Ctrl Pts',(-4.75919860374648,-2.53443656531169,
34.0361665344942));
#65712=CARTESIAN_POINT('Ctrl Pts',(-0.452059855948003,-5.3729863149027,
34.19492729674));
#65713=CARTESIAN_POINT('Ctrl Pts',(4.2688178803622,-3.29401486909083,34.353688058986));
#65714=CARTESIAN_POINT('Ctrl Pts',(5.08274309982495,1.79973960190727,34.5124488212318));
#65715=CARTESIAN_POINT('Ctrl Pts',(1.2447865799184,5.24631741547787,34.6712095834778));
#65716=CARTESIAN_POINT('Ctrl Pts',(-3.73243664043062,3.89130527955111,34.8299703457236));
#65717=CARTESIAN_POINT('Ctrl Pts',(-5.2936198386959,-1.02514830968824,34.9887311079695));
#65718=CARTESIAN_POINT('Ctrl Pts',(-2.00992046486332,-5.00335485233809,
35.1474918702154));
#65719=CARTESIAN_POINT('Ctrl Pts',(3.11331951223216,-4.40233820466419,35.3062526324613));
#65720=CARTESIAN_POINT('Ctrl Pts',(5.38715437415002,0.227832839089729,35.4650133947072));
#65721=CARTESIAN_POINT('Ctrl Pts',(2.73050100007286,4.64948430926405,35.6237741569531));
#65722=CARTESIAN_POINT('Ctrl Pts',(-2.42519029351004,4.81578571925249,35.782534919199));
#65723=CARTESIAN_POINT('Ctrl Pts',(-5.36127335207045,0.574532938890892,
35.9412956814449));
#65724=CARTESIAN_POINT('Ctrl Pts',(-3.39055527658917,-4.19254993648074,
36.1000564436907));
#65725=CARTESIAN_POINT('Ctrl Pts',(1.68330255388594,-5.12248304687996,36.2588172059367));
#65726=CARTESIAN_POINT('Ctrl Pts',(5.21655046989866,-1.36416320449261,36.4175779681825));
#65727=CARTESIAN_POINT('Ctrl Pts',(3.97545205425126,3.64268047155399,36.5763387304284));
#65728=CARTESIAN_POINT('Ctrl Pts',(-0.904101513210989,5.31563171291061,
36.7350994926743));
#65729=CARTESIAN_POINT('Ctrl Pts',(-4.95619375964226,2.12355444252664,36.8938602549202));
#65730=CARTESIAN_POINT('Ctrl Pts',(-4.47222608833935,-3.01206471847277,
37.0526210171661));
#65731=CARTESIAN_POINT('Ctrl Pts',(0.10485950493631,-5.39095024441108,37.211381779412));
#65732=CARTESIAN_POINT('Ctrl Pts',(4.58597447631896,-2.83587343794507,37.3701425416579));
#65733=CARTESIAN_POINT('Ctrl Pts',(4.8698655265602,2.31468136181031,37.5289033039037));
#65734=CARTESIAN_POINT('Ctrl Pts',(0.696706894914159,5.34676907637412,37.6876640661497));
#65735=CARTESIAN_POINT('Ctrl Pts',(-4.1140991681465,3.48533041305234,37.8464248283955));
#65736=CARTESIAN_POINT('Ctrl Pts',(-5.15955600572413,-1.56598910509857,
38.0051855906414));
#65737=CARTESIAN_POINT('Ctrl Pts',(-1.48282958617279,-5.18406756050325,
38.1639463528873));
#65738=CARTESIAN_POINT('Ctrl Pts',(3.55102776426338,-4.05752903512989,38.3227071151332));
#65739=CARTESIAN_POINT('Ctrl Pts',(5.33487603729029,0.782584002032494,38.4814678773791));
#65740=CARTESIAN_POINT('Ctrl Pts',(2.23608280507879,4.90645225619513,38.640228639625));
#65741=CARTESIAN_POINT('Ctrl Pts',(-2.90924171237944,4.53978553595244,38.7989894018709));
#65742=CARTESIAN_POINT('Ctrl Pts',(-5.39193935072285,0.0181684236512802,
38.9577501641167));
#65743=CARTESIAN_POINT('Ctrl Pts',(-2.93976939635272,-4.52007698493724,
39.1165109263627));
#65744=CARTESIAN_POINT('Ctrl Pts',(2.20296730598482,-4.92140986936197,39.2752716886085));
#65745=CARTESIAN_POINT('Ctrl Pts',(5.32948103937253,-0.818518114924823,
39.4340324508545));
#65746=CARTESIAN_POINT('Ctrl Pts',(3.5782909344085,4.03350642025291,39.5927932131003));
#65747=CARTESIAN_POINT('Ctrl Pts',(-1.44786033404595,5.19394267455733,39.7515539753462));
#65748=CARTESIAN_POINT('Ctrl Pts',(-5.14888559931178,1.60072394206216,39.9103147375921));
#65749=CARTESIAN_POINT('Ctrl Pts',(-4.13749348932905,-3.45752623695775,
40.069075499838));
#65750=CARTESIAN_POINT('Ctrl Pts',(0.660659043471872,-5.3513427923999,40.2278362620838));
#65751=CARTESIAN_POINT('Ctrl Pts',(4.85415623959407,-2.3474469653437,40.3865970243298));
#65752=CARTESIAN_POINT('Ctrl Pts',(4.60498137310684,2.80490402809622,40.5453577865757));
#65753=CARTESIAN_POINT('Ctrl Pts',(0.141186892964701,5.39012117811339,40.7041185488216));
#65754=CARTESIAN_POINT('Ctrl Pts',(-4.45182614422856,3.04213478252601,40.8628793110674));
#65755=CARTESIAN_POINT('Ctrl Pts',(-4.97039191142365,-2.09010628924604,
41.0216400733134));
#65756=CARTESIAN_POINT('Ctrl Pts',(-0.939903178686041,-5.30941824197221,
41.1804008355592));
#65757=CARTESIAN_POINT('Ctrl Pts',(3.95081365290143,-3.66938844135355,41.3391615978052));
#65758=CARTESIAN_POINT('Ctrl Pts',(5.22562515017917,1.32897774372121,41.497922360051));
#65759=CARTESIAN_POINT('Ctrl Pts',(1.71778489121437,5.11102290358859,41.6566831222969));
#65760=CARTESIAN_POINT('Ctrl Pts',(-3.36222457061253,4.21530378386431,41.8154438845428));
#65761=CARTESIAN_POINT('Ctrl Pts',(-5.36502340492809,-0.538390116983158,
41.9742046467887));
#65762=CARTESIAN_POINT('Ctrl Pts',(-2.4575889422798,-4.7993329374274,42.1329654090346));
#65763=CARTESIAN_POINT('Ctrl Pts',(2.69910598837468,-4.66777965600471,42.2917261712804));
#65764=CARTESIAN_POINT('Ctrl Pts',(5.38549667320271,-0.26413185422043,42.4504869335264));
#65765=CARTESIAN_POINT('Ctrl Pts',(3.14291630057783,4.38125748855891,42.6092476957722));
#65766=CARTESIAN_POINT('Ctrl Pts',(-1.97615707196429,5.01678615055665,42.7680084580181));
#65767=CARTESIAN_POINT('Ctrl Pts',(-5.28659112974097,1.06079888783667,42.926769220264));
#65768=CARTESIAN_POINT('Ctrl Pts',(-3.75857550455005,-3.86606391955536,
43.0855299825098));
#65769=CARTESIAN_POINT('Ctrl Pts',(1.20940322958872,-5.25458693731027,43.2442907447559));
#65770=CARTESIAN_POINT('Ctrl Pts',(5.07049918630525,-1.83395148659098,43.4030515070016));
#65771=CARTESIAN_POINT('Ctrl Pts',(4.29091940730092,3.26517238343396,43.5618122692476));
#65772=CARTESIAN_POINT('Ctrl Pts',(-0.41584088110511,5.37591075215103,43.7205730314935));
#65773=CARTESIAN_POINT('Ctrl Pts',(-4.74201089309862,2.56645139116746,43.8793337937394));
#65774=CARTESIAN_POINT('Ctrl Pts',(-4.72814768911957,-2.59190267629106,
44.0380945559852));
#65775=CARTESIAN_POINT('Ctrl Pts',(-0.386939296906612,-5.3780682437099,
44.1968553182311));
#65776=CARTESIAN_POINT('Ctrl Pts',(4.30840775904998,-3.24206147925195,44.3556160804771));
#65777=CARTESIAN_POINT('Ctrl Pts',(5.06056843189549,1.86117898107469,44.5143768427229));
#65778=CARTESIAN_POINT('Ctrl Pts',(1.18114229879479,5.26101158746959,44.6731376049688));
#65779=CARTESIAN_POINT('Ctrl Pts',(-3.77930134462421,3.84580568932092,44.8318983672147));
#65780=CARTESIAN_POINT('Ctrl Pts',(-5.2808129571804,-1.08919904735859,44.9906591294605));
#65781=CARTESIAN_POINT('Ctrl Pts',(-1.94916324679306,-5.02733554587743,
45.1494198917065));
#65782=CARTESIAN_POINT('Ctrl Pts',(3.16642020502591,-4.36430099084551,45.3081806539524));
#65783=CARTESIAN_POINT('Ctrl Pts',(5.38399916564066,0.293075140317788,45.4669414161982));
#65784=CARTESIAN_POINT('Ctrl Pts',(2.67397763346517,4.68221995096551,45.6257021784443));
#65785=CARTESIAN_POINT('Ctrl Pts',(-2.48334990656791,4.78605404221895,45.7844629406899));
#65786=CARTESIAN_POINT('Ctrl Pts',(-5.3678397571995,0.509545282109415,45.9432237029359));
#65787=CARTESIAN_POINT('Ctrl Pts',(-3.3395186992418,-4.23331488444999,46.1019844651818));
#65788=CARTESIAN_POINT('Ctrl Pts',(1.74523187918884,-5.10171596047391,46.2607452274276));
#65789=CARTESIAN_POINT('Ctrl Pts',(5.232692932984,-1.30087075552908,46.4195059896737));
#65790=CARTESIAN_POINT('Ctrl Pts',(3.93103357982541,3.69057110049061,46.5782667519194));
#65791=CARTESIAN_POINT('Ctrl Pts',(-0.96842778057353,5.30428955537918,46.7370275141654));
#65792=CARTESIAN_POINT('Ctrl Pts',(-4.98155445517987,2.06336018755066,46.8957882764112));
#65793=CARTESIAN_POINT('Ctrl Pts',(-4.43541032884349,-3.06601945008181,
47.0545490386572));
#65794=CARTESIAN_POINT('Ctrl Pts',(0.170156811823045,-5.3892844342159,47.213309800903));
#65795=CARTESIAN_POINT('Ctrl Pts',(4.61999124080161,-2.78011168631907,47.3720705631489));
#65796=CARTESIAN_POINT('Ctrl Pts',(4.8414685667286,2.37350419651411,47.5308313253948));
#65797=CARTESIAN_POINT('Ctrl Pts',(0.631885975802691,5.35481653906792,47.6895920876407));
#65798=CARTESIAN_POINT('Ctrl Pts',(-4.15601796138632,3.43523722006585,47.8483528498866));
#65799=CARTESIAN_POINT('Ctrl Pts',(-5.14020731309298,-1.62837613342762,
48.0071136121325));
#65800=CARTESIAN_POINT('Ctrl Pts',(-1.41992192218023,-5.20164991021152,
48.1658743743783));
#65801=CARTESIAN_POINT('Ctrl Pts',(3.59991938399174,-4.01421480270452,48.3246351366243));
#65802=CARTESIAN_POINT('Ctrl Pts',(5.32500450896511,0.847152308025391,48.4833958988701));
#65803=CARTESIAN_POINT('Ctrl Pts',(2.17648285295299,4.93317974984624,48.642156661116));
#65804=CARTESIAN_POINT('Ctrl Pts',(-2.96402239161607,4.50421039867032,48.800917423362));
#65805=CARTESIAN_POINT('Ctrl Pts',(-5.39176380613531,-0.0471498922667038,
48.9596781856078));
#65806=CARTESIAN_POINT('Ctrl Pts',(-2.88479829170963,-4.55535716158905,
49.1184389478537));
#65807=CARTESIAN_POINT('Ctrl Pts',(2.26242273659985,-4.89436241142882,49.2771997100995));
#65808=CARTESIAN_POINT('Ctrl Pts',(5.33900536977086,-0.753897682082513,
49.4359604723455));
#65809=CARTESIAN_POINT('Ctrl Pts',(3.52916720648512,4.07655723401027,49.5947212345913));
#65810=CARTESIAN_POINT('Ctrl Pts',(-1.51067258399179,5.1760224494748,49.7534819968373));
#65811=CARTESIAN_POINT('Ctrl Pts',(-5.16789868150448,1.53823381551562,49.9122427590831));
#65812=CARTESIAN_POINT('Ctrl Pts',(-4.09530605018365,-3.5073933923671,50.0710035213291));
#65813=CARTESIAN_POINT('Ctrl Pts',(0.72543577101732,-5.34294703282935,50.2297642835748));
#65814=CARTESIAN_POINT('Ctrl Pts',(4.88223661585912,-2.28847234640404,50.3885250458209));
#65815=CARTESIAN_POINT('Ctrl Pts',(4.57066538000743,2.86048213374822,50.5472858080667));
#65816=CARTESIAN_POINT('Ctrl Pts',(0.0758815755810925,5.39143599052969,
50.7060465703126));
#65817=CARTESIAN_POINT('Ctrl Pts',(-4.48835136464999,2.98798294522175,50.8648073325585));
#65818=CARTESIAN_POINT('Ctrl Pts',(-4.94470803747584,-2.15016336068061,
51.0235680948044));
#65819=CARTESIAN_POINT('Ctrl Pts',(-0.875516876330153,-5.32041448129303,
51.1823288570502));
#65820=CARTESIAN_POINT('Ctrl Pts',(3.99497407304406,-3.62125975444968,51.3410896192962));
#65821=CARTESIAN_POINT('Ctrl Pts',(5.20914272269644,1.39218251248544,51.499850381542));
#65822=CARTESIAN_POINT('Ctrl Pts',(1.65574483720076,5.13145681922537,51.658611143788));
#65823=CARTESIAN_POINT('Ctrl Pts',(-3.41304129868565,4.17426510262078,51.8173719060338));
#65824=CARTESIAN_POINT('Ctrl Pts',(-5.35810778531101,-0.603341540490118,
51.9761326682797));
#65825=CARTESIAN_POINT('Ctrl Pts',(-2.39927036128639,-4.82875157643711,
52.1348934305256));
#65826=CARTESIAN_POINT('Ctrl Pts',(2.75545258405494,-4.6347406734915,52.2936541927715));
#65827=CARTESIAN_POINT('Ctrl Pts',(5.38830115807414,-0.198873536169234,
52.4524149550174));
#65828=CARTESIAN_POINT('Ctrl Pts',(3.08961192442195,4.41900873612634,52.6111757172633));
#65829=CARTESIAN_POINT('Ctrl Pts',(-2.03678451588621,4.99247923273975,52.7699364795092));
#65830=CARTESIAN_POINT('Ctrl Pts',(-5.29905355286222,0.996680238285941,
52.928697241755));
#65831=CARTESIAN_POINT('Ctrl Pts',(-3.71146691656038,-3.91131095424147,
53.087458004001));
#65832=CARTESIAN_POINT('Ctrl Pts',(1.27296761001063,-5.23955088889833,53.2462187662468));
#65833=CARTESIAN_POINT('Ctrl Pts',(5.09234329659795,-1.77239380586966,53.4049795284928));
#65834=CARTESIAN_POINT('Ctrl Pts',(4.25105085048754,3.31691222676463,53.5637402907385));
#65835=CARTESIAN_POINT('Ctrl Pts',(-0.48093318402806,5.37047887306077,53.7225010529846));
#65836=CARTESIAN_POINT('Ctrl Pts',(-4.77275247822576,2.50881921131856,53.8812618152303));
#65837=CARTESIAN_POINT('Ctrl Pts',(-4.69640291872861,-2.64898842550301,
54.0400225774763));
#65838=CARTESIAN_POINT('Ctrl Pts',(-0.321761954516003,-5.38236094089921,
54.1987833397221));
#65839=CARTESIAN_POINT('Ctrl Pts',(4.34736537881655,-3.18963231682882,54.3575441019682));
#65840=CARTESIAN_POINT('Ctrl Pts',(5.03765112545161,1.92234523219103,54.5163048642139));
#65841=CARTESIAN_POINT('Ctrl Pts',(1.11732468501616,5.27493370590994,54.6750656264599));
#65842=CARTESIAN_POINT('Ctrl Pts',(-3.82561143627296,3.79974172703212,54.8338263887057));
#65843=CARTESIAN_POINT('Ctrl Pts',(-5.26723111626224,-1.15308994504782,
54.9925871509516));
#65844=CARTESIAN_POINT('Ctrl Pts',(-1.88811998897897,-5.05057847782898,
55.1513479131975));
#65845=CARTESIAN_POINT('Ctrl Pts',(3.21905622559384,-4.32562331577277,55.3101086754434));
#65846=CARTESIAN_POINT('Ctrl Pts',(5.38005385515049,0.358274432763269,55.4688694376893));
#65847=CARTESIAN_POINT('Ctrl Pts',(2.61706186058861,4.71426847679935,55.6276301999351));
#65848=CARTESIAN_POINT('Ctrl Pts',(-2.54114508797937,4.75562001166302,55.7863909621812));
#65849=CARTESIAN_POINT('Ctrl Pts',(-5.37361843174121,0.444482849548049,
55.9451517244269));
#65850=CARTESIAN_POINT('Ctrl Pts',(-3.28799204746135,-4.27345859337873,
56.1039124866729));
#65851=CARTESIAN_POINT('Ctrl Pts',(1.80690509167997,-5.08020019715291,56.2626732489186));
#65852=CARTESIAN_POINT('Ctrl Pts',(5.24806749828111,-1.23738740375719,56.4214340111647));
#65853=CARTESIAN_POINT('Ctrl Pts',(3.88603822614634,3.73792013804749,56.5801947734104));
#65854=CARTESIAN_POINT('Ctrl Pts',(-1.03261193114073,5.2921689932538,56.7389555356565));
#65855=CARTESIAN_POINT('Ctrl Pts',(-5.00618410750568,2.00286313442759,56.8977162979023));
#65856=CARTESIAN_POINT('Ctrl Pts',(-4.3979436727968,-3.11952424327782,57.0564770601482));
#65857=CARTESIAN_POINT('Ctrl Pts',(0.235429148194338,-5.38682774642662,
57.2152378223941));
#65858=CARTESIAN_POINT('Ctrl Pts',(4.65333002148106,-2.72394195324985,57.37399858464));
#65859=CARTESIAN_POINT('Ctrl Pts',(4.81236112129208,2.43197871943155,57.5327593468858));
#65860=CARTESIAN_POINT('Ctrl Pts',(0.566972327412124,5.36207818233195,57.6915201091318));
#65861=CARTESIAN_POINT('Ctrl Pts',(-4.19732685891063,3.38463990595143,57.8502808713776));
#65862=CARTESIAN_POINT('Ctrl Pts',(-5.12010429494008,-1.6905241975279,58.0090416336235));
#65863=CARTESIAN_POINT('Ctrl Pts',(-1.35680588461835,-5.21846891769574,
58.1678023958695));
#65864=CARTESIAN_POINT('Ctrl Pts',(3.64828271548151,-3.97031148417985,58.3265631581153));
#65865=CARTESIAN_POINT('Ctrl Pts',(5.31435153612611,0.911596294400786,58.4853239203612));
#65866=CARTESIAN_POINT('Ctrl Pts',(2.11656350192684,4.95918329927446,58.6440846826071));
#65867=CARTESIAN_POINT('Ctrl Pts',(-3.01836810050987,4.46797426842589,58.8028454448529));
#65868=CARTESIAN_POINT('Ctrl Pts',(-5.39079702010585,-0.112461288937121,
58.9616062070989));
#65869=CARTESIAN_POINT('Ctrl Pts',(-2.8294038428619,-4.58996883949007,59.1203669693448));
#65870=CARTESIAN_POINT('Ctrl Pts',(2.32154615663493,-4.86659670571795,59.2791277315906));
#65871=CARTESIAN_POINT('Ctrl Pts',(5.34774620102881,-0.689166614740877,
59.4378884938366));
#65872=CARTESIAN_POINT('Ctrl Pts',(3.47952557320649,4.11900981291542,59.5966492560824));
#65873=CARTESIAN_POINT('Ctrl Pts',(-1.5732631427069,5.15734264299855,59.7554100183284));
#65874=CARTESIAN_POINT('Ctrl Pts',(-5.18615337446655,1.47551795312722,59.9141707805741));
#65875=CARTESIAN_POINT('Ctrl Pts',(-4.05251762479693,-3.55674583772888,
60.0729315428202));
#65876=CARTESIAN_POINT('Ctrl Pts',(0.790106040849496,-5.33376719567931,
60.2316923050659));
#65877=CARTESIAN_POINT('Ctrl Pts',(4.90960052380718,-2.22916189410365,60.3904530673119));
#65878=CARTESIAN_POINT('Ctrl Pts',(4.53567864167587,2.91564046359228,60.5492138295578));
#65879=CARTESIAN_POINT('Ctrl Pts',(0.0105651225747838,5.39195960961101,
60.7079745918036));
#65880=CARTESIAN_POINT('Ctrl Pts',(-4.52421791942263,2.93339262136295,60.8667353540496));
#65881=CARTESIAN_POINT('Ctrl Pts',(-4.91829852752871,-2.20990489560075,
61.0254961162954));
#65882=CARTESIAN_POINT('Ctrl Pts',(-0.811002091855911,-5.3306299496867,
61.1842568785414));
#65883=CARTESIAN_POINT('Ctrl Pts',(4.03854823066489,-3.57259964760746,61.3430176407872));
#65884=CARTESIAN_POINT('Ctrl Pts',(5.19189585341926,1.4551829784393,61.5017784030331));
#65885=CARTESIAN_POINT('Ctrl Pts',(1.5934618026005,5.15113769347555,61.660539165279));
#65886=CARTESIAN_POINT('Ctrl Pts',(-3.4633571628827,4.1326138478934,61.8192999275249));
#65887=CARTESIAN_POINT('Ctrl Pts',(-5.35040586327371,-0.668204423614378,
61.9780606897707));
#65888=CARTESIAN_POINT('Ctrl Pts',(-2.34059968732153,-4.85746159606041,
62.1368214520167));
#65889=CARTESIAN_POINT('Ctrl Pts',(2.81139481701569,-4.60102154269558,62.2955822142625));
#65890=CARTESIAN_POINT('Ctrl Pts',(5.39031490964729,-0.133586033422769,
62.4543429765085));
#65891=CARTESIAN_POINT('Ctrl Pts',(3.03585414765692,4.45611149407704,62.6131037387543));
#65892=CARTESIAN_POINT('Ctrl Pts',(-2.09711306164141,4.96743966849971,62.7718645010003));
#65893=CARTESIAN_POINT('Ctrl Pts',(-5.310738339773,0.932415325891086,62.930625263246));
#65894=CARTESIAN_POINT('Ctrl Pts',(-3.66381367072956,-3.95598400396999,
63.089386025492));
#65895=CARTESIAN_POINT('Ctrl Pts',(1.33634518241131,-5.223745936293,63.2481467877379));
#65896=CARTESIAN_POINT('Ctrl Pts',(5.11344010541426,-1.71057602632341,63.4069075499838));
#65897=CARTESIAN_POINT('Ctrl Pts',(4.21055845188033,3.36816531316245,63.5656683122297));
#65898=CARTESIAN_POINT('Ctrl Pts',(-0.545954909997053,5.36425887609291,
63.7244290744756));
#65899=CARTESIAN_POINT('Ctrl Pts',(-4.80279366183524,2.45081886220229,63.8831898367214));
#65900=CARTESIAN_POINT('Ctrl Pts',(-4.66396895111927,-2.70568543561274,
64.0419505989674));
#65901=CARTESIAN_POINT('Ctrl Pts',(-0.256537393552353,-5.38586377651727,
64.2007113612132));
#65902=CARTESIAN_POINT('Ctrl Pts',(4.38568502263036,-3.13673507580205,64.3594721234591));
#65903=CARTESIAN_POINT('Ctrl Pts',(5.01399454360851,1.98322937910761,64.5182328857051));
#65904=CARTESIAN_POINT('Ctrl Pts',(1.05334310381863,5.28808172772786,64.6769936479507));
#65905=CARTESIAN_POINT('Ctrl Pts',(-3.87136011937014,3.75312015257198,64.8357544101969));
#65906=CARTESIAN_POINT('Ctrl Pts',(-5.25287630907674,-1.21681162676554,
64.9945151724425));
#65907=CARTESIAN_POINT('Ctrl Pts',(-1.82679964952023,-5.07308023729216,
65.1532759346887));
#65908=CARTESIAN_POINT('Ctrl Pts',(3.27121984959904,-4.28631085539543,65.3120366969344));
#65909=CARTESIAN_POINT('Ctrl Pts',(5.3753190216539,0.423421148429019,65.4707974591804));
#65910=CARTESIAN_POINT('Ctrl Pts',(2.55976203383379,4.7456251836438,65.6295582214262));
#65911=CARTESIAN_POINT('Ctrl Pts',(-2.59856735630046,4.7244880937792,65.7883189836722));
#65912=CARTESIAN_POINT('Ctrl Pts',(-5.37860852767513,0.379355189119878,
65.947079745918));
#65913=CARTESIAN_POINT('Ctrl Pts',(-3.23598288278473,-4.31297517217702,
66.1058405081639));
#65914=CARTESIAN_POINT('Ctrl Pts',(1.86831314081432,-5.05793891435551,66.2646012704098));
#65915=CARTESIAN_POINT('Ctrl Pts',(5.26267190957225,-1.17372246536004,66.4233620326557));
#65916=CARTESIAN_POINT('Ctrl Pts',(3.84047259628301,3.78472063575253,66.5821227949015));
#65917=CARTESIAN_POINT('Ctrl Pts',(-1.09664454588739,5.27927180522719,66.7408835571475));
#65918=CARTESIAN_POINT('Ctrl Pts',(-5.03007910221774,1.94207216110101,66.8996443193933));
#65919=CARTESIAN_POINT('Ctrl Pts',(-4.35983161843177,-3.17257124623133,
67.0584050816393));
#65920=CARTESIAN_POINT('Ctrl Pts',(0.300666935333765,-5.38358054156236,
67.2171658438851));
#65921=CARTESIAN_POINT('Ctrl Pts',(4.68598592589077,-2.66737248164657,67.375926606131));
#65922=CARTESIAN_POINT('Ctrl Pts',(4.78254746176859,2.49009634942548,67.534687368377));
#65923=CARTESIAN_POINT('Ctrl Pts',(0.50197547582154,5.3685529405199,67.6934481306227));
#65924=CARTESIAN_POINT('Ctrl Pts',(-4.23801979863793,3.33354589586587,67.8522088928688));
#65925=CARTESIAN_POINT('Ctrl Pts',(-5.09924990138375,-1.75242417716988,
68.0109696551145));
#65926=CARTESIAN_POINT('Ctrl Pts',(-1.29349073576672,-5.2345221147663,68.1697304173606));
#65927=CARTESIAN_POINT('Ctrl Pts',(3.69611066141296,-3.92582552236859,68.3284911796063));
#65928=CARTESIAN_POINT('Ctrl Pts',(5.30291868209728,0.975906504002708,68.4872519418522));
#65929=CARTESIAN_POINT('Ctrl Pts',(2.05633354516605,4.98445908845845,68.6460127040982));
#65930=CARTESIAN_POINT('Ctrl Pts',(-3.07227086382722,4.43108246287181,68.804773466344));
#65931=CARTESIAN_POINT('Ctrl Pts',(-5.38903913451035,-0.177756181911403,
68.96353422859));
#65932=CARTESIAN_POINT('Ctrl Pts',(-2.77359417894579,-4.62390693937597,
69.1222949908358));
#65933=CARTESIAN_POINT('Ctrl Pts',(2.38032888972716,-4.83811682684714,69.2810557530817));
#65934=CARTESIAN_POINT('Ctrl Pts',(5.35570225042921,-0.624334412185203,
69.4398165153275));
#65935=CARTESIAN_POINT('Ctrl Pts',(3.42937331948324,4.16085792705156,69.5985772775736));
#65936=CARTESIAN_POINT('Ctrl Pts',(-1.63562282502583,5.13790599639058,69.7573380398193));
#65937=CARTESIAN_POINT('Ctrl Pts',(-5.20364699932156,1.4125855584507,69.9160988020653));
#65938=CARTESIAN_POINT('Ctrl Pts',(-4.00913449237088,-3.60557633057093,
70.0748595643111));
#65939=CARTESIAN_POINT('Ctrl Pts',(0.854660362605124,-5.32380462809097,
70.233620326557));
#65940=CARTESIAN_POINT('Ctrl Pts',(4.93624394778424,-2.1695243122525,70.392381088803));
#65941=CARTESIAN_POINT('Ctrl Pts',(4.50002629241666,2.97037092314251,70.5511418510488));
#65942=CARTESIAN_POINT('Ctrl Pts',(-0.0547528808636342,5.39169195851627,
70.7099026132947));
#65943=CARTESIAN_POINT('Ctrl Pts',(-4.55942054512895,2.87837182208054,70.8686633755406));
#65944=CARTESIAN_POINT('Ctrl Pts',(-4.89116725717831,-2.26932212693528,
71.0274241377865));
#65945=CARTESIAN_POINT('Ctrl Pts',(-0.746368292808977,-5.34006314803305,
71.1861849000323));
#65946=CARTESIAN_POINT('Ctrl Pts',(4.08152973125557,-3.52341526169831,71.3449456622782));
#65947=CARTESIAN_POINT('Ctrl Pts',(5.17388707332602,1.51796989626334,71.5037064245242));
#65948=CARTESIAN_POINT('Ctrl Pts',(1.53094492744998,5.1700626381705,71.66246718677));
#65949=CARTESIAN_POINT('Ctrl Pts',(-3.51316477934987,4.09035613200449,71.8212279490159));
#65950=CARTESIAN_POINT('Ctrl Pts',(-5.34191876907334,-0.732969247726808,
71.9799887112618));
#65951=CARTESIAN_POINT('Ctrl Pts',(-2.28158553030752,-4.88545878310146,
72.1387494735077));
#65952=CARTESIAN_POINT('Ctrl Pts',(2.86692447773331,-4.56662721189998,72.2975102357536));
#65953=CARTESIAN_POINT('Ctrl Pts',(5.39153763240408,-0.0682789269231456,
72.4562709979995));
#65954=CARTESIAN_POINT('Ctrl Pts',(2.98165085923738,4.49256031758063,72.6150317602455));
#65955=CARTESIAN_POINT('Ctrl Pts',(-2.15713385601469,4.94167113239301,72.7737925224911));
#65956=CARTESIAN_POINT('Ctrl Pts',(-5.32164377573057,0.868013581529248,
72.9325532847373));
#65957=CARTESIAN_POINT('Ctrl Pts',(-3.61562276017225,-4.00007651297025,
73.091314046983));
#65958=CARTESIAN_POINT('Ctrl Pts',(1.39952664613108,-5.20717439887132,73.250074809229));
#65959=CARTESIAN_POINT('Ctrl Pts',(5.13378651679711,-1.64850721971224,73.4088355714748));
#65960=CARTESIAN_POINT('Ctrl Pts',(4.16944815373948,3.41892412123604,73.5675963337207));
#65961=CARTESIAN_POINT('Ctrl Pts',(-0.610896517072584,5.35725167403211,
73.7263570959665));
#65962=CARTESIAN_POINT('Ctrl Pts',(-4.83213003538284,2.39245885537094,73.8851178582126));
#65963=CARTESIAN_POINT('Ctrl Pts',(-4.63085054597687,-2.76198538633308,
74.0438786204583));
#65964=CARTESIAN_POINT('Ctrl Pts',(-0.191275185721079,-5.38857623652284,
74.2026393827044));
#65965=CARTESIAN_POINT('Ctrl Pts',(4.42336106708315,-3.08337751884262,74.3614001449501));
#65966=CARTESIAN_POINT('Ctrl Pts',(4.98960215796993,2.04382248707493,74.5201609071961));
#65967=CARTESIAN_POINT('Ctrl Pts',(0.989206944500219,5.30045372345089,74.678921669442));
#65968=CARTESIAN_POINT('Ctrl Pts',(-3.9165406802957,3.70594780765739,74.8376824316877));
#65969=CARTESIAN_POINT('Ctrl Pts',(-5.23775064219211,-1.2803547413539,74.9964431939339));
#65970=CARTESIAN_POINT('Ctrl Pts',(-1.76521122717783,-5.09483752213321,
75.1552039561795));
#65971=CARTESIAN_POINT('Ctrl Pts',(3.32290342202856,-4.24636937881787,75.3139647184255));
#65972=CARTESIAN_POINT('Ctrl Pts',(5.36979535998785,0.488505727033064,75.4727254806714));
#65973=CARTESIAN_POINT('Ctrl Pts',(2.50208656195135,4.77628546990172,75.6314862429173));
#65974=CARTESIAN_POINT('Ctrl Pts',(-2.65560828481232,4.69266285717694,75.7902470051632));
#65975=CARTESIAN_POINT('Ctrl Pts',(-5.38280931270438,0.314171858310403,
75.9490077674091));
#65976=CARTESIAN_POINT('Ctrl Pts',(-3.18349883755812,-4.35185882178607,
76.107768529655));
#65977=CARTESIAN_POINT('Ctrl Pts',(1.92944701495941,-5.03493537892548,76.2665292919008));
#65978=CARTESIAN_POINT('Ctrl Pts',(5.27650402365974,-1.10988528316864,76.4252900541468));
#65979=CARTESIAN_POINT('Ctrl Pts',(3.7943433769926,3.83096572563162,76.5840508163925));
#65980=CARTESIAN_POINT('Ctrl Pts',(-1.16051622802576,5.26559988396195,76.7428115786386));
#65981=CARTESIAN_POINT('Ctrl Pts',(-5.0532359327251,1.88099618864767,76.9015723408843));
#65982=CARTESIAN_POINT('Ctrl Pts',(-4.32107975869319,-3.22515267429361,
77.0603331031303));
#65983=CARTESIAN_POINT('Ctrl Pts',(0.365860599594574,-5.37954329615034,
77.2190938653761));
#65984=CARTESIAN_POINT('Ctrl Pts',(4.7179541617759,-2.61041157308061,77.3778546276221));
#65985=CARTESIAN_POINT('Ctrl Pts',(4.75203196331349,2.54784855773221,77.5366153898679));
#65986=CARTESIAN_POINT('Ctrl Pts',(0.436904959320356,5.37423986346092,77.6953761521139));
#65987=CARTESIAN_POINT('Ctrl Pts',(-4.27809080887851,3.28196268785622,77.8541369143598));
#65988=CARTESIAN_POINT('Ctrl Pts',(-5.07764719280662,-1.81406698853016,
78.0128976766055));
#65989=CARTESIAN_POINT('Ctrl Pts',(-1.22998576712498,-5.24980714561609,
78.1716584388517));
#65990=CARTESIAN_POINT('Ctrl Pts',(3.74339620303386,-3.88076344558682,78.3304192010973));
#65991=CARTESIAN_POINT('Ctrl Pts',(5.29070762465021,1.0400734993063,78.4891799633433));
#65992=CARTESIAN_POINT('Ctrl Pts',(1.99580182141817,5.00900340817564,78.6479407255891));
#65993=CARTESIAN_POINT('Ctrl Pts',(-3.12572277133616,4.39354039588141,78.8067014878351));
#65994=CARTESIAN_POINT('Ctrl Pts',(-5.38649040731852,-0.243024989162281,
78.965462250081));
#65995=CARTESIAN_POINT('Ctrl Pts',(-2.71737749003105,-4.65716648082978,
79.1242230123268));
#65996=CARTESIAN_POINT('Ctrl Pts',(2.43876230950906,-4.8089269542393,79.2829837745728));
#65997=CARTESIAN_POINT('Ctrl Pts',(5.36287235042167,-0.559410588542699,
79.4417445368186));
#65998=CARTESIAN_POINT('Ctrl Pts',(3.37871780515969,4.20209543520715,79.6005052990646));
#65999=CARTESIAN_POINT('Ctrl Pts',(-1.69774247966381,5.11771536197905,79.7592660613104));
#66000=CARTESIAN_POINT('Ctrl Pts',(-5.2203769888794,1.34944586681667,79.9180268235563));
#66001=CARTESIAN_POINT('Ctrl Pts',(-3.96516301938171,-3.65387770501744,
80.0767875858022));
#66002=CARTESIAN_POINT('Ctrl Pts',(0.91908926293675,-5.31306079207099,80.235548348048));
#66003=CARTESIAN_POINT('Ctrl Pts',(4.96216297786599,-2.10956835266785,80.3943091102941));
#66004=CARTESIAN_POINT('Ctrl Pts',(4.46371356421533,3.02466548070436,80.5530698725397));
#66005=CARTESIAN_POINT('Ctrl Pts',(-0.120062849320441,5.39063307652007,
80.7118306347859));
#66006=CARTESIAN_POINT('Ctrl Pts',(-4.59395407577343,2.82292862168424,80.8705913970315));
#66007=CARTESIAN_POINT('Ctrl Pts',(-4.86331820795707,-2.32840633521552,
81.0293521592777));
#66008=CARTESIAN_POINT('Ctrl Pts',(-0.681624964166643,-5.34871269198804,
81.1881129215234));
#66009=CARTESIAN_POINT('Ctrl Pts',(4.12391226721417,-3.47371381457424,81.3468736837694));
#66010=CARTESIAN_POINT('Ctrl Pts',(5.15511902533117,1.58053405205645,81.5056344460152));
#66011=CARTESIAN_POINT('Ctrl Pts',(1.46820338586184,5.18822887591951,81.6643952082611));
#66012=CARTESIAN_POINT('Ctrl Pts',(-3.56245683835765,4.04749815657105,81.823155970507));
#66013=CARTESIAN_POINT('Ctrl Pts',(-5.33264774907332,-0.797626509155247,
81.9819167327528));
#66014=CARTESIAN_POINT('Ctrl Pts',(-2.22223654888384,-4.91273902788576,
82.1406774949988));
#66015=CARTESIAN_POINT('Ctrl Pts',(2.92203341399256,-4.53156273055457,82.2994382572446));
#66016=CARTESIAN_POINT('Ctrl Pts',(5.39196915310808,-0.0029617965042665,
82.4581990194906));
#66017=CARTESIAN_POINT('Ctrl Pts',(2.92701000162586,4.52834985013744,82.6169597817364));
#66018=CARTESIAN_POINT('Ctrl Pts',(-2.21683806821556,4.91517742057454,82.7757205439824));
#66019=CARTESIAN_POINT('Ctrl Pts',(-5.33176830391211,0.803484428152502,
82.9344813062282));
#66020=CARTESIAN_POINT('Ctrl Pts',(-3.56690117349271,-4.04358195702611,
83.0932420684741));
#66021=CARTESIAN_POINT('Ctrl Pts',(1.46250256952503,-5.18983881124397,83.2520028307201));
#66022=CARTESIAN_POINT('Ctrl Pts',(5.15337985091046,-1.58619629785924,83.4107635929658));
#66023=CARTESIAN_POINT('Ctrl Pts',(4.12772540290961,3.46918082523772,83.5695243552118));
#66024=CARTESIAN_POINT('Ctrl Pts',(-0.675747352509778,5.34945901705833,
83.7282851174576));
#66025=CARTESIAN_POINT('Ctrl Pts',(-4.86075944383677,2.33374637252957,83.8870458797035));
#66026=CARTESIAN_POINT('Ctrl Pts',(-4.59704844530487,-2.81787736745293,
84.0458066419496));
#66027=CARTESIAN_POINT('Ctrl Pts',(-0.125992795831606,-5.39050299503273,
84.2045674041953));
#66028=CARTESIAN_POINT('Ctrl Pts',(4.46040309055735,-3.02955776127604,84.3633281664412));
#66029=CARTESIAN_POINT('Ctrl Pts',(4.96444861251837,2.10409705678322,84.5220889286871));
#66030=CARTESIAN_POINT('Ctrl Pts',(0.924981040394022,5.31208351664113,84.6808496909329));
#66031=CARTESIAN_POINT('Ctrl Pts',(-3.96125263942776,3.65816335371309,84.8396104531789));
#66032=CARTESIAN_POINT('Ctrl Pts',(-5.22165301904991,-1.3435792187099,84.9983712154247));
#66033=CARTESIAN_POINT('Ctrl Pts',(-1.70375320028204,-5.11609758128303,
85.1571319776708));
#66034=CARTESIAN_POINT('Ctrl Pts',(3.37484546343723,-4.20532487574203,85.3158927399164));
#66035=CARTESIAN_POINT('Ctrl Pts',(5.36205285859353,0.552597767150946,85.4746535021625));
#66036=CARTESIAN_POINT('Ctrl Pts',(2.4468005092104,4.80802425479881,85.6334142644084));
#66037=CARTESIAN_POINT('Ctrl Pts',(-2.7176845769921,4.65659903150035,85.7921750266542));
#66038=CARTESIAN_POINT('Ctrl Pts',(-4.93173550418608,0.99029557446776,85.9244756618591));
#66039=CARTESIAN_POINT('Ctrl Pts',(-4.26716318148111,-2.08115166207624,
86.0303161700231));
#66040=CARTESIAN_POINT('Ctrl Pts',(-3.26619649360748,-3.2739962098191,86.083236424105));
#66041=CARTESIAN_POINT('Ctrl Pts',(-2.64867169498456,-3.71434815979703,
86.109696551146));
#66042=CARTESIAN_POINT('Ctrl Pts',(-2.08577545033697,4.2697827545171,25.890303448854));
#66043=CARTESIAN_POINT('Ctrl Pts',(-2.79564340622372,3.92301449006545,25.9167635758949));
#66044=CARTESIAN_POINT('Ctrl Pts',(-4.02828411678504,2.86869268329956,25.9696838299769));
#66045=CARTESIAN_POINT('Ctrl Pts',(-5.2368061558258,-0.173451583736938,
26.0755243381408));
#66046=CARTESIAN_POINT('Ctrl Pts',(-3.58937700474797,-4.31948327041665,
26.2078249733457));
#66047=CARTESIAN_POINT('Ctrl Pts',(1.69117135154962,-5.35897536965486,26.3665857355916));
#66048=CARTESIAN_POINT('Ctrl Pts',(5.4148867130437,-1.48550731689914,26.5253464978375));
#66049=CARTESIAN_POINT('Ctrl Pts',(4.18736849490951,3.74332949976516,26.6841072600834));
#66050=CARTESIAN_POINT('Ctrl Pts',(-0.874969621673782,5.54834523009075,
26.8428680223293));
#66051=CARTESIAN_POINT('Ctrl Pts',(-5.13525022907948,2.27420458855161,27.0016287845751));
#66052=CARTESIAN_POINT('Ctrl Pts',(-4.6962499784134,-3.08076179886732,27.1603895468211));
#66053=CARTESIAN_POINT('Ctrl Pts',(0.0412447165789918,-5.61643191744809,
27.319150309067));
#66054=CARTESIAN_POINT('Ctrl Pts',(4.7408118992853,-3.01160959987317,27.4779110713129));
#66055=CARTESIAN_POINT('Ctrl Pts',(5.1015367238218,2.34944503074463,27.6366718335587));
#66056=CARTESIAN_POINT('Ctrl Pts',(0.793130492629709,5.56026007017329,27.7954325958046));
#66057=CARTESIAN_POINT('Ctrl Pts',(-4.24114750411255,3.68213214181093,27.9541933580505));
#66058=CARTESIAN_POINT('Ctrl Pts',(-5.39381106478857,-1.56598352850948,
28.1129541202964));
#66059=CARTESIAN_POINT('Ctrl Pts',(-1.60988703512753,-5.3808695398533,28.2717148825423));
#66060=CARTESIAN_POINT('Ctrl Pts',(3.6474511562916,-4.2710160983281,28.4304756447882));
#66061=CARTESIAN_POINT('Ctrl Pts',(5.5665325305163,0.747800018975952,28.5892364070341));
#66062=CARTESIAN_POINT('Ctrl Pts',(2.39095231205807,5.08220761366869,28.74799716928));
#66063=CARTESIAN_POINT('Ctrl Pts',(-2.97289997872796,4.76522309415968,28.9067579315259));
#66064=CARTESIAN_POINT('Ctrl Pts',(-5.61586367010893,0.0869610876472672,
29.0655186937718));
#66065=CARTESIAN_POINT('Ctrl Pts',(-3.11901725108991,-4.67089049014597,
29.2242794560176));
#66066=CARTESIAN_POINT('Ctrl Pts',(2.23244895427517,-5.15380035052699,29.3830402182635));
#66067=CARTESIAN_POINT('Ctrl Pts',(5.54070972400729,-0.91979474000819,29.5418009805094));
#66068=CARTESIAN_POINT('Ctrl Pts',(3.77794369111745,4.15603513022305,29.7005617427553));
#66069=CARTESIAN_POINT('Ctrl Pts',(-1.44251179621886,5.42813469204637,29.8593225050012));
#66070=CARTESIAN_POINT('Ctrl Pts',(-5.34273643101869,1.73223958412626,30.0180832672471));
#66071=CARTESIAN_POINT('Ctrl Pts',(-4.35312548529055,-3.54905410571791,
30.176844029493));
#66072=CARTESIAN_POINT('Ctrl Pts',(0.620598871036556,-5.58214506939038,
30.3356047917389));
#66073=CARTESIAN_POINT('Ctrl Pts',(5.02633218492865,-2.50628635742007,30.4943655539847));
#66074=CARTESIAN_POINT('Ctrl Pts',(4.83181275145273,2.86340218474256,30.6531263162307));
#66075=CARTESIAN_POINT('Ctrl Pts',(0.215070698416827,5.61241758347815,30.8118870784765));
#66076=CARTESIAN_POINT('Ctrl Pts',(-4.59851062734073,3.22477697638755,30.9706478407224));
#66077=CARTESIAN_POINT('Ctrl Pts',(-5.2033945635623,-2.11427802164059,31.1294086029683));
#66078=CARTESIAN_POINT('Ctrl Pts',(-1.04597285548533,-5.51828119277288,
31.2881693652142));
#66079=CARTESIAN_POINT('Ctrl Pts',(4.06875515960443,-3.87178485819991,31.4469301274601));
#66080=CARTESIAN_POINT('Ctrl Pts',(5.4596341708714,1.31828724381346,31.605690889706));
#66081=CARTESIAN_POINT('Ctrl Pts',(1.853689222264,5.30182259267667,31.7644516519519));
#66082=CARTESIAN_POINT('Ctrl Pts',(-3.4488087242362,4.43296795844451,31.9232124141977));
#66083=CARTESIAN_POINT('Ctrl Pts',(-5.59485158108012,-0.493074358126545,
32.0819731764437));
#66084=CARTESIAN_POINT('Ctrl Pts',(-2.62031537395337,-4.96783996098723,
32.2407339386895));
#66085=CARTESIAN_POINT('Ctrl Pts',(2.75241350199106,-4.89588668690527,32.3994947009355));
#66086=CARTESIAN_POINT('Ctrl Pts',(5.60604946734801,-0.343068370161422,
32.5582554631813));
#66087=CARTESIAN_POINT('Ctrl Pts',(3.3288577211775,4.52373659811392,32.7170162254272));
#66088=CARTESIAN_POINT('Ctrl Pts',(-1.99500629269775,5.25027965246184,32.8757769876731));
#66089=CARTESIAN_POINT('Ctrl Pts',(-5.49297960923532,1.17160639699654,33.034537749919));
#66090=CARTESIAN_POINT('Ctrl Pts',(-3.96361020215392,-3.97935682018335,
33.1932985121649));
#66091=CARTESIAN_POINT('Ctrl Pts',(1.19337633198882,-5.48829112449471,33.3520592744107));
#66092=CARTESIAN_POINT('Ctrl Pts',(5.25814839494067,-1.97417374963327,33.5108200366567));
#66093=CARTESIAN_POINT('Ctrl Pts',(4.51050243460883,3.34676774281486,33.6695807989025));
#66094=CARTESIAN_POINT('Ctrl Pts',(-0.365293128967798,5.60464516868708,
33.8283415611484));
#66095=CARTESIAN_POINT('Ctrl Pts',(-4.9067612628892,2.73298014006108,33.9871023233943));
#66096=CARTESIAN_POINT('Ctrl Pts',(-4.95741161004009,-2.63999179271414,
34.1458630856402));
#66097=CARTESIAN_POINT('Ctrl Pts',(-0.470887425572999,-5.59676259719809,
34.3046238478861));
#66098=CARTESIAN_POINT('Ctrl Pts',(4.4466073142222,-3.43120531738688,34.463384610132));
#66099=CARTESIAN_POINT('Ctrl Pts',(5.29443121665232,1.87469587642792,34.6221453723779));
#66100=CARTESIAN_POINT('Ctrl Pts',(1.296629949095,5.4648181408047,34.7809061346238));
#66101=CARTESIAN_POINT('Ctrl Pts',(-3.88788665395154,4.05337191767345,34.9396668968696));
#66102=CARTESIAN_POINT('Ctrl Pts',(-5.51409063425751,-1.06784409636987,
35.0984276591156));
#66103=CARTESIAN_POINT('Ctrl Pts',(-2.09363043599948,-5.21173657569289,
35.2571884213614));
#66104=CARTESIAN_POINT('Ctrl Pts',(3.2429842880596,-4.58568854637521,35.4159491836074));
#66105=CARTESIAN_POINT('Ctrl Pts',(5.61152073344166,0.237321712265504,35.5747099458532));
#66106=CARTESIAN_POINT('Ctrl Pts',(2.8442219974453,4.84312789075476,35.7334707080991));
#66107=CARTESIAN_POINT('Ctrl Pts',(-2.52619558850515,5.01635548835761,35.892231470345));
#66108=CARTESIAN_POINT('Ctrl Pts',(-5.58456180820669,0.598461316442061,
36.0509922325909));
#66109=CARTESIAN_POINT('Ctrl Pts',(-3.53176647837594,-4.36716293252018,
36.2097529948368));
#66110=CARTESIAN_POINT('Ctrl Pts',(1.7534094116762,-5.33582626891128,36.3685137570827));
#66111=CARTESIAN_POINT('Ctrl Pts',(5.43381144957445,-1.4209784190592,36.5272745193285));
#66112=CARTESIAN_POINT('Ctrl Pts',(4.14102327089027,3.79439228426682,36.6860352815745));
#66113=CARTESIAN_POINT('Ctrl Pts',(-0.941755894515449,5.5370192678104,36.8447960438203));
#66114=CARTESIAN_POINT('Ctrl Pts',(-5.16261129895229,2.2119970869982,37.0035568060662));
#66115=CARTESIAN_POINT('Ctrl Pts',(-4.65848714857258,-3.13751239416556,
37.1623175683121));
#66116=CARTESIAN_POINT('Ctrl Pts',(0.109226735523501,-5.61547469562505,
37.321078330558));
#66117=CARTESIAN_POINT('Ctrl Pts',(4.77697297489437,-2.95398302874052,37.4798390928039));
#66118=CARTESIAN_POINT('Ctrl Pts',(5.07268763310252,2.4110841366338,37.6385998550498));
#66119=CARTESIAN_POINT('Ctrl Pts',(0.725723622233936,5.56945345263699,37.7973606172957));
#66120=CARTESIAN_POINT('Ctrl Pts',(-4.2854448152198,3.63048884761598,37.9561213795416));
#66121=CARTESIAN_POINT('Ctrl Pts',(-5.37444325716809,-1.63121004546892,
38.1148821417874));
#66122=CARTESIAN_POINT('Ctrl Pts',(-1.54458706564933,-5.39997567898108,
38.2736429040334));
#66123=CARTESIAN_POINT('Ctrl Pts',(3.69892238837796,-4.22651862668493,38.4324036662792));
#66124=CARTESIAN_POINT('Ctrl Pts',(5.55706508750621,0.815177373445694,38.5911644285252));
#66125=CARTESIAN_POINT('Ctrl Pts',(2.32921207578554,5.11079814148172,38.749925190771));
#66126=CARTESIAN_POINT('Ctrl Pts',(-3.0304069744033,4.7288603390718,38.908685953017));
#66127=CARTESIAN_POINT('Ctrl Pts',(-5.61650499663195,0.0189251094235045,
39.0674467152627));
#66128=CARTESIAN_POINT('Ctrl Pts',(-3.0622060875641,-4.70833095844415,39.2262074775087));
#66129=CARTESIAN_POINT('Ctrl Pts',(2.29471736914525,-5.126378715302,39.3849682397545));
#66130=CARTESIAN_POINT('Ctrl Pts',(5.55144539655818,-0.852608084638733,
39.5437290020005));
#66131=CARTESIAN_POINT('Ctrl Pts',(3.72732102593349,4.20149550833897,39.7024897642464));
#66132=CARTESIAN_POINT('Ctrl Pts',(-1.50816140012871,5.41026207573349,39.8612505264922));
#66133=CARTESIAN_POINT('Ctrl Pts',(-5.3633284454033,1.66739153280986,40.0200112887382));
#66134=CARTESIAN_POINT('Ctrl Pts',(-4.30981347244434,-3.60152667207889,
40.178772050984));
#66135=CARTESIAN_POINT('Ctrl Pts',(0.688174435462339,-5.57421765661644,
40.3375328132299));
#66136=CARTESIAN_POINT('Ctrl Pts',(5.05632407947203,-2.4452143751233,40.4962935754758));
#66137=CARTESIAN_POINT('Ctrl Pts',(4.79677147851891,2.92172379252827,40.6550543377217));
#66138=CARTESIAN_POINT('Ctrl Pts',(0.147067101132706,5.61461110004271,40.8138150999676));
#66139=CARTESIAN_POINT('Ctrl Pts',(-4.63723757943327,3.16883482826894,40.9725758622135));
#66140=CARTESIAN_POINT('Ctrl Pts',(-5.1774007810357,-2.17715587165673,41.1313366244594));
#66141=CARTESIAN_POINT('Ctrl Pts',(-0.979048642068222,-5.53054701575012,
41.2900973867053));
#66142=CARTESIAN_POINT('Ctrl Pts',(4.11535871955024,-3.82221259827082,41.4488581489512));
#66143=CARTESIAN_POINT('Ctrl Pts',(5.44326407576748,1.38432754014994,41.607618911197));
#66144=CARTESIAN_POINT('Ctrl Pts',(1.7893278831762,5.32388882899019,41.7663796734429));
#66145=CARTESIAN_POINT('Ctrl Pts',(-3.50225584382976,4.39086444123689,41.9251404356888));
#66146=CARTESIAN_POINT('Ctrl Pts',(-5.58846804476507,-0.560813203837097,
42.0839011979347));
#66147=CARTESIAN_POINT('Ctrl Pts',(-2.55994358915231,-4.99921747449702,
42.2426619601806));
#66148=CARTESIAN_POINT('Ctrl Pts',(2.81151943374774,-4.86218520941121,42.4014227224265));
#66149=CARTESIAN_POINT('Ctrl Pts',(5.60979399190252,-0.275132523291236,
42.5601834846724));
#66150=CARTESIAN_POINT('Ctrl Pts',(3.27381373527952,4.56372985217721,42.7189442469183));
#66151=CARTESIAN_POINT('Ctrl Pts',(-2.05846085181392,5.22572726598967,42.8777050091642));
#66152=CARTESIAN_POINT('Ctrl Pts',(-5.50676919082185,1.10497946405063,43.03646577141));
#66153=CARTESIAN_POINT('Ctrl Pts',(-3.91511415993451,-4.02707929542473,
43.1952265336559));
#66154=CARTESIAN_POINT('Ctrl Pts',(1.25977293884402,-5.47343207498865,43.3539872959018));
#66155=CARTESIAN_POINT('Ctrl Pts',(5.28167736372706,-1.91033263136333,43.5127480581477));
#66156=CARTESIAN_POINT('Ctrl Pts',(4.46962933439137,3.40116158835573,43.6715088203935));
#66157=CARTESIAN_POINT('Ctrl Pts',(-0.433159988384986,5.59980883257818,
43.8302695826396));
#66158=CARTESIAN_POINT('Ctrl Pts',(-4.93950805874728,2.67333998483713,43.9890303448854));
#66159=CARTESIAN_POINT('Ctrl Pts',(-4.92506747450587,-2.69985127525994,
44.1477911071313));
#66160=CARTESIAN_POINT('Ctrl Pts',(-0.403054699451855,-5.60205618020814,
44.3065518693771));
#66161=CARTESIAN_POINT('Ctrl Pts',(4.48784604800658,-3.37708815199574,44.4653126316231));
#66162=CARTESIAN_POINT('Ctrl Pts',(5.27133300928694,1.93869410742388,44.6240733938689));
#66163=CARTESIAN_POINT('Ctrl Pts',(1.2303349855046,5.48012430154663,44.7828341561148));
#66164=CARTESIAN_POINT('Ctrl Pts',(-3.93670319808305,4.00597734231749,44.9415949183607));
#66165=CARTESIAN_POINT('Ctrl Pts',(-5.50075036662014,-1.13456244477178,
45.1003556806066));
#66166=CARTESIAN_POINT('Ctrl Pts',(-2.03034277701881,-5.23671602674481,
45.2591164428525));
#66167=CARTESIAN_POINT('Ctrl Pts',(3.2982965397378,-4.5460671434672,45.4178772050984));
#66168=CARTESIAN_POINT('Ctrl Pts',(5.60823411554676,0.305281250940591,45.5766379673442));
#66169=CARTESIAN_POINT('Ctrl Pts',(2.78534452306571,4.87722691955032,45.7353987295903));
#66170=CARTESIAN_POINT('Ctrl Pts',(-2.5867774563813,4.98538553455152,45.894159491836));
#66171=CARTESIAN_POINT('Ctrl Pts',(-5.59140169360195,0.53076702774728,46.052920254082));
#66172=CARTESIAN_POINT('Ctrl Pts',(-3.47860430924953,-4.40962567534128,
46.2116810163279));
#66173=CARTESIAN_POINT('Ctrl Pts',(1.81791799428017,-5.3141942665874,46.3704417785737));
#66174=CARTESIAN_POINT('Ctrl Pts',(5.45062622041652,-1.35504994087535,46.5292025408197));
#66175=CARTESIAN_POINT('Ctrl Pts',(4.09475483808194,3.84427748126524,46.6879633030655));
#66176=CARTESIAN_POINT('Ctrl Pts',(-1.00876124798033,5.52520472756723,46.8467240653114));
#66177=CARTESIAN_POINT('Ctrl Pts',(-5.18902822687748,2.14929583762384,47.0054848275573));
#66178=CARTESIAN_POINT('Ctrl Pts',(-4.62013807160538,-3.19371425400909,
47.1642455898032));
#66179=CARTESIAN_POINT('Ctrl Pts',(0.177243570754919,-5.61373950710082,
47.3230063520491));
#66180=CARTESIAN_POINT('Ctrl Pts',(4.81240648318495,-2.89589888938787,47.4817671142949));
#66181=CARTESIAN_POINT('Ctrl Pts',(5.04310798533405,2.47235684827615,47.6405278765409));
#66182=CARTESIAN_POINT('Ctrl Pts',(0.658203015566318,5.57783607927463,47.7992886387866));
#66183=CARTESIAN_POINT('Ctrl Pts',(-4.32910945912064,3.57830935329949,47.9580494010327));
#66184=CARTESIAN_POINT('Ctrl Pts',(-5.35428872245015,-1.69619539369769,
48.1168101632785));
#66185=CARTESIAN_POINT('Ctrl Pts',(-1.47905939811478,-5.41829030541985,
48.2755709255244));
#66186=CARTESIAN_POINT('Ctrl Pts',(3.74985026583283,-4.18140042578941,48.4343316877703));
#66187=CARTESIAN_POINT('Ctrl Pts',(5.54678242582246,0.882434846062579,48.5930924500162));
#66188=CARTESIAN_POINT('Ctrl Pts',(2.26712988102407,5.13863879247473,48.7518532122621));
#66189=CARTESIAN_POINT('Ctrl Pts',(-3.08746918127143,4.69180355424833,48.9106139745079));
#66190=CARTESIAN_POINT('Ctrl Pts',(-5.61632214089325,-0.0491136098317049,
49.0693747367539));
#66191=CARTESIAN_POINT('Ctrl Pts',(-3.00494552437603,-4.74508049799904,
49.2281354989997));
#66192=CARTESIAN_POINT('Ctrl Pts',(2.35664902330628,-5.09820477402661,49.3868962612456));
#66193=CARTESIAN_POINT('Ctrl Pts',(5.561366400077,-0.785296314172567,49.5456570234916));
#66194=CARTESIAN_POINT('Ctrl Pts',(3.67615137334867,4.24633931960047,49.7044177857373));
#66195=CARTESIAN_POINT('Ctrl Pts',(-1.57358967977417,5.39159550195178,49.8631785479833));
#66196=CARTESIAN_POINT('Ctrl Pts',(-5.38313339204505,1.60229879248781,50.0219393102291));
#66197=CARTESIAN_POINT('Ctrl Pts',(-4.26586899396583,-3.65347071471485,
50.1807000724751));
#66198=CARTESIAN_POINT('Ctrl Pts',(0.755649010055931,-5.56547222709447,
50.339460834721));
#66199=CARTESIAN_POINT('Ctrl Pts',(5.08557395847498,-2.38378355767454,50.4982215969668));
#66200=CARTESIAN_POINT('Ctrl Pts',(4.76102627921851,2.97961663734597,50.6569823592128));
#66201=CARTESIAN_POINT('Ctrl Pts',(0.0790419217800287,5.61598067229221,
50.8157431214586));
#66202=CARTESIAN_POINT('Ctrl Pts',(-4.6752840168385,3.11242765359339,50.9745038837046));
#66203=CARTESIAN_POINT('Ctrl Pts',(-5.15064721483666,-2.2397142240147,51.1332646459504));
#66204=CARTESIAN_POINT('Ctrl Pts',(-0.911980753248584,-5.54200123084275,
51.2920254081963));
#66205=CARTESIAN_POINT('Ctrl Pts',(4.16135835052739,-3.77207942857173,51.4507861704422));
#66206=CARTESIAN_POINT('Ctrl Pts',(5.42609518155485,1.45016468639448,51.6095469326881));
#66207=CARTESIAN_POINT('Ctrl Pts',(1.72470396018791,5.34517378451539,51.768307694934));
#66208=CARTESIAN_POINT('Ctrl Pts',(-3.55518900731147,4.34811656458864,51.9270684571799));
#66209=CARTESIAN_POINT('Ctrl Pts',(-5.58126440065713,-0.62846975019945,
52.0858292194257));
#66210=CARTESIAN_POINT('Ctrl Pts',(-2.49919613258049,-5.0298613527465,52.2445899816716));
#66211=CARTESIAN_POINT('Ctrl Pts',(2.87021277497366,-4.82777020614449,52.4033507439175));
#66212=CARTESIAN_POINT('Ctrl Pts',(5.61271527908117,-0.207156300717966,
52.5621115061634));
#66213=CARTESIAN_POINT('Ctrl Pts',(3.2182893171531,4.60305337879721,52.7208722684093));
#66214=CARTESIAN_POINT('Ctrl Pts',(-2.12161333176065,5.20040800394102,52.8796330306552));
#66215=CARTESIAN_POINT('Ctrl Pts',(-5.51975065392403,1.03819037534721,53.038393792901));
#66216=CARTESIAN_POINT('Ctrl Pts',(-3.86604357463707,-4.07421079670234,
53.197154555147));
#66217=CARTESIAN_POINT('Ctrl Pts',(1.32598467399636,-5.45776979922066,53.3559153173929));
#66218=CARTESIAN_POINT('Ctrl Pts',(5.30443124625904,-1.84621117174306,53.5146760796387));
#66219=CARTESIAN_POINT('Ctrl Pts',(4.4281003159834,3.4550563133683,53.6734368418847));
#66220=CARTESIAN_POINT('Ctrl Pts',(-0.500963281565584,5.59415072441577,
53.8321976041305));
#66221=CARTESIAN_POINT('Ctrl Pts',(-4.97152998170303,2.61330751691913,53.9909583663765));
#66222=CARTESIAN_POINT('Ctrl Pts',(-4.89200058522532,-2.75931455457936,
54.1497191286223));
#66223=CARTESIAN_POINT('Ctrl Pts',(-0.33516282504586,-5.60652766136632,
54.3084798908682));
#66224=CARTESIAN_POINT('Ctrl Pts',(4.5284261902974,-3.32247539885354,54.4672406531142));
#66225=CARTESIAN_POINT('Ctrl Pts',(5.24746123370139,2.00240783502248,54.6260014153599));
#66226=CARTESIAN_POINT('Ctrl Pts',(1.16385947023147,5.49462625394218,54.7847621776059));
#66227=CARTESIAN_POINT('Ctrl Pts',(-3.9849420309447,3.95799488970978,54.9435229398517));
#66228=CARTESIAN_POINT('Ctrl Pts',(-5.48660286376106,-1.20111429611312,
55.1022837020977));
#66229=CARTESIAN_POINT('Ctrl Pts',(-1.96675716519669,-5.26092698961938,
55.2610444643435));
#66230=CARTESIAN_POINT('Ctrl Pts',(3.35312476633552,-4.50577860511874,55.4198052265895));
#66231=CARTESIAN_POINT('Ctrl Pts',(5.60412448918787,0.373195989586127,55.5785659888352));
#66232=CARTESIAN_POINT('Ctrl Pts',(2.72605829932405,4.91061021520187,55.7373267510813));
#66233=CARTESIAN_POINT('Ctrl Pts',(-2.64697971461612,4.95368397532273,55.8960875133271));
#66234=CARTESIAN_POINT('Ctrl Pts',(-5.59742104069143,0.462994848981032,
56.054848275573));
#66235=CARTESIAN_POINT('Ctrl Pts',(-3.4249316548741,-4.45144130550992,56.2136090378189));
#66236=CARTESIAN_POINT('Ctrl Pts',(1.88215979738361,-5.29178240615308,56.3723698000648));
#66237=CARTESIAN_POINT('Ctrl Pts',(5.46664111175626,-1.28892260908666,56.5311305623107));
#66238=CARTESIAN_POINT('Ctrl Pts',(4.04788549992257,3.8935985304696,56.6898913245566));
#66239=CARTESIAN_POINT('Ctrl Pts',(-1.07561856571275,5.51257936342436,56.8486520868024));
#66240=CARTESIAN_POINT('Ctrl Pts',(-5.21468366481089,2.08627917904408,57.0074128490483));
#66241=CARTESIAN_POINT('Ctrl Pts',(-4.58111098928757,-3.24944743622466,
57.1661736112942));
#66242=CARTESIAN_POINT('Ctrl Pts',(0.245234395488895,-5.61118050219625,
57.3249343735402));
#66243=CARTESIAN_POINT('Ctrl Pts',(4.84713377073179,-2.83738977681774,57.4836951357859));
#66244=CARTESIAN_POINT('Ctrl Pts',(5.01278826137211,2.53326674150361,57.6424558980319));
#66245=CARTESIAN_POINT('Ctrl Pts',(0.590585817593506,5.58540015836071,57.8012166602777));
#66246=CARTESIAN_POINT('Ctrl Pts',(-4.37213880612535,3.52560474201678,57.9599774225237));
#66247=CARTESIAN_POINT('Ctrl Pts',(-5.33334844575954,-1.76093182521995,
58.1187381847696));
#66248=CARTESIAN_POINT('Ctrl Pts',(-1.41331467858517,-5.43580979765242,
58.2774989470154));
#66249=CARTESIAN_POINT('Ctrl Pts',(3.80022785268933,-4.1356686043012,58.4362597092614));
#66250=CARTESIAN_POINT('Ctrl Pts',(5.53568577371134,0.949562821348838,58.5950204715072));
#66251=CARTESIAN_POINT('Ctrl Pts',(2.20471498490915,5.16572534812638,58.7537812337531));
#66252=CARTESIAN_POINT('Ctrl Pts',(-3.144078301978,4.65405824716339,58.9125419959989));
#66253=CARTESIAN_POINT('Ctrl Pts',(-5.61531508977269,-0.117145121663757,
59.071302758245));
#66254=CARTESIAN_POINT('Ctrl Pts',(-2.94724398537462,-4.78113369689988,
59.2300635204908));
#66255=CARTESIAN_POINT('Ctrl Pts',(2.41823483917798,-5.06928267110287,59.3888242827367));
#66256=CARTESIAN_POINT('Ctrl Pts',(5.57047127296998,-0.717869301457213,
59.5475850449825));
#66257=CARTESIAN_POINT('Ctrl Pts',(3.6244422454793,4.29055998048545,59.7063458072285));
#66258=CARTESIAN_POINT('Ctrl Pts',(-1.63878703510391,5.37213771142675,59.8651065694744));
#66259=CARTESIAN_POINT('Ctrl Pts',(-5.40214836375828,1.53697091478732,60.0238673317203));
#66260=CARTESIAN_POINT('Ctrl Pts',(-4.22129849913074,-3.70487861045338,
60.1826280939661));
#66261=CARTESIAN_POINT('Ctrl Pts',(0.823012693142843,-5.55591006441646,
60.3413888562121));
#66262=CARTESIAN_POINT('Ctrl Pts',(5.11407752940203,-2.32200291994295,60.5001496184578));
#66263=CARTESIAN_POINT('Ctrl Pts',(4.72458239922035,3.03707222336503,60.6589103807039));
#66264=CARTESIAN_POINT('Ctrl Pts',(0.0110051430237869,5.61652609927038,
60.8176711429496));
#66265=CARTESIAN_POINT('Ctrl Pts',(-4.71264435622464,3.05556373009997,60.9764319051957));
#66266=CARTESIAN_POINT('Ctrl Pts',(-5.12313779106008,-2.30194389826733,
61.1351926674413));
#66267=CARTESIAN_POINT('Ctrl Pts',(-0.844779031235954,-5.55264215714847,
61.2939534296875));
#66268=CARTESIAN_POINT('Ctrl Pts',(4.20674730208683,-3.72139270614424,61.4527141919332));
#66269=CARTESIAN_POINT('Ctrl Pts',(5.4081300077703,1.51578902094353,61.6114749541792));
#66270=CARTESIAN_POINT('Ctrl Pts',(1.65982693686032,5.36567433568524,61.770235716425));
#66271=CARTESIAN_POINT('Ctrl Pts',(-3.60760044673811,4.30473060175118,61.9289964786709));
#66272=CARTESIAN_POINT('Ctrl Pts',(-5.5732417058914,-0.696034068613847,
62.0877572409168));
#66273=CARTESIAN_POINT('Ctrl Pts',(-2.43808191892836,-5.05976709874605,
62.2465180031627));
#66274=CARTESIAN_POINT('Ctrl Pts',(2.92848491241984,-4.79264672750744,62.4052787654085));
#66275=CARTESIAN_POINT('Ctrl Pts',(5.61481290018499,-0.139149677953565,
62.5640395276545));
#66276=CARTESIAN_POINT('Ctrl Pts',(3.16229261500766,4.64170140724564,62.7228002899003));
#66277=CARTESIAN_POINT('Ctrl Pts',(-2.18445446491029,5.17432558191808,62.8815610521463));
#66278=CARTESIAN_POINT('Ctrl Pts',(-5.53192209351194,0.97124893218624,63.0403218143921));
#66279=CARTESIAN_POINT('Ctrl Pts',(-3.81640564737093,-4.12074440746734,
63.199082576638));
#66280=CARTESIAN_POINT('Ctrl Pts',(1.39200182087229,-5.44130659563001,63.357843338884));
#66281=CARTESIAN_POINT('Ctrl Pts',(5.32640670340396,-1.78181878059799,63.5166041011298));
#66282=CARTESIAN_POINT('Ctrl Pts',(4.38592147376913,3.50844400880067,63.6753648633758));
#66283=CARTESIAN_POINT('Ctrl Pts',(-0.568693058375023,5.58767167452727,
63.8341256256215));
#66284=CARTESIAN_POINT('Ctrl Pts',(-5.00282233253868,2.55289154607289,63.9928863878675));
#66285=CARTESIAN_POINT('Ctrl Pts',(-4.85821579476509,-2.818372904435,64.1516471501133));
#66286=CARTESIAN_POINT('Ctrl Pts',(-0.267221765488804,-5.61017638448271,
64.3104079123593));
#66287=CARTESIAN_POINT('Ctrl Pts',(4.56834178595791,-3.26737507238287,64.4691686746051));
#66288=CARTESIAN_POINT('Ctrl Pts',(5.2228193930792,2.06582770923283,64.6279294368511));
#66289=CARTESIAN_POINT('Ctrl Pts',(1.0972131585588,5.50832186982966,64.7866901990968));
#66290=CARTESIAN_POINT('Ctrl Pts',(-4.03259607348695,3.90943160127608,64.9454509613429));
#66291=CARTESIAN_POINT('Ctrl Pts',(-5.4716502018265,-1.26748988390853,65.1042117235886));
#66292=CARTESIAN_POINT('Ctrl Pts',(-1.90288293172278,-5.28436591135743,
65.2629724858347));
#66293=CARTESIAN_POINT('Ctrl Pts',(3.40746092180959,-4.46482884367352,65.4217332480805));
#66294=CARTESIAN_POINT('Ctrl Pts',(5.59919245745271,0.441055961713188,65.5804940103263));
#66295=CARTESIAN_POINT('Ctrl Pts',(2.66637202647467,4.94327287871016,65.7392547725723));
#66296=CARTESIAN_POINT('Ctrl Pts',(-2.70679352852708,4.92125546287557,65.8980155348181));
#66297=CARTESIAN_POINT('Ctrl Pts',(-5.60261896613596,0.395154725711709,
66.0567762970641));
#66298=CARTESIAN_POINT('Ctrl Pts',(-3.37075639171248,-4.49260368658171,
66.2155370593099));
#66299=CARTESIAN_POINT('Ctrl Pts',(1.94612539350076,-5.26859397654912,66.3742978215559));
#66300=CARTESIAN_POINT('Ctrl Pts',(5.48185377340806,-1.22260612788034,66.5330585838017));
#66301=CARTESIAN_POINT('Ctrl Pts',(4.00042213448843,3.94234819401505,66.6918193460476));
#66302=CARTESIAN_POINT('Ctrl Pts',(-1.1423180364002,5.49914502815419,66.8505801082935));
#66303=CARTESIAN_POINT('Ctrl Pts',(-5.23957384781653,2.02295635895467,67.0093408705393));
#66304=CARTESIAN_POINT('Ctrl Pts',(-4.54141162884421,-3.30470376196668,
67.1681016327853));
#66305=CARTESIAN_POINT('Ctrl Pts',(0.31318923207078,-5.60779805644547,67.3268623950311));
#66306=CARTESIAN_POINT('Ctrl Pts',(4.88114974130499,-2.77846427724327,67.4856231572771));
#66307=CARTESIAN_POINT('Ctrl Pts',(4.98173291063654,2.59380487778839,67.6443839195229));
#66308=CARTESIAN_POINT('Ctrl Pts',(0.522881951140529,5.59214457986643,67.8031446817689));
#66309=CARTESIAN_POINT('Ctrl Pts',(-4.41452654167645,3.47238274817052,67.9619054440147));
#66310=CARTESIAN_POINT('Ctrl Pts',(-5.31162550008227,-1.82540983996319,
68.1206662062607));
#66311=CARTESIAN_POINT('Ctrl Pts',(-1.34736255509922,-5.45253158469304,
68.2794269685065));
#66312=CARTESIAN_POINT('Ctrl Pts',(3.85004775603573,-4.08932987336585,68.4381877307524));
#66313=CARTESIAN_POINT('Ctrl Pts',(5.52377675960678,1.01655144827307,68.5969484929983));
#66314=CARTESIAN_POINT('Ctrl Pts',(2.14197654682777,5.19205383348419,68.7557092552442));
#66315=CARTESIAN_POINT('Ctrl Pts',(-3.20022602913364,4.61562995694134,68.9144700174901));
#66316=CARTESIAN_POINT('Ctrl Pts',(-5.61348399105505,-0.185159442447144,
69.073230779736));
#66317=CARTESIAN_POINT('Ctrl Pts',(-2.88910993826166,-4.81648526433911,
69.2319915419818));
#66318=CARTESIAN_POINT('Ctrl Pts',(2.47946577904082,-5.0396166508499,69.3907523042278));
#66319=CARTESIAN_POINT('Ctrl Pts',(5.57875867909682,-0.650336941407984,
69.5495130664736));
#66320=CARTESIAN_POINT('Ctrl Pts',(3.57220123064088,4.33415100161104,69.7082738287195));
#66321=CARTESIAN_POINT('Ctrl Pts',(-1.70374389840499,5.35189155958961,69.8670345909654));
#66322=CARTESIAN_POINT('Ctrl Pts',(-5.42037057009564,1.47141748657539,70.0257953532113));
#66323=CARTESIAN_POINT('Ctrl Pts',(-4.17610852865976,-3.75574281518495,
70.1845561154572));
#66324=CARTESIAN_POINT('Ctrl Pts',(0.89025559910136,-5.54553257182993,70.343316877703));
#66325=CARTESIAN_POINT('Ctrl Pts',(5.14183060935358,-2.2598815282383,70.5020776399489));
#66326=CARTESIAN_POINT('Ctrl Pts',(4.68744518666451,3.09408211897719,70.6608384021949));
#66327=CARTESIAN_POINT('Ctrl Pts',(-0.0570332507375796,5.61624730093583,
70.8195991644407));
#66328=CARTESIAN_POINT('Ctrl Pts',(-4.74931311496125,2.99825140257037,70.9783599266866));
#66329=CARTESIAN_POINT('Ctrl Pts',(-5.09487654671437,-2.36383576220895,
71.1371206889325));
#66330=CARTESIAN_POINT('Ctrl Pts',(-0.777453337884133,-5.56246823311117,
71.2958814511784));
#66331=CARTESIAN_POINT('Ctrl Pts',(4.25151891339917,-3.67015986926562,71.4546422134243));
#66332=CARTESIAN_POINT('Ctrl Pts',(5.38937119080337,1.58119091342487,71.6134029756702));
#66333=CARTESIAN_POINT('Ctrl Pts',(1.59470633389773,5.38538747404349,71.7721637379161));
#66334=CARTESIAN_POINT('Ctrl Pts',(-3.65948247073021,4.26071291961525,71.9309245001618));
#66335=CARTESIAN_POINT('Ctrl Pts',(-5.56440113779842,-0.763496244015491,
72.089685262408));
#66336=CARTESIAN_POINT('Ctrl Pts',(-2.3766099167077,-5.08893032382693,72.2484460246537));
#66337=CARTESIAN_POINT('Ctrl Pts',(2.98632729464914,-4.75681992787116,72.4072067868998));
#66338=CARTESIAN_POINT('Ctrl Pts',(5.61608654738804,-0.0711226349710497,
72.5659675491454));
#66339=CARTESIAN_POINT('Ctrl Pts',(3.10583184636022,4.67966826592364,72.7247283113916));
#66340=CARTESIAN_POINT('Ctrl Pts',(-2.24697502932542,5.14748382751671,72.8834890736371));
#66341=CARTESIAN_POINT('Ctrl Pts',(-5.54328172342653,0.904164958225804,
73.0422498358833));
#66342=CARTESIAN_POINT('Ctrl Pts',(-3.76620766250282,-4.1666732989117,73.2010105981289));
#66343=CARTESIAN_POINT('Ctrl Pts',(1.45781469145456,-5.42404488019209,73.3597713603751));
#66344=CARTESIAN_POINT('Ctrl Pts',(5.34760051026307,-1.71716490751244,73.5185321226207));
#66345=CARTESIAN_POINT('Ctrl Pts',(4.3430989974944,3.56131684000752,73.6772928848668));
#66346=CARTESIAN_POINT('Ctrl Pts',(-0.636339379467287,5.58037263371339,
73.8360536471125));
#66347=CARTESIAN_POINT('Ctrl Pts',(-5.03338051910119,2.49210093834326,73.9948144093586));
#66348=CARTESIAN_POINT('Ctrl Pts',(-4.82371806104376,-2.87701765801306,
74.1535751716043));
#66349=CARTESIAN_POINT('Ctrl Pts',(-0.199241491132339,-5.61300181410709,
74.3123359338505));
#66350=CARTESIAN_POINT('Ctrl Pts',(4.60758697737389,-3.21179525855753,74.4710966960961));
#66351=CARTESIAN_POINT('Ctrl Pts',(5.19741110361085,2.12894442318739,74.6298574583422));
#66352=CARTESIAN_POINT('Ctrl Pts',(1.0304058308339,5.52120913937719,74.7886182205879));
#66353=CARTESIAN_POINT('Ctrl Pts',(-4.07965833247825,3.86029460367982,74.9473789828338));
#66354=CARTESIAN_POINT('Ctrl Pts',(-5.45589457511983,-1.33367946753936,
75.1061397450798));
#66355=CARTESIAN_POINT('Ctrl Pts',(-1.8387294501421,-5.30702935229665,75.2649005073255));
#66356=CARTESIAN_POINT('Ctrl Pts',(3.46129703232802,-4.42322386850986,75.4236612695716));
#66357=CARTESIAN_POINT('Ctrl Pts',(5.5934387441171,0.508851208869345,75.5824220318174));
#66358=CARTESIAN_POINT('Ctrl Pts',(2.60629446347919,4.97521011682889,75.7411827940634));
#66359=CARTESIAN_POINT('Ctrl Pts',(-2.76621012043596,4.88810475609477,75.8999435563092));
#66360=CARTESIAN_POINT('Ctrl Pts',(-5.60699470713969,0.327256613478776,
76.0587043185551));
#66361=CARTESIAN_POINT('Ctrl Pts',(-3.31608646998587,-4.53310677797631,
76.2174650808009));
#66362=CARTESIAN_POINT('Ctrl Pts',(2.00980539567907,-5.24463238067812,76.3762258430469));
#66363=CARTESIAN_POINT('Ctrl Pts',(5.49626197291347,-1.15611022920134,76.5349866052928));
#66364=CARTESIAN_POINT('Ctrl Pts',(3.95237170702942,3.99051931788734,76.6937473675386));
#66365=CARTESIAN_POINT('Ctrl Pts',(-1.20884987189374,5.48490369324573,76.8525081297847));
#66366=CARTESIAN_POINT('Ctrl Pts',(-5.26369512325953,1.95933666998091,77.0112688920303));
#66367=CARTESIAN_POINT('Ctrl Pts',(-4.50104581615728,-3.35947512236825,
77.1700296542764));
#66368=CARTESIAN_POINT('Ctrl Pts',(0.381098108126755,-5.60359266622235,
77.3287904165222));
#66369=CARTESIAN_POINT('Ctrl Pts',(4.91444940305996,-2.71913103798297,77.4875511787681));
#66370=CARTESIAN_POINT('Ctrl Pts',(4.94994649050095,2.65396237315744,77.646311941014));
#66371=CARTESIAN_POINT('Ctrl Pts',(0.455101351751309,5.59806835404786,77.8050727032599));
#66372=CARTESIAN_POINT('Ctrl Pts',(-4.45626644537291,3.41865118208945,77.9638334655057));
#66373=CARTESIAN_POINT('Ctrl Pts',(-5.28912307326102,-1.88961997577731,
78.1225942277517));
#66374=CARTESIAN_POINT('Ctrl Pts',(-1.28121270613263,-5.468453212619,78.2813549899975));
#66375=CARTESIAN_POINT('Ctrl Pts',(3.89930266479998,-4.04239103319333,78.4401157522435));
#66376=CARTESIAN_POINT('Ctrl Pts',(5.51105713115687,1.08339089625261,78.5988765144893));
#66377=CARTESIAN_POINT('Ctrl Pts',(2.07892377364716,5.21762038484239,78.7576372767352));
#66378=CARTESIAN_POINT('Ctrl Pts',(-3.2559041230579,4.57652432293467,78.9163980389812));
#66379=CARTESIAN_POINT('Ctrl Pts',(-5.61082911345409,-0.253146591078478,
79.0751588012269));
#66380=CARTESIAN_POINT('Ctrl Pts',(-2.83055191421017,-4.85113001247338,
79.2339195634729));
#66381=CARTESIAN_POINT('Ctrl Pts',(2.54033285725292,-5.00921106675685,79.3926803257188));
#66382=CARTESIAN_POINT('Ctrl Pts',(5.58622740228054,-0.582709144400273,
79.5514410879646));
#66383=CARTESIAN_POINT('Ctrl Pts',(3.51943599520346,4.37710598599406,79.7102018502106));
#66384=CARTESIAN_POINT('Ctrl Pts',(-1.7684507372563,5.33086001756339,79.8689626124564));
#66385=CARTESIAN_POINT('Ctrl Pts',(-5.43779733694764,1.40564812781938,80.0277233747023));
#66386=CARTESIAN_POINT('Ctrl Pts',(-4.13030571418267,-3.80605586458648,
80.1864841369483));
#66387=CARTESIAN_POINT('Ctrl Pts',(0.95736786003426,-5.53434127223174,80.345244899194));
#66388=CARTESIAN_POINT('Ctrl Pts',(5.16882912556325,-2.19742849887699,80.5040056614401));
#66389=CARTESIAN_POINT('Ctrl Pts',(4.64962009144032,3.15063795798068,80.6627664236858));
#66390=CARTESIAN_POINT('Ctrl Pts',(-0.125063274873211,5.61514431819889,
80.8215271859319));
#66391=CARTESIAN_POINT('Ctrl Pts',(-4.78528491189737,2.9404990815964,80.9802879481776));
#66392=CARTESIAN_POINT('Ctrl Pts',(-5.06586762915643,-2.42538073321897,
81.1390487104236));
#66393=CARTESIAN_POINT('Ctrl Pts',(-0.710013553204522,-5.5714780167311,
81.2978094726694));
#66394=CARTESIAN_POINT('Ctrl Pts',(4.29566661416096,-3.61838843639986,81.4565702349154));
#66395=CARTESIAN_POINT('Ctrl Pts',(5.36982148364171,1.64636076619313,81.6153309971612));
#66396=CARTESIAN_POINT('Ctrl Pts',(1.52935170749991,5.4043103065256,81.7740917594071));
#66397=CARTESIAN_POINT('Ctrl Pts',(-3.71082746511973,4.21606997808528,81.932852521653));
#66398=CARTESIAN_POINT('Ctrl Pts',(-5.55474399465067,-0.830846376919461,
82.0916132838989));
#66399=CARTESIAN_POINT('Ctrl Pts',(-2.3147891451765,-5.11734674715333,82.2503740461448));
#66400=CARTESIAN_POINT('Ctrl Pts',(3.04373142991963,-4.72029506698704,82.4091348083907));
#66401=CARTESIAN_POINT('Ctrl Pts',(5.61653604023885,-0.00308515058908493,
82.5678955706366));
#66402=CARTESIAN_POINT('Ctrl Pts',(3.04891528446413,4.71694837524191,82.7266563328824));
#66403=CARTESIAN_POINT('Ctrl Pts',(-2.30916582642725,5.11988669499558,82.8854170951283));
#66404=CARTESIAN_POINT('Ctrl Pts',(-5.55382792200581,0.836948268868883,
83.0441778573743));
#66405=CARTESIAN_POINT('Ctrl Pts',(-3.71545689970117,-4.21199067509615,
83.2029386196201));
#66406=CARTESIAN_POINT('Ctrl Pts',(1.52341346128536,-5.40598729308003,83.3616993818661));
#66407=CARTESIAN_POINT('Ctrl Pts',(5.36800987538946,-1.65225883547266,83.5204601441119));
#66408=CARTESIAN_POINT('Ctrl Pts',(4.29963856085619,3.61366665531133,83.6792209063577));
#66409=CARTESIAN_POINT('Ctrl Pts',(-0.703891148427739,5.57225542504627,
83.8379816686037));
#66410=CARTESIAN_POINT('Ctrl Pts',(-5.06320229660515,2.43094317454181,83.9967424308495));
#66411=CARTESIAN_POINT('Ctrl Pts',(-4.78850815696806,-2.93523745070957,
84.1555031930955));
#66412=CARTESIAN_POINT('Ctrl Pts',(-0.131240194167233,-5.61500881902578,
84.3142639553413));
#66413=CARTESIAN_POINT('Ctrl Pts',(4.64617174185204,-3.15573399420934,84.4730247175873));
#66414=CARTESIAN_POINT('Ctrl Pts',(5.17120995324134,2.19172933227414,84.6317854798331));
#66415=CARTESIAN_POINT('Ctrl Pts',(0.963505020594375,5.53332329484411,84.790546242079));
#66416=CARTESIAN_POINT('Ctrl Pts',(-4.12623247316118,3.81052000369223,84.949307004325));
#66417=CARTESIAN_POINT('Ctrl Pts',(-5.43912651173278,-1.39953714320699,
85.1080677665708));
#66418=CARTESIAN_POINT('Ctrl Pts',(-1.77471179476972,-5.32917485889023,
85.2668285288167));
#66419=CARTESIAN_POINT('Ctrl Pts',(3.51540237664497,-4.38046992755931,85.4255892910626));
#66420=CARTESIAN_POINT('Ctrl Pts',(5.58537377992907,0.575612579899635,85.5843500533083));
#66421=CARTESIAN_POINT('Ctrl Pts',(2.54870583510895,5.00827077132932,85.7431108155546));
#66422=CARTESIAN_POINT('Ctrl Pts',(-2.83087179085208,4.8505389297872,85.9018715778));
#66423=CARTESIAN_POINT('Ctrl Pts',(-5.13713439629382,1.0315398004976,86.0341722130053));
#66424=CARTESIAN_POINT('Ctrl Pts',(-4.44488369978034,-2.16782829859426,
86.140012721169));
#66425=CARTESIAN_POINT('Ctrl Pts',(-3.40222835107896,-3.41035291299011,
86.1929329752511));
#66426=CARTESIAN_POINT('Ctrl Pts',(-2.75898463274135,-3.86904481704426,
86.219393102292));
#66427=CARTESIAN_POINT('Ctrl Pts',(-2.16917135428577,4.44050218283316,26.));
#66428=CARTESIAN_POINT('Ctrl Pts',(-2.90742207776898,4.07986902565299,26.026460127041));
#66429=CARTESIAN_POINT('Ctrl Pts',(-4.18934766522561,2.98339209614179,26.0793803811229));
#66430=CARTESIAN_POINT('Ctrl Pts',(-5.44619024033903,-0.180386727026251,
26.1852208892869));
#66431=CARTESIAN_POINT('Ctrl Pts',(-3.73289165771545,-4.49218988265986,
26.3175215244917));
#66432=CARTESIAN_POINT('Ctrl Pts',(1.7587897347136,-5.57324416600043,26.4762822867377));
#66433=CARTESIAN_POINT('Ctrl Pts',(5.63139102185651,-1.54490260103424,26.6350430489835));
#66434=CARTESIAN_POINT('Ctrl Pts',(4.35479274028667,3.89299966074075,26.7938038112295));
#66435=CARTESIAN_POINT('Ctrl Pts',(-0.909953676412603,5.770185632809,26.9525645734753));
#66436=CARTESIAN_POINT('Ctrl Pts',(-5.34057378621867,2.36513448582097,27.1113253357212));
#66437=CARTESIAN_POINT('Ctrl Pts',(-4.88402091610239,-3.20394040614541,
27.2700860979671));
#66438=CARTESIAN_POINT('Ctrl Pts',(0.0428938108868349,-5.84099464142013,
27.428846860213));
#66439=CARTESIAN_POINT('Ctrl Pts',(4.93036456360867,-3.13202328336963,27.5876076224589));
#66440=CARTESIAN_POINT('Ctrl Pts',(5.30551230831797,2.44338327902792,27.7463683847048));
#66441=CARTESIAN_POINT('Ctrl Pts',(0.824842359969521,5.78257686590837,27.9051291469507));
#66442=CARTESIAN_POINT('Ctrl Pts',(-4.41072200448754,3.82935543872663,28.0638899091965));
#66443=CARTESIAN_POINT('Ctrl Pts',(-5.60947270247999,-1.62859650629097,
28.2226506714425));
#66444=CARTESIAN_POINT('Ctrl Pts',(-1.67425541405712,-5.59601373441819,
28.3814114336883));
#66445=CARTESIAN_POINT('Ctrl Pts',(3.79328779764178,-4.44178483963319,28.5401721959342));
#66446=CARTESIAN_POINT('Ctrl Pts',(5.78910011906805,0.777699430509262,28.6989329581801));
#66447=CARTESIAN_POINT('Ctrl Pts',(2.48655015281781,5.28541035916478,28.8576937204261));
#66448=CARTESIAN_POINT('Ctrl Pts',(-3.09176592905605,4.95575179531496,29.0164544826718));
#66449=CARTESIAN_POINT('Ctrl Pts',(-5.84040367375386,0.0904380671616019,
29.1752152449178));
#66450=CARTESIAN_POINT('Ctrl Pts',(-3.24372543242543,-4.85764747523187,
29.3339760071636));
#66451=CARTESIAN_POINT('Ctrl Pts',(2.32170932913062,-5.35986560023234,29.4927367694096));
#66452=CARTESIAN_POINT('Ctrl Pts',(5.76224483502612,-0.956571044848404,
29.6514975316554));
#66453=CARTESIAN_POINT('Ctrl Pts',(3.92899783701638,4.32220656851071,29.8102582939014));
#66454=CARTESIAN_POINT('Ctrl Pts',(-1.50018798335741,5.64516869698926,29.9690190561472));
#66455=CARTESIAN_POINT('Ctrl Pts',(-5.55635594320173,1.80150000520858,30.1277798183931));
#66456=CARTESIAN_POINT('Ctrl Pts',(-4.52717721976122,-3.69095652156115,
30.286540580639));
#66457=CARTESIAN_POINT('Ctrl Pts',(0.645412378085751,-5.80533689665976,
30.4453013428849));
#66458=CARTESIAN_POINT('Ctrl Pts',(5.22730085393893,-2.60649561834369,30.6040621051308));
#66459=CARTESIAN_POINT('Ctrl Pts',(5.02500391786172,2.97789006670843,30.7628228673767));
#66460=CARTESIAN_POINT('Ctrl Pts',(0.223669905634492,5.83681980167278,30.9215836296225));
#66461=CARTESIAN_POINT('Ctrl Pts',(-4.78237363643064,3.35371376626822,31.0803443918685));
#66462=CARTESIAN_POINT('Ctrl Pts',(-5.41144274686964,-2.19881354860029,
31.2391051541144));
#66463=CARTESIAN_POINT('Ctrl Pts',(-1.08779416073393,-5.73891954012705,
31.3978659163602));
#66464=CARTESIAN_POINT('Ctrl Pts',(4.23143686842713,-4.0265910709645,31.5566266786062));
#66465=CARTESIAN_POINT('Ctrl Pts',(5.67792762467303,1.37099654017823,31.715387440852));
#66466=CARTESIAN_POINT('Ctrl Pts',(1.92780558426513,5.51380624011119,31.8741482030979));
#66467=CARTESIAN_POINT('Ctrl Pts',(-3.58670301245285,4.61021204769197,32.0329089653438));
#66468=CARTESIAN_POINT('Ctrl Pts',(-5.81855145490275,-0.512789031536669,
32.1916697275897));
#66469=CARTESIAN_POINT('Ctrl Pts',(-2.72508387585791,-5.16646992575742,
32.3504304898355));
#66470=CARTESIAN_POINT('Ctrl Pts',(2.86246370514321,-5.09163973204659,32.5091912520815));
#66471=CARTESIAN_POINT('Ctrl Pts',(5.83019706810478,-0.35678532940591,32.6679520143274));
#66472=CARTESIAN_POINT('Ctrl Pts',(3.46195598864868,4.7046099048568,32.8267127765732));
#66473=CARTESIAN_POINT('Ctrl Pts',(-2.0747729584413,5.46020245001391,32.9854735388191));
#66474=CARTESIAN_POINT('Ctrl Pts',(-5.71260631920057,1.21845092886281,33.144234301065));
#66475=CARTESIAN_POINT('Ctrl Pts',(-4.12208788279547,-4.13846410045175,
33.3029950633109));
#66476=CARTESIAN_POINT('Ctrl Pts',(1.24109129475792,-5.70773037400097,33.4617558255568));
#66477=CARTESIAN_POINT('Ctrl Pts',(5.46838580972161,-2.05310746437012,33.6205165878027));
#66478=CARTESIAN_POINT('Ctrl Pts',(4.69084659760865,3.48058210963631,33.7792773500486));
#66479=CARTESIAN_POINT('Ctrl Pts',(-0.379898704410712,5.82873662113877,
33.9380381122945));
#66480=CARTESIAN_POINT('Ctrl Pts',(-5.1029491079964,2.8422533358967,34.0967988745404));
#66481=CARTESIAN_POINT('Ctrl Pts',(-5.15562461633369,-2.74554702011659,
34.2555596367863));
#66482=CARTESIAN_POINT('Ctrl Pts',(-0.489714995198005,-5.82053887949348,
34.4143203990321));
#66483=CARTESIAN_POINT('Ctrl Pts',(4.62439674808221,-3.56839576568293,34.573081161278));
#66484=CARTESIAN_POINT('Ctrl Pts',(5.50611933347969,1.94965215094856,34.7318419235239));
#66485=CARTESIAN_POINT('Ctrl Pts',(1.3484733182716,5.68331886613153,34.8906026857698));
#66486=CARTESIAN_POINT('Ctrl Pts',(-4.04333666747246,4.2154385557958,35.0493634480157));
#66487=CARTESIAN_POINT('Ctrl Pts',(-5.73456142981912,-1.11053988305151,
35.2081242102616));
#66488=CARTESIAN_POINT('Ctrl Pts',(-2.17734040713567,-5.42011829904768,
35.3668849725075));
#66489=CARTESIAN_POINT('Ctrl Pts',(3.37264906388706,-4.76903888808624,35.5256457347534));
#66490=CARTESIAN_POINT('Ctrl Pts',(5.83588709273329,0.246810585441287,35.6844064969993));
#66491=CARTESIAN_POINT('Ctrl Pts',(2.95794299481775,5.03677147224547,35.8431672592451));
#66492=CARTESIAN_POINT('Ctrl Pts',(-2.62720088350026,5.21692525746274,36.001928021491));
#66493=CARTESIAN_POINT('Ctrl Pts',(-5.80785026434291,0.622389693993225,
36.160688783737));
#66494=CARTESIAN_POINT('Ctrl Pts',(-3.67297768016272,-4.54177592855961,
36.3194495459828));
#66495=CARTESIAN_POINT('Ctrl Pts',(1.82351626946645,-5.54916949094261,36.4782103082287));
#66496=CARTESIAN_POINT('Ctrl Pts',(5.65107242925025,-1.47779363362579,36.6369710704746));
#66497=CARTESIAN_POINT('Ctrl Pts',(4.30659448752927,3.94610409697964,36.7957318327205));
#66498=CARTESIAN_POINT('Ctrl Pts',(-0.979410275819905,5.7584068227102,36.9544925949664));
#66499=CARTESIAN_POINT('Ctrl Pts',(-5.36902883826232,2.30043973146977,37.1132533572123));
#66500=CARTESIAN_POINT('Ctrl Pts',(-4.84474820880581,-3.26296006985836,
37.2720141194581));
#66501=CARTESIAN_POINT('Ctrl Pts',(0.113593966110691,-5.839999146839,37.4307748817041));
#66502=CARTESIAN_POINT('Ctrl Pts',(4.96797147346979,-3.07209261953597,37.5895356439499));
#66503=CARTESIAN_POINT('Ctrl Pts',(5.27550973964484,2.50748691145728,37.7482964061959));
#66504=CARTESIAN_POINT('Ctrl Pts',(0.754740349553719,5.79213782889985,37.9070571684417));
#66505=CARTESIAN_POINT('Ctrl Pts',(-4.4567904622931,3.77564728217961,38.0658179306876));
#66506=CARTESIAN_POINT('Ctrl Pts',(-5.58933050861204,-1.69643098583928,
38.2245786929334));
#66507=CARTESIAN_POINT('Ctrl Pts',(-1.60634454512588,-5.6158837974589,38.3833394551794));
#66508=CARTESIAN_POINT('Ctrl Pts',(3.84681701249253,-4.39550821823998,38.5421002174252));
#66509=CARTESIAN_POINT('Ctrl Pts',(5.77925413772213,0.847770744858901,38.7008609796712));
#66510=CARTESIAN_POINT('Ctrl Pts',(2.42234134649229,5.31514402676831,38.859621741917));
#66511=CARTESIAN_POINT('Ctrl Pts',(-3.15157223642715,4.91793514219116,39.018382504163));
#66512=CARTESIAN_POINT('Ctrl Pts',(-5.84107064254106,0.0196817951957224,
39.1771432664088));
#66513=CARTESIAN_POINT('Ctrl Pts',(-3.18464277877548,-4.89658493195106,
39.3359040286547));
#66514=CARTESIAN_POINT('Ctrl Pts',(2.38646743230569,-5.33134756124203,39.4946647909006));
#66515=CARTESIAN_POINT('Ctrl Pts',(5.77340975374383,-0.886698054352646,
39.6534255531465));
#66516=CARTESIAN_POINT('Ctrl Pts',(3.87635111745847,4.36948459642503,39.8121863153924));
#66517=CARTESIAN_POINT('Ctrl Pts',(-1.56846246621147,5.62658147690965,39.9709470776383));
#66518=CARTESIAN_POINT('Ctrl Pts',(-5.57777129149482,1.73405912355756,40.1297078398841));
#66519=CARTESIAN_POINT('Ctrl Pts',(-4.48213345555963,-3.74552710720003,
40.2884686021301));
#66520=CARTESIAN_POINT('Ctrl Pts',(0.7156898274528,-5.79709252083298,40.4472293643759));
#66521=CARTESIAN_POINT('Ctrl Pts',(5.25849191934999,-2.5429817849029,40.6059901266219));
#66522=CARTESIAN_POINT('Ctrl Pts',(4.98856158393098,3.03854355696032,40.7647508888677));
#66523=CARTESIAN_POINT('Ctrl Pts',(0.152947309300711,5.83910102197203,40.9235116511136));
#66524=CARTESIAN_POINT('Ctrl Pts',(-4.82264901463799,3.29553487401187,41.0822724133595));
#66525=CARTESIAN_POINT('Ctrl Pts',(-5.38440965064774,-2.26420545406742,
41.2410331756054));
#66526=CARTESIAN_POINT('Ctrl Pts',(-1.0181941054504,-5.75167578952804,41.3997939378513));
#66527=CARTESIAN_POINT('Ctrl Pts',(4.27990378619904,-3.97503675518808,41.5585547000972));
#66528=CARTESIAN_POINT('Ctrl Pts',(5.66090300135578,1.43967733657867,41.7173154623431));
#66529=CARTESIAN_POINT('Ctrl Pts',(1.86087087513805,5.53675475439179,41.8760762245889));
#66530=CARTESIAN_POINT('Ctrl Pts',(-3.64228711704701,4.56642509860946,42.0348369868349));
#66531=CARTESIAN_POINT('Ctrl Pts',(-5.81191268460203,-0.583236290691027,
42.1935977490807));
#66532=CARTESIAN_POINT('Ctrl Pts',(-2.66229823602482,-5.19910201156664,
42.3523585113267));
#66533=CARTESIAN_POINT('Ctrl Pts',(2.92393287912081,-5.05659076281771,42.5111192735725));
#66534=CARTESIAN_POINT('Ctrl Pts',(5.83409131060233,-0.286133192362046,
42.6698800358184));
#66535=CARTESIAN_POINT('Ctrl Pts',(3.4047111699812,4.74620221579552,42.8286407980643));
#66536=CARTESIAN_POINT('Ctrl Pts',(-2.14076463166355,5.43466838142269,42.9874015603102));
#66537=CARTESIAN_POINT('Ctrl Pts',(-5.72694725190272,1.1491600402646,43.1461623225561));
#66538=CARTESIAN_POINT('Ctrl Pts',(-4.07165281531897,-4.18809467129411,
43.3049230848019));
#66539=CARTESIAN_POINT('Ctrl Pts',(1.31014264809932,-5.69227721266703,43.4636838470478));
#66540=CARTESIAN_POINT('Ctrl Pts',(5.49285554114887,-1.98671377613569,43.6224446092938));
#66541=CARTESIAN_POINT('Ctrl Pts',(4.64833926148183,3.53715079327751,43.7812053715396));
#66542=CARTESIAN_POINT('Ctrl Pts',(-0.450479095664875,5.82370691300532,
43.9399661337855));
#66543=CARTESIAN_POINT('Ctrl Pts',(-5.13700522439592,2.78022857850681,44.0987268960314));
#66544=CARTESIAN_POINT('Ctrl Pts',(-5.12198725989218,-2.80779987422883,
44.2574876582773));
#66545=CARTESIAN_POINT('Ctrl Pts',(-0.419170101997096,-5.82604411670637,
44.4162484205232));
#66546=CARTESIAN_POINT('Ctrl Pts',(4.66728433696318,-3.51211482473953,44.575009182769));
#66547=CARTESIAN_POINT('Ctrl Pts',(5.48209758667841,2.01620923377307,44.733769945015));
#66548=CARTESIAN_POINT('Ctrl Pts',(1.27952767221442,5.69923701562366,44.8925307072609));
#66549=CARTESIAN_POINT('Ctrl Pts',(-4.09410505154189,4.16614899531406,45.0512914695068));
#66550=CARTESIAN_POINT('Ctrl Pts',(-5.72068777605988,-1.17992584218497,
45.2100522317526));
#66551=CARTESIAN_POINT('Ctrl Pts',(-2.11152230724456,-5.4460965076122,45.3688129939986));
#66552=CARTESIAN_POINT('Ctrl Pts',(3.43017287444968,-4.72783329608889,45.5275737562444));
#66553=CARTESIAN_POINT('Ctrl Pts',(5.83246906545287,0.317487361563403,45.6863345184903));
#66554=CARTESIAN_POINT('Ctrl Pts',(2.89671141266624,5.07223388813511,45.8450952807362));
#66555=CARTESIAN_POINT('Ctrl Pts',(-2.69020500619468,5.1847170268841,46.003856042982));
#66556=CARTESIAN_POINT('Ctrl Pts',(-5.8149636300044,0.551988773385138,46.162616805228));
#66557=CARTESIAN_POINT('Ctrl Pts',(-3.61768991925726,-4.58593646623255,
46.3213775674738));
#66558=CARTESIAN_POINT('Ctrl Pts',(1.89060410937151,-5.5266725727009,46.4801383297198));
#66559=CARTESIAN_POINT('Ctrl Pts',(5.66855950784905,-1.40922912622162,46.6388990919655));
#66560=CARTESIAN_POINT('Ctrl Pts',(4.25847609633845,3.99798386203986,46.7976598542116));
#66561=CARTESIAN_POINT('Ctrl Pts',(-1.04909471538713,5.74611989975528,46.9564206164574));
#66562=CARTESIAN_POINT('Ctrl Pts',(-5.39650199857509,2.23523148769702,47.1151813787033));
#66563=CARTESIAN_POINT('Ctrl Pts',(-4.80486581436728,-3.32140905793637,
47.2739421409491));
#66564=CARTESIAN_POINT('Ctrl Pts',(0.184330329686807,-5.83819457998573,
47.4327029031951));
#66565=CARTESIAN_POINT('Ctrl Pts',(5.00482172556827,-3.01168609245668,47.5914636654409));
#66566=CARTESIAN_POINT('Ctrl Pts',(5.24474740393951,2.5712095000382,47.7502244276869));
#66567=CARTESIAN_POINT('Ctrl Pts',(0.684520055329939,5.80085561948134,47.9089851899327));
#66568=CARTESIAN_POINT('Ctrl Pts',(-4.50220095685495,3.72138148653313,48.0677459521787));
#66569=CARTESIAN_POINT('Ctrl Pts',(-5.56837013180732,-1.76401465396777,
48.2265067144245));
#66570=CARTESIAN_POINT('Ctrl Pts',(-1.53819687404933,-5.63493070062818,
48.3852674766705));
#66571=CARTESIAN_POINT('Ctrl Pts',(3.89978114767392,-4.3485860488743,48.5440282389163));
#66572=CARTESIAN_POINT('Ctrl Pts',(5.76856034267981,0.917717384099773,48.7027890011622));
#66573=CARTESIAN_POINT('Ctrl Pts',(2.35777690909515,5.34409783510322,48.8615497634081));
#66574=CARTESIAN_POINT('Ctrl Pts',(-3.21091597092679,4.87939670982634,49.020310525654));
#66575=CARTESIAN_POINT('Ctrl Pts',(-5.84088047565118,-0.0510773273967016,
49.1790712878999));
#66576=CARTESIAN_POINT('Ctrl Pts',(-3.12509275704243,-4.93480383440904,
49.3378320501458));
#66577=CARTESIAN_POINT('Ctrl Pts',(2.45087531001271,-5.3020471366244,49.4965928123917));
#66578=CARTESIAN_POINT('Ctrl Pts',(5.78372743038313,-0.816694946262622,
49.6553535746376));
#66579=CARTESIAN_POINT('Ctrl Pts',(3.82313554021223,4.41612140519068,49.8141143368834));
#66580=CARTESIAN_POINT('Ctrl Pts',(-1.63650677555656,5.60716855442876,49.9728750991293));
#66581=CARTESIAN_POINT('Ctrl Pts',(-5.59836810258563,1.66636376946,50.1316358613752));
#66582=CARTESIAN_POINT('Ctrl Pts',(-4.43643193774801,-3.79954803706259,
50.2903966236211));
#66583=CARTESIAN_POINT('Ctrl Pts',(0.785862249094534,-5.78799742135959,
50.4491573858669));
#66584=CARTESIAN_POINT('Ctrl Pts',(5.28891130109086,-2.47909476894502,50.6079181481129));
#66585=CARTESIAN_POINT('Ctrl Pts',(4.95138717842959,3.0987511409437,50.7666789103587));
#66586=CARTESIAN_POINT('Ctrl Pts',(0.0822022679789686,5.84052535405474,
50.9254396726047));
#66587=CARTESIAN_POINT('Ctrl Pts',(-4.86221666902701,3.23687236196503,51.0842004348505));
#66588=CARTESIAN_POINT('Ctrl Pts',(-5.35658639219748,-2.32926508734879,
51.2429611970965));
#66589=CARTESIAN_POINT('Ctrl Pts',(-0.948444630167017,-5.76358798039247,
51.4017219593423));
#66590=CARTESIAN_POINT('Ctrl Pts',(4.32774262801073,-3.92289910269379,51.5604827215883));
#66591=CARTESIAN_POINT('Ctrl Pts',(5.64304764041327,1.50814686030353,51.7192434838341));
#66592=CARTESIAN_POINT('Ctrl Pts',(1.79366308317505,5.55889074980541,51.87800424608));
#66593=CARTESIAN_POINT('Ctrl Pts',(-3.69733671593728,4.52196802655651,52.0367650083259));
#66594=CARTESIAN_POINT('Ctrl Pts',(-5.80442101600325,-0.653597959908777,
52.1955257705718));
#66595=CARTESIAN_POINT('Ctrl Pts',(-2.59912190387458,-5.2309711290559,52.3542865328177));
#66596=CARTESIAN_POINT('Ctrl Pts',(2.98497296589237,-5.02079973879747,52.5130472950635));
#66597=CARTESIAN_POINT('Ctrl Pts',(5.83712940008821,-0.215439065266698,
52.6718080573094));
#66598=CARTESIAN_POINT('Ctrl Pts',(3.34696670988424,4.78709802146808,52.8305688195553));
#66599=CARTESIAN_POINT('Ctrl Pts',(-2.20644214763509,5.4083367751423,52.9893295818012));
#66600=CARTESIAN_POINT('Ctrl Pts',(-5.74044775498584,1.07970051240847,53.1480903440471));
#66601=CARTESIAN_POINT('Ctrl Pts',(-4.02062023271376,-4.2371106391632,53.306851106293));
#66602=CARTESIAN_POINT('Ctrl Pts',(1.37900173798208,-5.675988709543,53.4656118685389));
#66603=CARTESIAN_POINT('Ctrl Pts',(5.51651919592013,-1.92002853761645,53.6243726307848));
#66604=CARTESIAN_POINT('Ctrl Pts',(4.60514978147925,3.59320039997198,53.7831333930307));
#66605=CARTESIAN_POINT('Ctrl Pts',(-0.520993379103106,5.81782257577076,
53.9418941552766));
#66606=CARTESIAN_POINT('Ctrl Pts',(-5.1703074851803,2.71779582251969,54.1006549175224));
#66607=CARTESIAN_POINT('Ctrl Pts',(-5.08759825172204,-2.86964068365571,
54.2594156797684));
#66608=CARTESIAN_POINT('Ctrl Pts',(-0.348563695575712,-5.83069438183342,
54.4181764420142));
#66609=CARTESIAN_POINT('Ctrl Pts',(4.70948700177826,-3.45531848087826,54.5769372042601));
#66610=CARTESIAN_POINT('Ctrl Pts',(5.45727134195117,2.08247043785393,54.735697966506));
#66611=CARTESIAN_POINT('Ctrl Pts',(1.21039425544677,5.71431880197442,54.8944587287519));
#66612=CARTESIAN_POINT('Ctrl Pts',(-4.14427262561643,4.11624805238744,55.0532194909978));
#66613=CARTESIAN_POINT('Ctrl Pts',(-5.70597461125989,-1.24913864717843,
55.2119802532437));
#66614=CARTESIAN_POINT('Ctrl Pts',(-2.04539434141439,-5.47127550140978,
55.3707410154896));
#66615=CARTESIAN_POINT('Ctrl Pts',(3.48719330707719,-4.68593389446471,55.5295017777355));
#66616=CARTESIAN_POINT('Ctrl Pts',(5.82819512322526,0.388117546408988,55.6882625399813));
#66617=CARTESIAN_POINT('Ctrl Pts',(2.83505473805949,5.10695195360438,55.8470233022273));
#66618=CARTESIAN_POINT('Ctrl Pts',(-2.75281434125286,5.15174793898243,56.0057840644731));
#66619=CARTESIAN_POINT('Ctrl Pts',(-5.82122364964165,0.481506848414017,
56.1645448267191));
#66620=CARTESIAN_POINT('Ctrl Pts',(-3.56187126228685,-4.6294240176411,56.3233055889649));
#66621=CARTESIAN_POINT('Ctrl Pts',(1.95741450308725,-5.50336461515325,56.4820663512108));
#66622=CARTESIAN_POINT('Ctrl Pts',(5.6852147252314,-1.34045781441613,56.6408271134567));
#66623=CARTESIAN_POINT('Ctrl Pts',(4.20973277369882,4.0492769228917,56.7995878757026));
#66624=CARTESIAN_POINT('Ctrl Pts',(-1.11862520028478,5.73298973359492,56.9583486379484));
#66625=CARTESIAN_POINT('Ctrl Pts',(-5.42318322211612,2.16969522366057,57.1171094001944));
#66626=CARTESIAN_POINT('Ctrl Pts',(-4.76427830577834,-3.3793706291715,57.2758701624402));
#66627=CARTESIAN_POINT('Ctrl Pts',(0.255039642783455,-5.83553325796587,
57.4346309246862));
#66628=CARTESIAN_POINT('Ctrl Pts',(5.04093751998252,-2.95083760038564,57.593391686932));
#66629=CARTESIAN_POINT('Ctrl Pts',(5.21321540145215,2.63455476357568,57.7521524491779));
#66630=CARTESIAN_POINT('Ctrl Pts',(0.614199307774883,5.80872213438946,57.9109132114238));
#66631=CARTESIAN_POINT('Ctrl Pts',(-4.54695075334007,3.66656957808212,58.0696739736697));
#66632=CARTESIAN_POINT('Ctrl Pts',(-5.54659259657899,-1.83133945291199,
58.2284347359156));
#66633=CARTESIAN_POINT('Ctrl Pts',(-1.469823472552,-5.65315067760911,58.3871954981615));
#66634=CARTESIAN_POINT('Ctrl Pts',(3.95217298989717,-4.30102572442254,58.5459562604074));
#66635=CARTESIAN_POINT('Ctrl Pts',(5.75702001129657,0.987529348296885,58.7047170226532));
#66636=CARTESIAN_POINT('Ctrl Pts',(2.29286646789146,5.37226739697831,58.8634777848992));
#66637=CARTESIAN_POINT('Ctrl Pts',(-3.26978850344612,4.84014222590088,59.022238547145));
#66638=CARTESIAN_POINT('Ctrl Pts',(-5.83983315943952,-0.121828954390395,
59.180999309391));
#66639=CARTESIAN_POINT('Ctrl Pts',(-3.06508412788734,-4.97229855430969,
59.3397600716368));
#66640=CARTESIAN_POINT('Ctrl Pts',(2.51492352172104,-5.27196863648781,59.4985208338828));
#66641=CARTESIAN_POINT('Ctrl Pts',(5.79319634491114,-0.746571988173542,
59.6572815961285));
#66642=CARTESIAN_POINT('Ctrl Pts',(3.76935891775212,4.46211014805548,59.8160423583745));
#66643=CARTESIAN_POINT('Ctrl Pts',(-1.70431092750091,5.58693277985496,59.9748031206203));
#66644=CARTESIAN_POINT('Ctrl Pts',(-5.61814335305001,1.59842387644741,60.1335638828663));
#66645=CARTESIAN_POINT('Ctrl Pts',(-4.39007937346456,-3.85301138317786,
60.2923246451121));
#66646=CARTESIAN_POINT('Ctrl Pts',(0.85591934543619,-5.77805293315363,60.451085407358));
#66647=CARTESIAN_POINT('Ctrl Pts',(5.31855453499689,-2.41484394578226,60.609846169604));
#66648=CARTESIAN_POINT('Ctrl Pts',(4.91348615676483,3.15850398313777,60.7686069318498));
#66649=CARTESIAN_POINT('Ctrl Pts',(0.0114451634727917,5.84109258892977,
60.9273676940957));
#66650=CARTESIAN_POINT('Ctrl Pts',(-4.90107079302665,3.17773483883697,61.0861284563416));
#66651=CARTESIAN_POINT('Ctrl Pts',(-5.32797705459145,-2.3939829009339,61.2448892185875));
#66652=CARTESIAN_POINT('Ctrl Pts',(-0.878555970616003,-5.77465436461024,
61.4036499808334));
#66653=CARTESIAN_POINT('Ctrl Pts',(4.37494637350877,-3.87018576468102,61.5624107430792));
#66654=CARTESIAN_POINT('Ctrl Pts',(5.62436416212133,1.57639506344776,61.7211715053253));
#66655=CARTESIAN_POINT('Ctrl Pts',(1.72619207112014,5.58021097789493,61.879932267571));
#66656=CARTESIAN_POINT('Ctrl Pts',(-3.75184373059352,4.47684735560896,62.038693029817));
#66657=CARTESIAN_POINT('Ctrl Pts',(-5.79607754850909,-0.723863713613315,
62.1974537920628));
#66658=CARTESIAN_POINT('Ctrl Pts',(-2.53556415053518,-5.26207260143168,
62.3562145543087));
#66659=CARTESIAN_POINT('Ctrl Pts',(3.04557500782399,-4.9842719123193,62.5149753165546));
#66660=CARTESIAN_POINT('Ctrl Pts',(5.8393108907227,-0.144713322484355,62.6737360788005));
#66661=CARTESIAN_POINT('Ctrl Pts',(3.28873108235841,4.82729132041423,62.8324968410464));
#66662=CARTESIAN_POINT('Ctrl Pts',(-2.27179586817918,5.38121149533645,62.9912576032922));
#66663=CARTESIAN_POINT('Ctrl Pts',(-5.75310584725087,1.01008253848138,63.1500183655383));
#66664=CARTESIAN_POINT('Ctrl Pts',(-3.96899762401232,-4.28550481096468,
63.3087791277839));
#66665=CARTESIAN_POINT('Ctrl Pts',(1.44765845933327,-5.65886725496703,63.4675398900301));
#66666=CARTESIAN_POINT('Ctrl Pts',(5.53937330139366,-1.85306153487257,63.6263006522757));
#66667=CARTESIAN_POINT('Ctrl Pts',(4.56128449565793,3.64872270443888,63.7850614145219));
#66668=CARTESIAN_POINT('Ctrl Pts',(-0.591431206752995,5.81108447296164,
63.9438221767675));
#66669=CARTESIAN_POINT('Ctrl Pts',(-5.20285100324211,2.65496422994348,64.1025829390136));
#66670=CARTESIAN_POINT('Ctrl Pts',(-5.05246263841092,-2.93106037325727,
64.2613437012593));
#66671=CARTESIAN_POINT('Ctrl Pts',(-0.277906137425253,-5.83448899244814,
64.4201044635054));
#66672=CARTESIAN_POINT('Ctrl Pts',(4.75099854928546,-3.3980150689637,64.5788652257511));
#66673=CARTESIAN_POINT('Ctrl Pts',(5.4316442425499,2.14842603935805,64.7376259879971));
#66674=CARTESIAN_POINT('Ctrl Pts',(1.14108321329899,5.72856201193147,64.896386750243));
#66675=CARTESIAN_POINT('Ctrl Pts',(-4.19383202760378,4.06574304998017,65.0551475124888));
#66676=CARTESIAN_POINT('Ctrl Pts',(-5.69042409457625,-1.31816814105151,
65.2139082747347));
#66677=CARTESIAN_POINT('Ctrl Pts',(-1.97896621392534,-5.49565158542271,
65.3726690369806));
#66678=CARTESIAN_POINT('Ctrl Pts',(3.54370199402013,-4.6433468319516,65.5314297992266));
#66679=CARTESIAN_POINT('Ctrl Pts',(5.82306589325152,0.458690774997357,65.6901905614723));
#66680=CARTESIAN_POINT('Ctrl Pts',(2.77298201911554,5.14092057377652,65.8489513237183));
#66681=CARTESIAN_POINT('Ctrl Pts',(-2.8150197007537,5.11802283197194,66.0077120859641));
#66682=CARTESIAN_POINT('Ctrl Pts',(-5.8266294045968,0.410954262303533,66.1664728482102));
#66683=CARTESIAN_POINT('Ctrl Pts',(-3.50552990064023,-4.67223220098639,
66.3252336104559));
#66684=CARTESIAN_POINT('Ctrl Pts',(2.0239376461872,-5.47924903874272,66.483994372702));
#66685=CARTESIAN_POINT('Ctrl Pts',(5.70103563724385,-1.27148979040063,66.6427551349476));
#66686=CARTESIAN_POINT('Ctrl Pts',(4.16037167269387,4.09997575227756,66.8015158971937));
#66687=CARTESIAN_POINT('Ctrl Pts',(-1.18799152691301,5.71901825108119,66.9602766594395));
#66688=CARTESIAN_POINT('Ctrl Pts',(-5.44906859341531,2.10384055680833,67.1190374216854));
#66689=CARTESIAN_POINT('Ctrl Pts',(-4.72299163925665,-3.43683627770202,
67.2777981839313));
#66690=CARTESIAN_POINT('Ctrl Pts',(0.325711528807802,-5.8320155713286,67.4365589461772));
#66691=CARTESIAN_POINT('Ctrl Pts',(5.07631355671921,-2.88955607283996,67.5953197084231));
#66692=CARTESIAN_POINT('Ctrl Pts',(5.18091835950451,2.6975134061513,67.754080470669));
#66693=CARTESIAN_POINT('Ctrl Pts',(0.54378842645952,5.81573621921296,67.9128412329148));
#66694=CARTESIAN_POINT('Ctrl Pts',(-4.59103328471497,3.61121960047518,68.0716019951608));
#66695=CARTESIAN_POINT('Ctrl Pts',(-5.52400109878079,-1.8983955027565,68.2303627574066));
#66696=CARTESIAN_POINT('Ctrl Pts',(-1.40123437443171,-5.67054105461978,
68.3891235196526));
#66697=CARTESIAN_POINT('Ctrl Pts',(4.00398485065851,-4.2528342243631,68.5478842818984));
#66698=CARTESIAN_POINT('Ctrl Pts',(5.74463483711628,1.05719639254342,68.7066450441444));
#66699=CARTESIAN_POINT('Ctrl Pts',(2.22761954848948,5.39964857850993,68.8654058063901));
#66700=CARTESIAN_POINT('Ctrl Pts',(-3.32818119444006,4.80017745101086,69.0241665686361));
#66701=CARTESIAN_POINT('Ctrl Pts',(-5.83792884759976,-0.192562702982879,
69.182927330882));
#66702=CARTESIAN_POINT('Ctrl Pts',(-3.00462569757752,-5.00906358930226,
69.3416880931278));
#66703=CARTESIAN_POINT('Ctrl Pts',(2.57860266835449,-5.24111647485266,69.5004488553739));
#66704=CARTESIAN_POINT('Ctrl Pts',(5.80181510776444,-0.676339470630766,
69.6592096176196));
#66705=CARTESIAN_POINT('Ctrl Pts',(3.71502914179852,4.50744407617051,69.8179703798656));
#66706=CARTESIAN_POINT('Ctrl Pts',(-1.77186497178415,5.56587712278864,69.9767311421114));
#66707=CARTESIAN_POINT('Ctrl Pts',(-5.63709414086971,1.53024941470006,70.1354919043573));
#66708=CARTESIAN_POINT('Ctrl Pts',(-4.34308256494864,-3.90590929979895,
70.2942526666033));
#66709=CARTESIAN_POINT('Ctrl Pts',(0.925850835597592,-5.7672605155689,70.453013428849));
#66710=CARTESIAN_POINT('Ctrl Pts',(5.34741727092293,-2.35023874422409,70.6117741910951));
#66711=CARTESIAN_POINT('Ctrl Pts',(4.87486408091236,3.21779331481187,70.7705349533408));
#66712=CARTESIAN_POINT('Ctrl Pts',(-0.0593136206115266,5.8408026433554,
70.9292957155867));
#66713=CARTESIAN_POINT('Ctrl Pts',(-4.93920568479356,3.11813098306019,71.0880564778327));
#66714=CARTESIAN_POINT('Ctrl Pts',(-5.29858583625043,-2.45834939748262,
71.2468172400784));
#66715=CARTESIAN_POINT('Ctrl Pts',(-0.808538382959287,-5.78487331818929,
71.4055780023245));
#66716=CARTESIAN_POINT('Ctrl Pts',(4.42150809554277,-3.81690447683292,71.5643387645703));
#66717=CARTESIAN_POINT('Ctrl Pts',(5.60485530828073,1.64441193058638,71.7230995268162));
#66718=CARTESIAN_POINT('Ctrl Pts',(1.65846774034549,5.6007123099165,71.8818602890621));
#66719=CARTESIAN_POINT('Ctrl Pts',(-3.80580016211055,4.43106970722601,72.040621051308));
#66720=CARTESIAN_POINT('Ctrl Pts',(-5.78688350652351,-0.794023240304163,
72.1993818135539));
#66721=CARTESIAN_POINT('Ctrl Pts',(-2.47163430310789,-5.29240186455242,
72.3581425757998));
#66722=CARTESIAN_POINT('Ctrl Pts',(3.10573011156498,-4.94701264384235,72.5169033380457));
#66723=CARTESIAN_POINT('Ctrl Pts',(5.84063546237199,-0.0739663430189528,
72.6756641002916));
#66724=CARTESIAN_POINT('Ctrl Pts',(3.23001283348305,4.86677621426665,72.8344248625374));
#66725=CARTESIAN_POINT('Ctrl Pts',(-2.33681620263615,5.35329652264041,72.9931856247833));
#66726=CARTESIAN_POINT('Ctrl Pts',(-5.76491967112249,0.940316334922364,
73.1519463870293));
#66727=CARTESIAN_POINT('Ctrl Pts',(-3.9167925648334,-4.33327008485316,73.3107071492751));
#66728=CARTESIAN_POINT('Ctrl Pts',(1.51610273677804,-5.64091536151285,73.469467911521));
#66729=CARTESIAN_POINT('Ctrl Pts',(5.56141450372903,-1.78582259531264,73.6282286737669));
#66730=CARTESIAN_POINT('Ctrl Pts',(4.51674984124932,3.70370955877901,73.7869894360128));
#66731=CARTESIAN_POINT('Ctrl Pts',(-0.661782241861996,5.80349359339467,
73.9457501982587));
#66732=CARTESIAN_POINT('Ctrl Pts',(-5.23463100281954,2.59174302131558,74.1045109605046));
#66733=CARTESIAN_POINT('Ctrl Pts',(-5.01658557611066,-2.99204992969303,
74.2632717227504));
#66734=CARTESIAN_POINT('Ctrl Pts',(-0.207207796543587,-5.83742739169134,
74.4220324849964));
#66735=CARTESIAN_POINT('Ctrl Pts',(4.79181288766461,-3.34021299827244,74.5807932472422));
#66736=CARTESIAN_POINT('Ctrl Pts',(5.4052200492518,2.21406635929985,74.7395540094881));
#66737=CARTESIAN_POINT('Ctrl Pts',(1.07160471716756,5.7419645553035,74.8983147717341));
#66738=CARTESIAN_POINT('Ctrl Pts',(-4.2427759846608,4.01464139970224,75.0570755339798));
#66739=CARTESIAN_POINT('Ctrl Pts',(-5.67403850804756,-1.38700419372482,
75.2158362962259));
#66740=CARTESIAN_POINT('Ctrl Pts',(-1.91224767310636,-5.51922118246009,
75.3745970584716));
#66741=CARTESIAN_POINT('Ctrl Pts',(3.59969064262747,-4.60007835820185,75.5333578207176));
#66742=CARTESIAN_POINT('Ctrl Pts',(5.81708212824635,0.529196690705634,75.6921185829634));
#66743=CARTESIAN_POINT('Ctrl Pts',(2.71050236500702,5.17413476375605,75.8508793452094));
#66744=CARTESIAN_POINT('Ctrl Pts',(-2.87681195605961,5.08354665501262,76.0096401074552));
#66745=CARTESIAN_POINT('Ctrl Pts',(-5.83118010157501,0.340341368647152,
76.1684008697012));
#66746=CARTESIAN_POINT('Ctrl Pts',(-3.4486741024136,-4.71435473416655,76.327161631947));
#66747=CARTESIAN_POINT('Ctrl Pts',(2.09016377639872,-5.45432938243075,76.4859223941929));
#66748=CARTESIAN_POINT('Ctrl Pts',(5.71601992216721,-1.20233517523405,76.6446831564388));
#66749=CARTESIAN_POINT('Ctrl Pts',(4.11040003706624,4.15007291014307,76.8034439186847));
#66750=CARTESIAN_POINT('Ctrl Pts',(-1.25718351576172,5.7042075025295,76.9622046809306));
#66751=CARTESIAN_POINT('Ctrl Pts',(-5.47415431379396,2.03767715131415,77.1209654431764));
#66752=CARTESIAN_POINT('Ctrl Pts',(-4.68101187362137,-3.49379757044288,
77.2797262054223));
#66753=CARTESIAN_POINT('Ctrl Pts',(0.39633561665894,-5.82764203629436,77.4384869676682));
#66754=CARTESIAN_POINT('Ctrl Pts',(5.11094464434401,-2.82785050288533,77.5972477299141));
#66755=CARTESIAN_POINT('Ctrl Pts',(5.1478610176884,2.76007618858267,77.75600849216));
#66756=CARTESIAN_POINT('Ctrl Pts',(0.473297744182263,5.82189684463481,77.9147692544059));
#66757=CARTESIAN_POINT('Ctrl Pts',(-4.63444208186731,3.55533967632268,78.0735300166519));
#66758=CARTESIAN_POINT('Ctrl Pts',(-5.50059895371541,-1.96517296302448,
78.2322907788976));
#66759=CARTESIAN_POINT('Ctrl Pts',(-1.33243964514028,-5.6870992796219,78.3910515411437));
#66760=CARTESIAN_POINT('Ctrl Pts',(4.0552091265661,-4.20401862079985,78.5498123033894));
#66761=CARTESIAN_POINT('Ctrl Pts',(5.73140663766353,1.12670829319891,78.7085730656353));
#66762=CARTESIAN_POINT('Ctrl Pts',(2.16204572587615,5.42623736150913,78.8673338278812));
#66763=CARTESIAN_POINT('Ctrl Pts',(-3.38608547477963,4.75950824998793,79.0260945901272));
#66764=CARTESIAN_POINT('Ctrl Pts',(-5.83516781958967,-0.263268192994679,
79.184855352373));
#66765=CARTESIAN_POINT('Ctrl Pts',(-2.94372633838929,-5.04509354411697,
79.3436161146189));
#66766=CARTESIAN_POINT('Ctrl Pts',(2.64190340499678,-5.2094951792744,79.5023768768649));
#66767=CARTESIAN_POINT('Ctrl Pts',(5.80958245413942,-0.606007700257848,
79.6611376391106));
#66768=CARTESIAN_POINT('Ctrl Pts',(3.66015418524723,4.55211653678098,79.8198984013567));
#66769=CARTESIAN_POINT('Ctrl Pts',(-1.8391589948488,5.54400467314773,79.9786591636023));
#66770=CARTESIAN_POINT('Ctrl Pts',(-5.65521768501588,1.46185038882208,80.1374199258485));
#66771=CARTESIAN_POINT('Ctrl Pts',(-4.29544840898361,-3.95823402415551,
80.2961806880941));
#66772=CARTESIAN_POINT('Ctrl Pts',(0.995646457131763,-5.7556217523925,80.4549414503402));
#66773=CARTESIAN_POINT('Ctrl Pts',(5.3754952732605,-2.28528864508612,80.613702212586));
#66774=CARTESIAN_POINT('Ctrl Pts',(4.83552661866532,3.27661043525698,80.7724629748319));
#66775=CARTESIAN_POINT('Ctrl Pts',(-0.130063700425983,5.83965555987772,
80.9312237370779));
#66776=CARTESIAN_POINT('Ctrl Pts',(-4.9766157480213,3.05806954150856,81.0899844993236));
#66777=CARTESIAN_POINT('Ctrl Pts',(-5.26841705035579,-2.52235513122241,
81.2487452615697));
#66778=CARTESIAN_POINT('Ctrl Pts',(-0.738402142242399,-5.79424334147416,
81.4075060238153));
#66779=CARTESIAN_POINT('Ctrl Pts',(4.46742096110774,-3.76306305822547,81.5662667860616));
#66780=CARTESIAN_POINT('Ctrl Pts',(5.58452394195224,1.71218748032981,81.7250275483071));
#66781=CARTESIAN_POINT('Ctrl Pts',(1.590500029138,5.62039173713168,81.8837883105533));
#66782=CARTESIAN_POINT('Ctrl Pts',(-3.85919809188181,4.38464179959952,82.0425490727989));
#66783=CARTESIAN_POINT('Ctrl Pts',(-5.776840240228,-0.864066244683674,82.201309835045));
#66784=CARTESIAN_POINT('Ctrl Pts',(-2.40734174146917,-5.3219544664209,82.3600705972908));
#66785=CARTESIAN_POINT('Ctrl Pts',(3.16542944584671,-4.9090274034195,82.5188313595367));
#66786=CARTESIAN_POINT('Ctrl Pts',(5.84110292736961,-0.00320850467390637,
82.6775921217826));
#66787=CARTESIAN_POINT('Ctrl Pts',(3.1708205673024,4.90554690034638,82.8363528840285));
#66788=CARTESIAN_POINT('Ctrl Pts',(-2.40149358463894,5.32459596941663,82.9951136462743));
#66789=CARTESIAN_POINT('Ctrl Pts',(-5.7758875400995,0.870412109585264,83.1538744085203));
#66790=CARTESIAN_POINT('Ctrl Pts',(-3.86401262590961,-4.3803993931662,83.3126351707661));
#66791=CARTESIAN_POINT('Ctrl Pts',(1.58432435304567,-5.62213577491609,83.4713959330121));
#66792=CARTESIAN_POINT('Ctrl Pts',(5.58263989986849,-1.71832137308609,83.6301566952579));
#66793=CARTESIAN_POINT('Ctrl Pts',(4.47155171880276,3.75815248538495,83.7889174575037));
#66794=CARTESIAN_POINT('Ctrl Pts',(-0.732034944345687,5.79505183303421,
83.9476782197497));
#66795=CARTESIAN_POINT('Ctrl Pts',(-5.26564514937354,2.52813997655405,84.1064389819955));
#66796=CARTESIAN_POINT('Ctrl Pts',(-4.97996786863125,-3.05259753396621,
84.2651997442416));
#66797=CARTESIAN_POINT('Ctrl Pts',(-0.136487592502867,-5.83951464301881,
84.4239605064873));
#66798=CARTESIAN_POINT('Ctrl Pts',(4.83194039314673,-3.28191022714265,84.5827212687333));
#66799=CARTESIAN_POINT('Ctrl Pts',(5.3779712939643,2.27936160776507,84.7414820309791));
#66800=CARTESIAN_POINT('Ctrl Pts',(1.00202900079473,5.75456307304708,84.9002427932251));
#66801=CARTESIAN_POINT('Ctrl Pts',(-4.29121230689459,3.96287665367137,85.059003555471));
#66802=CARTESIAN_POINT('Ctrl Pts',(-5.65660000441566,-1.45549506770408,
85.2177643177168));
#66803=CARTESIAN_POINT('Ctrl Pts',(-1.84567038925739,-5.54225213649743,
85.3765250799627));
#66804=CARTESIAN_POINT('Ctrl Pts',(3.65595928985271,-4.55561497937659,85.5352858422086));
#66805=CARTESIAN_POINT('Ctrl Pts',(5.8086947012646,0.598627392648328,85.6940466044544));
#66806=CARTESIAN_POINT('Ctrl Pts',(2.65061116100751,5.20851728785982,85.8528073667005));
#66807=CARTESIAN_POINT('Ctrl Pts',(-2.94405900471206,5.04447882807405,86.0115681289463));
#66808=CARTESIAN_POINT('Ctrl Pts',(-5.34253328840157,1.07278402652743,86.1438687641512));
#66809=CARTESIAN_POINT('Ctrl Pts',(-4.62260421807956,-2.25450493511227,
86.2497092723151));
#66810=CARTESIAN_POINT('Ctrl Pts',(-3.53826020855044,-3.54670961616112,
86.3026295263971));
#66811=CARTESIAN_POINT('Ctrl Pts',(-2.86929757049814,-4.02374147429149,
86.3290896534381));
#66812=CARTESIAN_POINT('',(-2.16917135428524,4.44050218283342,86.));
#66813=CARTESIAN_POINT('Ctrl Pts',(-2.17574227734826,4.44486702454923,86.));
#66814=CARTESIAN_POINT('Ctrl Pts',(-2.28013295862628,4.38716599510334,86.));
#66815=CARTESIAN_POINT('Ctrl Pts',(-2.38203491056673,4.32558764363711,86.));
#66816=CARTESIAN_POINT('Ctrl Pts',(-2.48120820121107,4.26013722079047,86.));
#66817=CARTESIAN_POINT('Ctrl Pts',(-2.60006688906204,4.18169521963978,86.));
#66818=CARTESIAN_POINT('Ctrl Pts',(-2.7150074127347,4.09769239705542,86.));
#66819=CARTESIAN_POINT('Ctrl Pts',(-2.825877147636,4.00855468944723,86.));
#66820=CARTESIAN_POINT('Ctrl Pts',(-2.93875239431318,3.9178045785764,86.));
#66821=CARTESIAN_POINT('Ctrl Pts',(-3.04740870522866,3.82173148785291,86.));
#66822=CARTESIAN_POINT('Ctrl Pts',(-3.15164741290182,3.72074618418362,86.));
#66823=CARTESIAN_POINT('Ctrl Pts',(-3.25648521909179,3.61918048051708,86.));
#66824=CARTESIAN_POINT('Ctrl Pts',(-3.35685490813916,3.51264518527105,86.));
#66825=CARTESIAN_POINT('Ctrl Pts',(-3.45251018852357,3.40153010769327,86.));
#66826=CARTESIAN_POINT('Ctrl Pts',(-3.48145067837577,3.36791225866138,86.));
#66827=CARTESIAN_POINT('Ctrl Pts',(-3.50995929996644,3.33387504208837,86.));
#66828=CARTESIAN_POINT('Ctrl Pts',(-3.53802835306874,3.2994289123823,86.));
#66829=CARTESIAN_POINT('Ctrl Pts',(-3.55893895860226,3.27376757539972,86.));
#66830=CARTESIAN_POINT('Ctrl Pts',(-3.57960560368256,3.24787929661303,86.));
#66831=CARTESIAN_POINT('Ctrl Pts',(-3.60002494885949,3.22176835839145,86.));
#66832=CARTESIAN_POINT('Ctrl Pts',(-3.61193639941707,3.20653676565705,86.));
#66833=CARTESIAN_POINT('Ctrl Pts',(-3.62375830311465,3.19123627397227,86.));
#66834=CARTESIAN_POINT('Ctrl Pts',(-3.63548790188773,3.17587102356872,86.));
#66835=CARTESIAN_POINT('Ctrl Pts',(-3.72304104356389,3.06118031918079,86.));
#66836=CARTESIAN_POINT('Ctrl Pts',(-3.80549810494951,2.94282892853622,86.));
#66837=CARTESIAN_POINT('Ctrl Pts',(-3.88269282098784,2.82123575460696,86.));
#66838=CARTESIAN_POINT('Ctrl Pts',(-3.96010237178875,2.69930418393253,86.));
#66839=CARTESIAN_POINT('Ctrl Pts',(-4.03222060518193,2.57411198603205,86.));
#66840=CARTESIAN_POINT('Ctrl Pts',(-4.09883515477919,2.44605409339683,86.));
#66841=CARTESIAN_POINT('Ctrl Pts',(-4.16485320331115,2.31914289723916,86.));
#66842=CARTESIAN_POINT('Ctrl Pts',(-4.2254659552961,2.18941632853557,86.));
#66843=CARTESIAN_POINT('Ctrl Pts',(-4.28041834739517,2.05724343991072,86.));
#66844=CARTESIAN_POINT('Ctrl Pts',(-4.33438117280193,1.92745068221766,86.));
#66845=CARTESIAN_POINT('Ctrl Pts',(-4.38288583069982,1.79529822126205,86.));
#66846=CARTESIAN_POINT('Ctrl Pts',(-4.42564090526442,1.66113144401598,86.));
#66847=CARTESIAN_POINT('Ctrl Pts',(-4.43255967958786,1.63942011119941,86.));
#66848=CARTESIAN_POINT('Ctrl Pts',(-4.43932777954855,1.61765603376178,86.));
#66849=CARTESIAN_POINT('Ctrl Pts',(-4.4459438397712,1.59584068384471,86.));
#66850=CARTESIAN_POINT('Ctrl Pts',(-4.45171251084707,1.57681945764039,86.));
#66851=CARTESIAN_POINT('Ctrl Pts',(-4.45736585345657,1.55775815091916,86.));
#66852=CARTESIAN_POINT('Ctrl Pts',(-4.46289825998277,1.53867450299572,86.));
#66853=CARTESIAN_POINT('Ctrl Pts',(-4.50224730205451,1.40294274476988,86.));
#66854=CARTESIAN_POINT('Ctrl Pts',(-4.53554254717084,1.2658880814313,86.));
#66855=CARTESIAN_POINT('Ctrl Pts',(-4.56258502829437,1.12787819891714,86.));
#66856=CARTESIAN_POINT('Ctrl Pts',(-4.58931759393923,0.991449953775849,
86.));
#66857=CARTESIAN_POINT('Ctrl Pts',(-4.60994008626122,0.854087541637941,
86.));
#66858=CARTESIAN_POINT('Ctrl Pts',(-4.62421031200347,0.716138535076822,
86.));
#66859=CARTESIAN_POINT('Ctrl Pts',(-4.63813932416541,0.581488009932714,
86.));
#66860=CARTESIAN_POINT('Ctrl Pts',(-4.64601628194546,0.446277995360083,
86.));
#66861=CARTESIAN_POINT('Ctrl Pts',(-4.64756630557454,0.310834136529796,
86.));
#66862=CARTESIAN_POINT('Ctrl Pts',(-4.64793240287716,0.278843894287929,
86.));
#66863=CARTESIAN_POINT('Ctrl Pts',(-4.6479453277195,0.246840640295154,86.));
#66864=CARTESIAN_POINT('Ctrl Pts',(-4.64760103388387,0.214828741346587,
86.));
#66865=CARTESIAN_POINT('Ctrl Pts',(-4.64657805635091,0.119713900408526,
86.));
#66866=CARTESIAN_POINT('Ctrl Pts',(-4.64240219271064,0.0245223992060761,
86.));
#66867=CARTESIAN_POINT('Ctrl Pts',(-4.63512171526216,-0.0706009649893001,
86.));
#66868=CARTESIAN_POINT('Ctrl Pts',(-4.63272301775774,-0.101941241491998,
86.));
#66869=CARTESIAN_POINT('Ctrl Pts',(-4.62998723239254,-0.133274083991166,
86.));
#66870=CARTESIAN_POINT('Ctrl Pts',(-4.62691585213729,-0.16459419159554,
86.));
#66871=CARTESIAN_POINT('Ctrl Pts',(-4.62511596030474,-0.182948417118559,
86.));
#66872=CARTESIAN_POINT('Ctrl Pts',(-4.62320081633973,-0.201298267969776,
86.));
#66873=CARTESIAN_POINT('Ctrl Pts',(-4.62117070299388,-0.21964266601306,
86.));
#66874=CARTESIAN_POINT('Ctrl Pts',(-4.61910605502354,-0.238299123921961,
86.));
#66875=CARTESIAN_POINT('Ctrl Pts',(-4.6169235721841,-0.256940116225532,
86.));
#66876=CARTESIAN_POINT('Ctrl Pts',(-4.61462417515337,-0.275562596752177,
86.));
#66877=CARTESIAN_POINT('Ctrl Pts',(-4.59791089402231,-0.410921018216574,
86.));
#66878=CARTESIAN_POINT('Ctrl Pts',(-4.57502130177171,-0.545336418557933,
86.));
#66879=CARTESIAN_POINT('Ctrl Pts',(-4.54619383694625,-0.678403869974182,
86.));
#66880=CARTESIAN_POINT('Ctrl Pts',(-4.51690235263596,-0.81361323330078,
86.));
#66881=CARTESIAN_POINT('Ctrl Pts',(-4.48148002405017,-0.947431726142265,
86.));
#66882=CARTESIAN_POINT('Ctrl Pts',(-4.44012512005541,-1.07942238906511,
86.));
#66883=CARTESIAN_POINT('Ctrl Pts',(-4.39891579514076,-1.21094841351862,
86.));
#66884=CARTESIAN_POINT('Ctrl Pts',(-4.35181516564808,-1.34066022876501,
86.));
#66885=CARTESIAN_POINT('Ctrl Pts',(-4.29897383984103,-1.46810153698611,
86.));
#66886=CARTESIAN_POINT('Ctrl Pts',(-4.26316764637209,-1.55445796480857,
86.));
#66887=CARTESIAN_POINT('Ctrl Pts',(-4.22472458946287,-1.639771352916,86.));
#66888=CARTESIAN_POINT('Ctrl Pts',(-4.18368102987994,-1.72389071907676,
86.));
#66889=CARTESIAN_POINT('Ctrl Pts',(-4.16189573536735,-1.76853999376555,
86.));
#66890=CARTESIAN_POINT('Ctrl Pts',(-4.13937765883534,-1.81285273679093,
86.));
#66891=CARTESIAN_POINT('Ctrl Pts',(-4.11613135978827,-1.85680534418916,
86.));
#66892=CARTESIAN_POINT('Ctrl Pts',(-4.10598652796122,-1.87598653985015,
86.));
#66893=CARTESIAN_POINT('Ctrl Pts',(-4.09570182816448,-1.8951012704791,86.));
#66894=CARTESIAN_POINT('Ctrl Pts',(-4.08528136703263,-1.91414066944428,
86.));
#66895=CARTESIAN_POINT('Ctrl Pts',(-4.07459370444932,-1.93366827665418,
86.));
#66896=CARTESIAN_POINT('Ctrl Pts',(-4.06376686324371,-1.95311008122927,
86.));
#66897=CARTESIAN_POINT('Ctrl Pts',(-4.05280165642382,-1.97246424292779,
86.));
#66898=CARTESIAN_POINT('Ctrl Pts',(-3.98545341209713,-2.09133740530588,
86.));
#66899=CARTESIAN_POINT('Ctrl Pts',(-3.91288886269624,-2.20690686036164,
86.));
#66900=CARTESIAN_POINT('Ctrl Pts',(-3.83535609314517,-2.31888838615919,
86.));
#66901=CARTESIAN_POINT('Ctrl Pts',(-3.75793727989042,-2.43070532348649,
86.));
#66902=CARTESIAN_POINT('Ctrl Pts',(-3.67556431499777,-2.53894540267671,
86.));
#66903=CARTESIAN_POINT('Ctrl Pts',(-3.58844692437017,-2.6432897533722,86.));
#66904=CARTESIAN_POINT('Ctrl Pts',(-3.55106838804729,-2.68805967903758,
86.));
#66905=CARTESIAN_POINT('Ctrl Pts',(-3.51281602034817,-2.7321119355856,86.));
#66906=CARTESIAN_POINT('Ctrl Pts',(-3.47370464217661,-2.77541893263456,
86.));
#66907=CARTESIAN_POINT('Ctrl Pts',(-3.45527487716358,-2.79582572514213,
86.));
#66908=CARTESIAN_POINT('Ctrl Pts',(-3.43665436275494,-2.81606701722102,
86.));
#66909=CARTESIAN_POINT('Ctrl Pts',(-3.41784457942235,-2.83613979970913,
86.));
#66910=CARTESIAN_POINT('Ctrl Pts',(-3.40161580152966,-2.85345827291681,
86.));
#66911=CARTESIAN_POINT('Ctrl Pts',(-3.38525177230088,-2.87064524159307,
86.));
#66912=CARTESIAN_POINT('Ctrl Pts',(-3.36875789576418,-2.88769480011766,
86.));
#66913=CARTESIAN_POINT('Ctrl Pts',(-3.27548691461708,-2.98410809920928,
86.));
#66914=CARTESIAN_POINT('Ctrl Pts',(-3.1780247285723,-3.07617507300169,86.));
#66915=CARTESIAN_POINT('Ctrl Pts',(-3.07658549505738,-3.16359906081916,
86.));
#66916=CARTESIAN_POINT('Ctrl Pts',(-2.97674507744291,-3.24964513146433,
86.));
#66917=CARTESIAN_POINT('Ctrl Pts',(-2.87305144560376,-3.33119379608769,
86.));
#66918=CARTESIAN_POINT('Ctrl Pts',(-2.76568166074672,-3.40792026882373,
86.));
#66919=CARTESIAN_POINT('Ctrl Pts',(-2.691638695275,-3.46083138882947,86.));
#66920=CARTESIAN_POINT('Ctrl Pts',(-2.61584694697416,-3.51144841450292,
86.));
#66921=CARTESIAN_POINT('Ctrl Pts',(-2.53835875722777,-3.5596515025498,86.));
#66922=CARTESIAN_POINT('Ctrl Pts',(-4.94096920053978,-0.0044629540342261,
85.1776795453431));
#66923=CARTESIAN_POINT('Ctrl Pts',(-4.94470425404279,-0.419442432737937,
85.1910411361343));
#66924=CARTESIAN_POINT('Ctrl Pts',(-4.89679105157154,-0.83357493998294,
85.2044027269256));
#66925=CARTESIAN_POINT('Ctrl Pts',(-4.79388045230233,-1.23355929227409,
85.2177643177168));
#66926=CARTESIAN_POINT('Ctrl Pts',(-4.38629013269605,-2.81774742396872,
85.2706845717988));
#66927=CARTESIAN_POINT('Ctrl Pts',(-3.11598026097668,-4.17999978023304,
85.3236048258808));
#66928=CARTESIAN_POINT('Ctrl Pts',(-1.5638870452654,-4.69668643217841,85.3765250799627));
#66929=CARTESIAN_POINT('Ctrl Pts',(-0.0117938295540432,-5.21337308412381,
85.4294453340447));
#66930=CARTESIAN_POINT('Ctrl Pts',(1.82208273014937,-4.88449403175019,85.4823655881266));
#66931=CARTESIAN_POINT('Ctrl Pts',(3.09781024523634,-3.86101411022591,85.5352858422086));
#66932=CARTESIAN_POINT('Ctrl Pts',(4.37353776032332,-2.83753418870164,85.5882060962905));
#66933=CARTESIAN_POINT('Ctrl Pts',(5.0911162307939,-1.11945339802691,85.6411263503725));
#66934=CARTESIAN_POINT('Ctrl Pts',(4.92355820931981,0.507901979845797,85.6940466044544));
#66935=CARTESIAN_POINT('Ctrl Pts',(4.75600018784572,2.1352573577185,85.7469668585364));
#66936=CARTESIAN_POINT('Ctrl Pts',(3.70330567442676,3.67188732278906,85.7998871126184));
#66937=CARTESIAN_POINT('Ctrl Pts',(2.24451339009742,4.41286256202677,85.8528073667004));
#66938=CARTESIAN_POINT('Ctrl Pts',(0.892016244518137,5.09984651908455,85.9018715778003));
#66939=CARTESIAN_POINT('Ctrl Pts',(-0.809554018707134,5.10290237899098,
85.9509357889001));
#66940=CARTESIAN_POINT('Ctrl Pts',(-2.17574227734751,4.44486702454959,86.));
#66941=CARTESIAN_POINT('',(-2.53835875722709,-3.55965150255029,26.));
#66942=CARTESIAN_POINT('Ctrl Pts',(-2.54472725763298,-3.56250530678305,
26.));
#66943=CARTESIAN_POINT('Ctrl Pts',(-2.63508309937759,-3.50703322951937,
26.));
#66944=CARTESIAN_POINT('Ctrl Pts',(-2.72311007746572,-3.44818980724315,
26.));
#66945=CARTESIAN_POINT('Ctrl Pts',(-2.80858488092082,-3.38601400346164,
26.));
#66946=CARTESIAN_POINT('Ctrl Pts',(-2.91385291450225,-3.30944027253914,
26.));
#66947=CARTESIAN_POINT('Ctrl Pts',(-3.01525129898596,-3.22781364096124,
26.));
#66948=CARTESIAN_POINT('Ctrl Pts',(-3.11268784287649,-3.1415518359691,26.));
#66949=CARTESIAN_POINT('Ctrl Pts',(-3.17680627098234,-3.08478698039414,
26.));
#66950=CARTESIAN_POINT('Ctrl Pts',(-3.23920859831056,-3.02601391139215,
26.));
#66951=CARTESIAN_POINT('Ctrl Pts',(-3.29986195943645,-2.96534150637499,
26.));
#66952=CARTESIAN_POINT('Ctrl Pts',(-3.33570437568566,-2.9294878363541,26.));
#66953=CARTESIAN_POINT('Ctrl Pts',(-3.37093593415121,-2.89297075792499,
26.));
#66954=CARTESIAN_POINT('Ctrl Pts',(-3.40554888779674,-2.85581160143786,
26.));
#66955=CARTESIAN_POINT('Ctrl Pts',(-3.4189115430604,-2.84146596069563,26.));
#66956=CARTESIAN_POINT('Ctrl Pts',(-3.43218080021828,-2.82702583304496,
26.));
#66957=CARTESIAN_POINT('Ctrl Pts',(-3.44534999888201,-2.81249952818835,
26.));
#66958=CARTESIAN_POINT('Ctrl Pts',(-3.53470458244056,-2.71393681725578,
26.));
#66959=CARTESIAN_POINT('Ctrl Pts',(-3.61953742655147,-2.6113223183339,26.));
#66960=CARTESIAN_POINT('Ctrl Pts',(-3.69975229053408,-2.50508736800556,
26.));
#66961=CARTESIAN_POINT('Ctrl Pts',(-3.78158309623279,-2.39671229701354,
26.));
#66962=CARTESIAN_POINT('Ctrl Pts',(-3.85860846570253,-2.28456889207013,
26.));
#66963=CARTESIAN_POINT('Ctrl Pts',(-3.93069241652625,-2.16907329602735,
26.));
#66964=CARTESIAN_POINT('Ctrl Pts',(-3.96222914501164,-2.11854397275863,
26.));
#66965=CARTESIAN_POINT('Ctrl Pts',(-3.99281958123178,-2.06737253695488,
26.));
#66966=CARTESIAN_POINT('Ctrl Pts',(-4.02244999738294,-2.01559181929177,
26.));
#66967=CARTESIAN_POINT('Ctrl Pts',(-4.03719360535128,-1.98982658543039,
26.));
#66968=CARTESIAN_POINT('Ctrl Pts',(-4.05169949925962,-1.96391048284628,
26.));
#66969=CARTESIAN_POINT('Ctrl Pts',(-4.06596584566683,-1.93784746217908,
26.));
#66970=CARTESIAN_POINT('Ctrl Pts',(-4.07831325232761,-1.91529012999318,
26.));
#66971=CARTESIAN_POINT('Ctrl Pts',(-4.09048280358417,-1.89261955019595,
26.));
#66972=CARTESIAN_POINT('Ctrl Pts',(-4.10246124623198,-1.86986160408455,
26.));
#66973=CARTESIAN_POINT('Ctrl Pts',(-4.16682782765767,-1.74757098296373,
26.));
#66974=CARTESIAN_POINT('Ctrl Pts',(-4.22575033277333,-1.62263418183686,
26.));
#66975=CARTESIAN_POINT('Ctrl Pts',(-4.27912376767658,-1.49549834075104,
26.));
#66976=CARTESIAN_POINT('Ctrl Pts',(-4.333101839857,-1.36692225005554,26.));
#66977=CARTESIAN_POINT('Ctrl Pts',(-4.38140486252481,-1.23609633060621,
26.));
#66978=CARTESIAN_POINT('Ctrl Pts',(-4.42388482122499,-1.10344716235086,
26.));
#66979=CARTESIAN_POINT('Ctrl Pts',(-4.46661826556875,-0.970006452370537,
26.));
#66980=CARTESIAN_POINT('Ctrl Pts',(-4.50345940350737,-0.83471991605117,
26.));
#66981=CARTESIAN_POINT('Ctrl Pts',(-4.53421101307421,-0.697996575960625,
26.));
#66982=CARTESIAN_POINT('Ctrl Pts',(-4.55727472024934,-0.595454070892716,
26.));
#66983=CARTESIAN_POINT('Ctrl Pts',(-4.57691215392772,-0.492102769524819,
26.));
#66984=CARTESIAN_POINT('Ctrl Pts',(-4.59302069983613,-0.388109915197262,
26.));
#66985=CARTESIAN_POINT('Ctrl Pts',(-4.59983051322201,-0.344147416318648,
26.));
#66986=CARTESIAN_POINT('Ctrl Pts',(-4.60600945165704,-0.300070227388598,
26.));
#66987=CARTESIAN_POINT('Ctrl Pts',(-4.61154878947915,-0.25589088056297,
26.));
#66988=CARTESIAN_POINT('Ctrl Pts',(-4.6146089290101,-0.231484539947162,
26.));
#66989=CARTESIAN_POINT('Ctrl Pts',(-4.61747426508659,-0.207042538674214,
26.));
#66990=CARTESIAN_POINT('Ctrl Pts',(-4.62014035545176,-0.182595807090288,
26.));
#66991=CARTESIAN_POINT('Ctrl Pts',(-4.6355064624287,-0.0416961970611351,
26.));
#66992=CARTESIAN_POINT('Ctrl Pts',(-4.64428121342256,0.099526957690747,
26.));
#66993=CARTESIAN_POINT('Ctrl Pts',(-4.64631642071577,0.240645210364403,
26.));
#66994=CARTESIAN_POINT('Ctrl Pts',(-4.64782495501833,0.345244739654039,
26.));
#66995=CARTESIAN_POINT('Ctrl Pts',(-4.64562987589745,0.449787288147385,
26.));
#66996=CARTESIAN_POINT('Ctrl Pts',(-4.6396534459514,0.554104703798643,26.));
#66997=CARTESIAN_POINT('Ctrl Pts',(-4.63179775743763,0.691224210145253,
26.));
#66998=CARTESIAN_POINT('Ctrl Pts',(-4.61741097334291,0.827954978565883,
26.));
#66999=CARTESIAN_POINT('Ctrl Pts',(-4.59676076751363,0.963919018344825,
26.));
#67000=CARTESIAN_POINT('Ctrl Pts',(-4.57581741441672,1.1018131835223,26.));
#67001=CARTESIAN_POINT('Ctrl Pts',(-4.54843137134414,1.23891944459888,26.));
#67002=CARTESIAN_POINT('Ctrl Pts',(-4.51482841662203,1.3748401921847,26.));
#67003=CARTESIAN_POINT('Ctrl Pts',(-4.50509310232456,1.41421861019102,26.));
#67004=CARTESIAN_POINT('Ctrl Pts',(-4.49483564045414,1.45349746044631,26.));
#67005=CARTESIAN_POINT('Ctrl Pts',(-4.48406073341117,1.49266688179373,26.));
#67006=CARTESIAN_POINT('Ctrl Pts',(-4.47783668509381,1.51529281908091,26.));
#67007=CARTESIAN_POINT('Ctrl Pts',(-4.47143997379187,1.53788224103568,26.));
#67008=CARTESIAN_POINT('Ctrl Pts',(-4.46487145429867,1.56043322804307,26.));
#67009=CARTESIAN_POINT('Ctrl Pts',(-4.45973334069111,1.57807335734872,26.));
#67010=CARTESIAN_POINT('Ctrl Pts',(-4.45449021537901,1.59568938184522,26.));
#67011=CARTESIAN_POINT('Ctrl Pts',(-4.44914654369818,1.61326759097873,26.));
#67012=CARTESIAN_POINT('Ctrl Pts',(-4.40827604464057,1.7477126360219,26.));
#67013=CARTESIAN_POINT('Ctrl Pts',(-4.36147201478811,1.88014056905998,26.));
#67014=CARTESIAN_POINT('Ctrl Pts',(-4.30904356529584,2.01016709268461,26.));
#67015=CARTESIAN_POINT('Ctrl Pts',(-4.25484746504965,2.14457752399178,26.));
#67016=CARTESIAN_POINT('Ctrl Pts',(-4.19464124103037,2.27642270082558,26.));
#67017=CARTESIAN_POINT('Ctrl Pts',(-4.12870910753944,2.4052752225727,26.));
#67018=CARTESIAN_POINT('Ctrl Pts',(-4.06277697404851,2.53412774431982,26.));
#67019=CARTESIAN_POINT('Ctrl Pts',(-3.991118562445,2.65998845878048,26.));
#67020=CARTESIAN_POINT('Ctrl Pts',(-3.91396546539836,2.78241449550764,26.));
#67021=CARTESIAN_POINT('Ctrl Pts',(-3.8599022254897,2.86820169586649,26.));
#67022=CARTESIAN_POINT('Ctrl Pts',(-3.80313988532888,2.95230207537908,26.));
#67023=CARTESIAN_POINT('Ctrl Pts',(-3.74376497539126,3.03461721426763,26.));
#67024=CARTESIAN_POINT('Ctrl Pts',(-3.71778845229355,3.07063008753137,26.));
#67025=CARTESIAN_POINT('Ctrl Pts',(-3.69131172751679,3.10630115823714,26.));
#67026=CARTESIAN_POINT('Ctrl Pts',(-3.66434142116742,3.1416216999591,26.));
#67027=CARTESIAN_POINT('Ctrl Pts',(-3.64886736739569,3.16188665189447,26.));
#67028=CARTESIAN_POINT('Ctrl Pts',(-3.63323082853231,3.18203621015477,26.));
#67029=CARTESIAN_POINT('Ctrl Pts',(-3.61743300165625,3.20206867796743,26.));
#67030=CARTESIAN_POINT('Ctrl Pts',(-3.60562290128194,3.21704450074792,26.));
#67031=CARTESIAN_POINT('Ctrl Pts',(-3.59372248215876,3.23195501636103,26.));
#67032=CARTESIAN_POINT('Ctrl Pts',(-3.58174179779154,3.24678792441536,26.));
#67033=CARTESIAN_POINT('Ctrl Pts',(-3.49102566491969,3.35910071195637,26.));
#67034=CARTESIAN_POINT('Ctrl Pts',(-3.39558140635013,3.46713215575717,26.));
#67035=CARTESIAN_POINT('Ctrl Pts',(-3.29573453983928,3.57065014592309,26.));
#67036=CARTESIAN_POINT('Ctrl Pts',(-3.19481521819522,3.67528002275919,26.));
#67037=CARTESIAN_POINT('Ctrl Pts',(-3.08939783097439,3.77529957447928,26.));
#67038=CARTESIAN_POINT('Ctrl Pts',(-2.97977151694561,3.87044492257043,26.));
#67039=CARTESIAN_POINT('Ctrl Pts',(-2.87044051512184,3.9653339673936,26.));
#67040=CARTESIAN_POINT('Ctrl Pts',(-2.75692276267532,4.05537559850027,26.));
#67041=CARTESIAN_POINT('Ctrl Pts',(-2.63946507568592,4.14027538885812,26.));
#67042=CARTESIAN_POINT('Ctrl Pts',(-2.52377549108901,4.22389717412067,26.));
#67043=CARTESIAN_POINT('Ctrl Pts',(-2.40426319127569,4.30253122094905,26.));
#67044=CARTESIAN_POINT('Ctrl Pts',(-2.28113248745318,4.37585694114117,26.));
#67045=CARTESIAN_POINT('Ctrl Pts',(-2.24413725288456,4.39788801977718,26.));
#67046=CARTESIAN_POINT('Ctrl Pts',(-2.20681518281834,4.41943960051781,26.));
#67047=CARTESIAN_POINT('Ctrl Pts',(-2.16917135428626,4.44050218283292,26.));
#67048=CARTESIAN_POINT('Ctrl Pts',(-2.54472725763282,-3.56250530678316,
26.));
#67049=CARTESIAN_POINT('Ctrl Pts',(-1.44818804155806,-4.33531677513798,
26.0490642110999));
#67050=CARTESIAN_POINT('Ctrl Pts',(1.63914523023693,-4.84388073813931,26.1510486762817));
#67051=CARTESIAN_POINT('Ctrl Pts',(4.98187809541805,-1.36671674862893,26.3059533955455));
#67052=CARTESIAN_POINT('Ctrl Pts',(3.85252000415521,3.44398917781397,26.4647141577913));
#67053=CARTESIAN_POINT('Ctrl Pts',(-0.805001512196143,5.10466442465425,
26.6234749200372));
#67054=CARTESIAN_POINT('Ctrl Pts',(-3.96413630374849,2.67678406505067,26.7514334980751));
#67055=CARTESIAN_POINT('Ctrl Pts',(-4.3679444184666,0.611489669763926,26.826471822031));
#67056=CARTESIAN_POINT('Ctrl Pts',(-4.36558297706963,0.00185075076461511,
26.848589891905));
#67057=CARTESIAN_POINT('Origin',(0.,0.,24.1514101080949));
#67058=CARTESIAN_POINT('',(2.5383587572269,-3.55965150255042,26.));
#67059=CARTESIAN_POINT('Origin',(0.,0.,26.));
#67060=CARTESIAN_POINT('Ctrl Pts',(2.53835875722654,-3.55965150255068,26.));
#67061=CARTESIAN_POINT('Ctrl Pts',(3.13016463613492,-3.13763950664917,26.026460127041));
#67062=CARTESIAN_POINT('Ctrl Pts',(4.08944058768451,-1.99447514282845,26.079380381123));
#67063=CARTESIAN_POINT('Ctrl Pts',(4.72633908941221,0.949051473338421,26.1852208892869));
#67064=CARTESIAN_POINT('Ctrl Pts',(2.60449620246589,4.46265906441401,26.3175215244918));
#67065=CARTESIAN_POINT('Ctrl Pts',(-2.34489469821123,4.60777770546463,26.4762822867377));
#67066=CARTESIAN_POINT('Ctrl Pts',(-4.30346090622908,1.74883727013167,26.5875784812721));
#67067=CARTESIAN_POINT('Ctrl Pts',(-4.3779262327693,0.151632086931482,26.6459544217245));
#67068=CARTESIAN_POINT('Ctrl Pts',(-4.37688026104952,0.00226901643694839,
26.651410108095));
#67069=CARTESIAN_POINT('Ctrl Pts',(2.86929757049756,-4.02374147429191,25.6709103465619));
#67070=CARTESIAN_POINT('Ctrl Pts',(3.53826020854994,-3.54670961616163,25.6973704736029));
#67071=CARTESIAN_POINT('Ctrl Pts',(4.62260187198943,-2.25450506767067,25.7502907276849));
#67072=CARTESIAN_POINT('Ctrl Pts',(5.34253608871791,1.0727841677129,25.8561312358488));
#67073=CARTESIAN_POINT('Ctrl Pts',(2.94405769272283,5.04447875030544,25.9884318710537));
#67074=CARTESIAN_POINT('Ctrl Pts',(-2.65061061266289,5.20851725077882,26.1471926332996));
#67075=CARTESIAN_POINT('Ctrl Pts',(-5.80869481541901,0.598627327994403,
26.3059533955455));
#67076=CARTESIAN_POINT('Ctrl Pts',(-3.6559591721986,-4.55561486272761,26.4647141577913));
#67077=CARTESIAN_POINT('Ctrl Pts',(1.84567034813922,-5.54225209737284,26.6234749200373));
#67078=CARTESIAN_POINT('Ctrl Pts',(5.65659992177503,-1.45549501989441,26.7822356822831));
#67079=CARTESIAN_POINT('Ctrl Pts',(4.29121225256454,3.96287657984353,26.940996444529));
#67080=CARTESIAN_POINT('Ctrl Pts',(-1.00202899277672,5.75456300236789,27.0997572067749));
#67081=CARTESIAN_POINT('Ctrl Pts',(-5.37797121296738,2.27936156876184,27.2585179690208));
#67082=CARTESIAN_POINT('Ctrl Pts',(-4.83194032779028,-3.28191017660925,
27.4172787312667));
#67083=CARTESIAN_POINT('Ctrl Pts',(0.136487592633803,-5.83951456248522,
27.5760394935126));
#67084=CARTESIAN_POINT('Ctrl Pts',(4.97996779668276,-3.05259748930662,27.7348002557585));
#67085=CARTESIAN_POINT('Ctrl Pts',(5.26564507543792,2.52813993990873,27.8935610180044));
#67086=CARTESIAN_POINT('Ctrl Pts',(0.732034933496452,5.79505175124635,28.0523217802503));
#67087=CARTESIAN_POINT('Ctrl Pts',(-4.47155165508331,3.75815243181214,28.2110825424962));
#67088=CARTESIAN_POINT('Ctrl Pts',(-5.58263982081247,-1.71832134856424,
28.369843304742));
#67089=CARTESIAN_POINT('Ctrl Pts',(-1.58432433047622,-5.62213569522022,
28.5286040669879));
#67090=CARTESIAN_POINT('Ctrl Pts',(3.86401257103054,-4.38039933096899,28.6873648292338));
#67091=CARTESIAN_POINT('Ctrl Pts',(5.77588745817332,0.870412097209825,28.8461255914797));
#67092=CARTESIAN_POINT('Ctrl Pts',(2.40149355054825,5.32459589387785,29.0048863537256));
#67093=CARTESIAN_POINT('Ctrl Pts',(-3.17082052230127,4.90554683073371,29.1636471159715));
#67094=CARTESIAN_POINT('Ctrl Pts',(-5.84110284449404,-0.00320850462351047,
29.3224078782174));
#67095=CARTESIAN_POINT('Ctrl Pts',(-3.16542940092975,-4.90902733376601,
29.4811686404633));
#67096=CARTESIAN_POINT('Ctrl Pts',(2.40734170730851,-5.32195439090584,29.6399294027091));
#67097=CARTESIAN_POINT('Ctrl Pts',(5.77684015826,-0.8640662324248,29.7986901649551));
#67098=CARTESIAN_POINT('Ctrl Pts',(3.85919803712304,4.38464173738479,29.9574509272009));
#67099=CARTESIAN_POINT('Ctrl Pts',(-1.59050000656898,5.62039165738282,30.1162116894468));
#67100=CARTESIAN_POINT('Ctrl Pts',(-5.58452386271215,1.71218745603623,30.2749724516927));
#67101=CARTESIAN_POINT('Ctrl Pts',(-4.46742089771919,-3.76306300482994,
30.4337332139386));
#67102=CARTESIAN_POINT('Ctrl Pts',(0.738402131764131,-5.79424325925859,
30.5924939761845));
#67103=CARTESIAN_POINT('Ctrl Pts',(5.26841697560084,-2.522355095433,30.7512547384304));
#67104=CARTESIAN_POINT('Ctrl Pts',(4.97661567740753,3.05806949811635,30.9100155006762));
#67105=CARTESIAN_POINT('Ctrl Pts',(0.130063698581311,5.83965547701761,31.0687762629222));
#67106=CARTESIAN_POINT('Ctrl Pts',(-4.83552655005252,3.27661038876524,31.227537025168));
#67107=CARTESIAN_POINT('Ctrl Pts',(-5.37549519698693,-2.28528861265885,
31.386297787414));
#67108=CARTESIAN_POINT('Ctrl Pts',(-0.995646443005195,-5.75562167072471,
31.5450585496598));
#67109=CARTESIAN_POINT('Ctrl Pts',(4.2954483480341,-3.95823396799194,31.7038193119058));
#67110=CARTESIAN_POINT('Ctrl Pts',(5.65521760477304,1.46185036807875,31.8625800741516));
#67111=CARTESIAN_POINT('Ctrl Pts',(1.83915896875347,5.54400459448242,32.0213408363975));
#67112=CARTESIAN_POINT('Ctrl Pts',(-3.66015413331184,4.5521164721907,32.1801015986434));
#67113=CARTESIAN_POINT('Ctrl Pts',(-5.80958237170622,-0.606007691658192,
32.3388623608893));
#67114=CARTESIAN_POINT('Ctrl Pts',(-2.64190336751104,-5.20949510535547,
32.4976231231352));
#67115=CARTESIAN_POINT('Ctrl Pts',(2.9437262966194,-5.04509347253155,32.6563838853811));
#67116=CARTESIAN_POINT('Ctrl Pts',(5.83516773679323,-0.263268189260048,
32.8151446476269));
#67117=CARTESIAN_POINT('Ctrl Pts',(3.3860854267346,4.75950818245377,32.9739054098728));
#67118=CARTESIAN_POINT('Ctrl Pts',(-2.1620456951976,5.42623728451552,33.1326661721187));
#67119=CARTESIAN_POINT('Ctrl Pts',(-5.73140655633933,1.12670827721268,33.2914269343647));
#67120=CARTESIAN_POINT('Ctrl Pts',(-4.0552090690265,-4.20401856114767,33.4501876966105));
#67121=CARTESIAN_POINT('Ctrl Pts',(1.33243962623321,-5.68709919892666,33.6089484588564));
#67122=CARTESIAN_POINT('Ctrl Pts',(5.50059887566598,-1.96517293514109,33.7677092211022));
#67123=CARTESIAN_POINT('Ctrl Pts',(4.63444201610888,3.55533962587452,33.9264699833482));
#67124=CARTESIAN_POINT('Ctrl Pts',(-0.473297737465698,5.82189676202686,
34.0852307455941));
#67125=CARTESIAN_POINT('Ctrl Pts',(-5.14786094464401,2.7600761494201,34.24399150784));
#67126=CARTESIAN_POINT('Ctrl Pts',(-5.11094457182416,-2.82785046275963,
34.4027522700858));
#67127=CARTESIAN_POINT('Ctrl Pts',(-0.396335611036177,-5.82764195360469,
34.5615130323317));
#67128=CARTESIAN_POINT('Ctrl Pts',(4.68101180720102,-3.49379752086946,34.7202737945776));
#67129=CARTESIAN_POINT('Ctrl Pts',(5.47415423612042,2.03767712240033,34.8790345568235));
#67130=CARTESIAN_POINT('Ctrl Pts',(1.2571834979241,5.7042074215912,35.0377953190694));
#67131=CARTESIAN_POINT('Ctrl Pts',(-4.11039997874232,4.15007285125745,35.1965560813153));
#67132=CARTESIAN_POINT('Ctrl Pts',(-5.71601984106162,-1.20233515817297,
35.3553168435612));
#67133=CARTESIAN_POINT('Ctrl Pts',(-2.09016374674189,-5.45432930503785,
35.5140776058071));
#67134=CARTESIAN_POINT('Ctrl Pts',(3.44867405347895,-4.71435466727419,35.6728383680529));
#67135=CARTESIAN_POINT('Ctrl Pts',(5.8311800188353,0.340341363817132,35.8315991302989));
#67136=CARTESIAN_POINT('Ctrl Pts',(2.87681191524069,5.0835465828807,35.9903598925447));
#67137=CARTESIAN_POINT('Ctrl Pts',(-2.7105023265463,5.17413469033962,36.1491206547906));
#67138=CARTESIAN_POINT('Ctrl Pts',(-5.81708204570653,0.529196683197753,
36.3078814170365));
#67139=CARTESIAN_POINT('Ctrl Pts',(-3.5996905915515,-4.60007829292986,36.4666421792824));
#67140=CARTESIAN_POINT('Ctrl Pts',(1.91224764597227,-5.51922110414707,36.6254029415283));
#67141=CARTESIAN_POINT('Ctrl Pts',(5.67403842753732,-1.38700417404515,36.7841637037742));
#67142=CARTESIAN_POINT('Ctrl Pts',(4.24277592445978,4.01464134273703,36.9429244660201));
#67143=CARTESIAN_POINT('Ctrl Pts',(-1.07160470196143,5.74196447382976,37.1016852282659));
#67144=CARTESIAN_POINT('Ctrl Pts',(-5.40521997255572,2.2140663278849,37.2604459905119));
#67145=CARTESIAN_POINT('Ctrl Pts',(-4.79181281967314,-3.34021295087678,
37.4192067527577));
#67146=CARTESIAN_POINT('Ctrl Pts',(0.207207793602656,-5.83742730886296,
37.5779675150036));
#67147=CARTESIAN_POINT('Ctrl Pts',(5.01658550492884,-2.99204988723897,37.7367282772495));
#67148=CARTESIAN_POINT('Ctrl Pts',(5.23463092854471,2.59174298453994,37.8954890394954));
#67149=CARTESIAN_POINT('Ctrl Pts',(0.661782232472825,5.80349351104764,38.0542498017413));
#67150=CARTESIAN_POINT('Ctrl Pts',(-4.51674977715968,3.70370950622708,38.2130105639872));
#67151=CARTESIAN_POINT('Ctrl Pts',(-5.5614144248173,-1.78582256997244,38.371771326233));
#67152=CARTESIAN_POINT('Ctrl Pts',(-1.51610271526659,-5.64091528147253,
38.530532088479));
#67153=CARTESIAN_POINT('Ctrl Pts',(3.91679250925652,-4.33327002336813,38.6892928507249));
#67154=CARTESIAN_POINT('Ctrl Pts',(5.76491958932306,0.940316321579044,38.8480536129708));
#67155=CARTESIAN_POINT('Ctrl Pts',(2.33681616947948,5.35329644668107,39.0068143752167));
#67156=CARTESIAN_POINT('Ctrl Pts',(-3.23001278765103,4.86677614521149,39.1655751374625));
#67157=CARTESIAN_POINT('Ctrl Pts',(-5.84063537949807,-0.0739663419686063,
39.3243358997085));
#67158=CARTESIAN_POINT('Ctrl Pts',(-3.10573006749788,-4.94701257364771,
39.4830966619543));
#67159=CARTESIAN_POINT('Ctrl Pts',(2.47163426803653,-5.29240178945783,39.6418574242002));
#67160=CARTESIAN_POINT('Ctrl Pts',(5.78688342441216,-0.794023229038551,
39.8006181864461));
#67161=CARTESIAN_POINT('Ctrl Pts',(3.80580010810998,4.43106964435213,39.959378948692));
#67162=CARTESIAN_POINT('Ctrl Pts',(-1.65846771681237,5.60071223044711,40.1181397109378));
#67163=CARTESIAN_POINT('Ctrl Pts',(-5.60485522875205,1.64441190725433,40.2769004731838));
#67164=CARTESIAN_POINT('Ctrl Pts',(-4.4215080328057,-3.81690442267336,40.4356612354296));
#67165=CARTESIAN_POINT('Ctrl Pts',(0.808538371485783,-5.78487323610672,
40.5944219976756));
#67166=CARTESIAN_POINT('Ctrl Pts',(5.29858576106737,-2.45834936260147,40.7531827599214));
#67167=CARTESIAN_POINT('Ctrl Pts',(4.93920561471065,3.1181309388157,40.9119435221673));
#67168=CARTESIAN_POINT('Ctrl Pts',(0.0593136197707885,5.84080256047905,
41.0707042844132));
#67169=CARTESIAN_POINT('Ctrl Pts',(-4.87486401174139,3.21779326915472,41.2294650466591));
#67170=CARTESIAN_POINT('Ctrl Pts',(-5.34741719504777,-2.35023871087517,
41.388225808905));
#67171=CARTESIAN_POINT('Ctrl Pts',(-0.925850822461446,-5.76726043373597,
41.5469865711509));
#67172=CARTESIAN_POINT('Ctrl Pts',(4.34308250332321,-3.90590924437788,41.7057473333967));
#67173=CARTESIAN_POINT('Ctrl Pts',(5.63709406088405,1.53024939298615,41.8645080956427));
#67174=CARTESIAN_POINT('Ctrl Pts',(1.77186494664376,5.56587704381296,42.0232688578886));
#67175=CARTESIAN_POINT('Ctrl Pts',(-3.71502908908446,4.50744401221416,42.1820296201344));
#67176=CARTESIAN_POINT('Ctrl Pts',(-5.80181502544146,-0.676339461033121,
42.3407903823803));
#67177=CARTESIAN_POINT('Ctrl Pts',(-2.57860263176698,-5.24111640048504,
42.4995511446262));
#67178=CARTESIAN_POINT('Ctrl Pts',(3.00462565494359,-5.00906351822809,42.6583119068721));
#67179=CARTESIAN_POINT('Ctrl Pts',(5.83792876476416,-0.192562700251437,
42.817072669118));
#67180=CARTESIAN_POINT('Ctrl Pts',(3.32818114721658,4.80017738289961,42.9758334313639));
#67181=CARTESIAN_POINT('Ctrl Pts',(-2.22761951688042,5.39964850189364,43.1345941936098));
#67182=CARTESIAN_POINT('Ctrl Pts',(-5.74463475560437,1.05719637754358,43.2933549558557));
#67183=CARTESIAN_POINT('Ctrl Pts',(-4.0039847938458,-4.25283416401821,43.4521157181015));
#67184=CARTESIAN_POINT('Ctrl Pts',(1.40123435454846,-5.67054097415953,43.6108764803475));
#67185=CARTESIAN_POINT('Ctrl Pts',(5.5240010203993,-1.89839547582067,43.7696372425933));
#67186=CARTESIAN_POINT('Ctrl Pts',(4.59103321957251,3.61121954923408,43.9283980048393));
#67187=CARTESIAN_POINT('Ctrl Pts',(-0.543788418742688,5.81573613669244,
44.0871587670851));
#67188=CARTESIAN_POINT('Ctrl Pts',(-5.18091828599107,2.69751336787648,44.245919529331));
#67189=CARTESIAN_POINT('Ctrl Pts',(-5.07631348469077,-2.88955603183869,
44.4046802915769));
#67190=CARTESIAN_POINT('Ctrl Pts',(-0.325711524187161,-5.83201548857688,
44.5634410538228));
#67191=CARTESIAN_POINT('Ctrl Pts',(4.7229915722406,-3.43683622893689,44.7222018160687));
#67192=CARTESIAN_POINT('Ctrl Pts',(5.44906851609775,2.1038405269557,44.8809625783145));
#67193=CARTESIAN_POINT('Ctrl Pts',(1.18799151005716,5.71901816993276,45.0397233405605));
#67194=CARTESIAN_POINT('Ctrl Pts',(-4.16037161366087,4.09997569410277,45.1984841028063));
#67195=CARTESIAN_POINT('Ctrl Pts',(-5.70103555635091,-1.27148977235826,
45.3572448650522));
#67196=CARTESIAN_POINT('Ctrl Pts',(-2.02393761747008,-5.47924896099626,
45.5160056272981));
#67197=CARTESIAN_POINT('Ctrl Pts',(3.50552985089882,-4.67223213469171,45.674766389544));
#67198=CARTESIAN_POINT('Ctrl Pts',(5.82662932192163,0.410954256471436,45.8335271517899));
#67199=CARTESIAN_POINT('Ctrl Pts',(2.81501966081174,5.11802275935076,45.9922879140358));
#67200=CARTESIAN_POINT('Ctrl Pts',(-2.77298197976823,5.1409205008315,46.1510486762817));
#67201=CARTESIAN_POINT('Ctrl Pts',(-5.82306581062682,0.458690768489886,
46.3098094385276));
#67202=CARTESIAN_POINT('Ctrl Pts',(-3.54370194373858,-4.64334676606566,
46.4685702007734));
#67203=CARTESIAN_POINT('Ctrl Pts',(1.97896618584451,-5.49565150744413,46.6273309630194));
#67204=CARTESIAN_POINT('Ctrl Pts',(5.69042401383344,-1.31816812234872,46.7860917252652));
#67205=CARTESIAN_POINT('Ctrl Pts',(4.19383196809736,4.0657429922898,46.9448524875111));
#67206=CARTESIAN_POINT('Ctrl Pts',(-1.14108319710691,5.72856193064797,47.103613249757));
#67207=CARTESIAN_POINT('Ctrl Pts',(-5.4316441654788,2.14842600887457,47.2623740120029));
#67208=CARTESIAN_POINT('Ctrl Pts',(-4.75099848187323,-3.39801502074773,
47.4211347742488));
#67209=CARTESIAN_POINT('Ctrl Pts',(0.277906133480956,-5.83448890966147,
47.5798955364947));
#67210=CARTESIAN_POINT('Ctrl Pts',(5.05246256671996,-2.93106033166876,47.7386562987406));
#67211=CARTESIAN_POINT('Ctrl Pts',(5.20285092941832,2.65496419227074,47.8974170609865));
#67212=CARTESIAN_POINT('Ctrl Pts',(0.591431198362095,5.8110843905069,48.0561778232323));
#67213=CARTESIAN_POINT('Ctrl Pts',(-4.56128443093633,3.6487226526672,48.2149385854782));
#67214=CARTESIAN_POINT('Ctrl Pts',(-5.53937322279471,-1.85306150857812,
48.3736993477241));
#67215=CARTESIAN_POINT('Ctrl Pts',(-1.44765843879317,-5.65886717467194,
48.53246010997));
#67216=CARTESIAN_POINT('Ctrl Pts',(3.96899756769466,-4.28550475015754,48.6912208722159));
#67217=CARTESIAN_POINT('Ctrl Pts',(5.75310576561908,1.01008252414809,48.8499816344618));
#67218=CARTESIAN_POINT('Ctrl Pts',(2.27179583594514,5.38121141898098,49.0087423967076));
#67219=CARTESIAN_POINT('Ctrl Pts',(-3.28873103569315,4.8272912519194,49.1675031589537));
#67220=CARTESIAN_POINT('Ctrl Pts',(-5.83931080786754,-0.144713320429998,
49.3262639211994));
#67221=CARTESIAN_POINT('Ctrl Pts',(-3.04557496461057,-4.98427184159595,
49.4850246834454));
#67222=CARTESIAN_POINT('Ctrl Pts',(2.53556411455661,-5.26207252676754,49.6437854456913));
#67223=CARTESIAN_POINT('Ctrl Pts',(5.79607746626723,-0.72386370334331,49.8025462079371));
#67224=CARTESIAN_POINT('Ctrl Pts',(3.75184367735869,4.47684729208542,49.961306970183));
#67225=CARTESIAN_POINT('Ctrl Pts',(-1.72619204662586,5.58021089871651,50.120067732429));
#67226=CARTESIAN_POINT('Ctrl Pts',(-5.62436408231579,1.57639504108098,50.2788284946748));
#67227=CARTESIAN_POINT('Ctrl Pts',(-4.37494631143252,-3.87018570976535,
50.4375892569207));
#67228=CARTESIAN_POINT('Ctrl Pts',(0.878555958148904,-5.77465428267269,
50.5963500191666));
#67229=CARTESIAN_POINT('Ctrl Pts',(5.32797697899131,-2.39398286696617,50.7551107814125));
#67230=CARTESIAN_POINT('Ctrl Pts',(4.90107072348494,3.17773479374659,50.9138715436583));
#67231=CARTESIAN_POINT('Ctrl Pts',(-0.0114451633093337,5.84109250604932,
51.0726323059043));
#67232=CARTESIAN_POINT('Ctrl Pts',(-4.91348608704586,3.15850393832203,51.2313930681501));
#67233=CARTESIAN_POINT('Ctrl Pts',(-5.31855445953128,-2.4148439115166,51.3901538303961));
#67234=CARTESIAN_POINT('Ctrl Pts',(-0.855919333292373,-5.77805285116754,
51.5489145926419));
#67235=CARTESIAN_POINT('Ctrl Pts',(4.39007931117216,-3.85301132850749,51.7076753548878));
#67236=CARTESIAN_POINT('Ctrl Pts',(5.61814327333331,1.59842385376603,51.8664361171337));
#67237=CARTESIAN_POINT('Ctrl Pts',(1.70431090331913,5.58693270058057,52.0251968793796));
#67238=CARTESIAN_POINT('Ctrl Pts',(-3.76935886426715,4.46211008474238,52.1839576416255));
#67239=CARTESIAN_POINT('Ctrl Pts',(-5.79319626271042,-0.746571977579234,
52.3427184038713));
#67240=CARTESIAN_POINT('Ctrl Pts',(-2.51492348603726,-5.27196856168236,
52.5014791661173));
#67241=CARTESIAN_POINT('Ctrl Pts',(3.06508408439537,-4.9722984837573,52.6602399283631));
#67242=CARTESIAN_POINT('Ctrl Pts',(5.83983307657691,-0.121828952662795,
52.8190006906091));
#67243=CARTESIAN_POINT('Ctrl Pts',(3.26978845705136,4.84014215722252,52.9777614528549));
#67244=CARTESIAN_POINT('Ctrl Pts',(-2.29286643535651,5.37226732075056,53.1365222151009));
#67245=CARTESIAN_POINT('Ctrl Pts',(-5.75701992960891,0.98752933428568,53.2952829773466));
#67246=CARTESIAN_POINT('Ctrl Pts',(-3.95217293381976,-4.30102566339373,
53.4540437395927));
#67247=CARTESIAN_POINT('Ctrl Pts',(1.46982345169535,-5.65315059739567,53.6128045018384));
#67248=CARTESIAN_POINT('Ctrl Pts',(5.54659251787697,-1.83133942692776,53.7715652640845));
#67249=CARTESIAN_POINT('Ctrl Pts',(4.54695068882314,3.66656952605562,53.9303260263302));
#67250=CARTESIAN_POINT('Ctrl Pts',(-0.61419929905889,5.80872205196845,54.0890867885762));
#67251=CARTESIAN_POINT('Ctrl Pts',(-5.21321532748033,2.63455472619438,54.2478475508221));
#67252=CARTESIAN_POINT('Ctrl Pts',(-5.04093744845616,-2.95083755851469,
54.4066083130679));
#67253=CARTESIAN_POINT('Ctrl Pts',(-0.255039639165707,-5.8355331751643,
54.5653690753139));
#67254=CARTESIAN_POINT('Ctrl Pts',(4.76427823817645,-3.37937058122179,54.7241298375597));
#67255=CARTESIAN_POINT('Ctrl Pts',(5.42318314516584,2.16969519287334,54.8828905998057));
#67256=CARTESIAN_POINT('Ctrl Pts',(1.11862518441343,5.7329896522482,55.0416513620514));
#67257=CARTESIAN_POINT('Ctrl Pts',(-4.20973271396536,4.04927686543645,55.2004121242976));
#67258=CARTESIAN_POINT('Ctrl Pts',(-5.68521464456297,-1.34045779539507,
55.3591728865431));
#67259=CARTESIAN_POINT('Ctrl Pts',(-1.95741447531414,-5.50336453706454,
55.5179336487893));
#67260=CARTESIAN_POINT('Ctrl Pts',(3.56187121174587,-4.62942395195395,55.676694411035));
#67261=CARTESIAN_POINT('Ctrl Pts',(5.82122356704326,0.481506841580768,55.835455173281));
#67262=CARTESIAN_POINT('Ctrl Pts',(2.75281430219354,5.15174786588276,55.9942159355268));
#67263=CARTESIAN_POINT('Ctrl Pts',(-2.83505469783139,5.10695188114131,56.1529766977728));
#67264=CARTESIAN_POINT('Ctrl Pts',(-5.82819504052776,0.388117540903014,
56.3117374600186));
#67265=CARTESIAN_POINT('Ctrl Pts',(-3.48719325759759,-4.6859338279744,56.4704982222645));
#67266=CARTESIAN_POINT('Ctrl Pts',(2.04539431239091,-5.47127542377716,56.6292589845104));
#67267=CARTESIAN_POINT('Ctrl Pts',(5.70597453029646,-1.24913862945516,56.7880197467563));
#67268=CARTESIAN_POINT('Ctrl Pts',(4.14427256681325,4.11624799398041,56.9467805090021));
#67269=CARTESIAN_POINT('Ctrl Pts',(-1.21039423827122,5.71431872089305,57.1055412712481));
#67270=CARTESIAN_POINT('Ctrl Pts',(-5.4572712645165,2.08247040830632,57.2643020334939));
#67271=CARTESIAN_POINT('Ctrl Pts',(-4.709486934955,-3.45531843184919,57.4230627957399));
#67272=CARTESIAN_POINT('Ctrl Pts',(0.348563690628765,-5.8306942991006,57.5818235579858));
#67273=CARTESIAN_POINT('Ctrl Pts',(5.08759817953255,-2.86964064293877,57.7405843202316));
#67274=CARTESIAN_POINT('Ctrl Pts',(5.17030741181829,2.71779578395536,57.8993450824775));
#67275=CARTESIAN_POINT('Ctrl Pts',(0.520993371711727,5.81782249322041,58.0581058447234));
#67276=CARTESIAN_POINT('Ctrl Pts',(-4.60514971613518,3.59320034898822,58.2168666069693));
#67277=CARTESIAN_POINT('Ctrl Pts',(-5.51651911764551,-1.9200285103718,58.3756273692151));
#67278=CARTESIAN_POINT('Ctrl Pts',(-1.37900171841615,-5.67598862900501,
58.5343881314612));
#67279=CARTESIAN_POINT('Ctrl Pts',(4.02062017566359,-4.23711057904269,58.6931488937069));
#67280=CARTESIAN_POINT('Ctrl Pts',(5.74044767353369,1.07970049708729,58.8519096559529));
#67281=CARTESIAN_POINT('Ctrl Pts',(2.20644211632846,5.40833669840192,59.0106704181987));
#67282=CARTESIAN_POINT('Ctrl Pts',(-3.34696666239261,4.78709795354361,59.1694311804446));
#67283=CARTESIAN_POINT('Ctrl Pts',(-5.83712931726406,-0.215439062208749,
59.3281919426906));
#67284=CARTESIAN_POINT('Ctrl Pts',(-2.98497292353889,-5.02079966755579,
59.4869527049364));
#67285=CARTESIAN_POINT('Ctrl Pts',(2.59912186699419,-5.23097105483309,59.6457134671823));
#67286=CARTESIAN_POINT('Ctrl Pts',(5.80442093364305,-0.653597950635783,
59.8044742294282));
#67287=CARTESIAN_POINT('Ctrl Pts',(3.69733666347582,4.52196796239271,59.9632349916741));
#67288=CARTESIAN_POINT('Ctrl Pts',(-1.79366305772334,5.55889067092954,60.1219957539199));
#67289=CARTESIAN_POINT('Ctrl Pts',(-5.64304756034266,1.5081468389052,60.2807565161659));
#67290=CARTESIAN_POINT('Ctrl Pts',(-4.32774256660426,-3.92289904703017,
60.4395172784117));
#67291=CARTESIAN_POINT('Ctrl Pts',(0.948444616708253,-5.76358789861195,
60.5982780406577));
#67292=CARTESIAN_POINT('Ctrl Pts',(5.35658631619137,-2.32926505429939,60.7570388029035));
#67293=CARTESIAN_POINT('Ctrl Pts',(4.86221660003666,3.23687231603548,60.9157995651494));
#67294=CARTESIAN_POINT('Ctrl Pts',(-0.0822022668114812,5.84052527118238,
61.0745603273953));
#67295=CARTESIAN_POINT('Ctrl Pts',(-4.95138710817278,3.09875109697584,61.2333210896412));
#67296=CARTESIAN_POINT('Ctrl Pts',(-5.28891122604591,-2.47909473376766,
61.3920818518871));
#67297=CARTESIAN_POINT('Ctrl Pts',(-0.785862237944882,-5.78799733923239,
61.5508426141331));
#67298=CARTESIAN_POINT('Ctrl Pts',(4.43643187479794,-3.79954798315087,61.7096033763787));
#67299=CARTESIAN_POINT('Ctrl Pts',(5.59836802314956,1.66636374581465,61.8683641386249));
#67300=CARTESIAN_POINT('Ctrl Pts',(1.63650675233685,5.6071684748672,62.0271249008705));
#67301=CARTESIAN_POINT('Ctrl Pts',(-3.82313548596416,4.41612134253018,62.1858856631167));
#67302=CARTESIAN_POINT('Ctrl Pts',(-5.78372734831682,-0.816694934673283,
62.3446464253623));
#67303=CARTESIAN_POINT('Ctrl Pts',(-2.45087527523776,-5.30204706139213,
62.5034071876083));
#67304=CARTESIAN_POINT('Ctrl Pts',(3.12509271269893,-4.93480376438871,62.6621679498542));
#67305=CARTESIAN_POINT('Ctrl Pts',(5.84088039277376,-0.0510773266730637,
62.8209287121001));
#67306=CARTESIAN_POINT('Ctrl Pts',(3.21091592536738,4.879396640591,62.979689474346));
#67307=CARTESIAN_POINT('Ctrl Pts',(-2.35777687563918,5.34409775927519,63.1384502365919));
#67308=CARTESIAN_POINT('Ctrl Pts',(-5.76856026082839,0.917717371079188,
63.2972109988377));
#67309=CARTESIAN_POINT('Ctrl Pts',(-3.89978109233997,-4.34858598717061,
63.4559717610837));
#67310=CARTESIAN_POINT('Ctrl Pts',(1.53819685222249,-5.63493062067332,63.6147325233296));
#67311=CARTESIAN_POINT('Ctrl Pts',(5.56837005279627,-1.76401462893886,63.7734932855754));
#67312=CARTESIAN_POINT('Ctrl Pts',(4.50220089297303,3.72138143372885,63.9322540478213));
#67313=CARTESIAN_POINT('Ctrl Pts',(-0.684520045616047,5.80085553717197,
64.0910148100672));
#67314=CARTESIAN_POINT('Ctrl Pts',(-5.2447473295203,2.57120946355576,64.2497755723131));
#67315=CARTESIAN_POINT('Ctrl Pts',(-5.00482165455439,-3.01168604972238,
64.408536334559));
#67316=CARTESIAN_POINT('Ctrl Pts',(-0.184330327072359,-5.83819449714635,
64.5672970968048));
#67317=CARTESIAN_POINT('Ctrl Pts',(4.80486574618941,-3.32140901080918,64.7260578590508));
#67318=CARTESIAN_POINT('Ctrl Pts',(5.39650192200348,2.23523145597974,64.8848186212967));
#67319=CARTESIAN_POINT('Ctrl Pts',(1.04909470050257,5.74611981822221,65.0435793835425));
#67320=CARTESIAN_POINT('Ctrl Pts',(-4.25847603591327,3.99798380531258,65.2023401457885));
#67321=CARTESIAN_POINT('Ctrl Pts',(-5.66855942741703,-1.40922910622467,
65.3611009080343));
#67322=CARTESIAN_POINT('Ctrl Pts',(-1.8906040825464,-5.52667249428149,65.5198616702802));
#67323=CARTESIAN_POINT('Ctrl Pts',(3.61768986792422,-4.58593640116248,65.6786224325261));
#67324=CARTESIAN_POINT('Ctrl Pts',(5.8149635474948,0.551988765551636,65.8373831947719));
#67325=CARTESIAN_POINT('Ctrl Pts',(2.6902049680239,5.18471695331663,65.996143957018));
#67326=CARTESIAN_POINT('Ctrl Pts',(-2.89671137156331,5.07223381616474,66.1549047192637));
#67327=CARTESIAN_POINT('Ctrl Pts',(-5.83246898269471,0.317487357059558,
66.3136654815097));
#67328=CARTESIAN_POINT('Ctrl Pts',(-3.4301728257792,-4.72783322900402,66.4724262437555));
#67329=CARTESIAN_POINT('Ctrl Pts',(2.11152227728272,-5.44609643033688,66.6311870060015));
#67330=CARTESIAN_POINT('Ctrl Pts',(5.72068769488774,-1.1799258254438,66.7899477682473));
#67331=CARTESIAN_POINT('Ctrl Pts',(4.0941049934505,4.16614893619904,66.9487085304932));
#67332=CARTESIAN_POINT('Ctrl Pts',(-1.27952765405788,5.69923693475624,67.1074692927391));
#67333=CARTESIAN_POINT('Ctrl Pts',(-5.48209750889141,2.01620920516577,67.266230054985));
#67334=CARTESIAN_POINT('Ctrl Pts',(-4.66728427073886,-3.51211477490457,
67.4249908172309));
#67335=CARTESIAN_POINT('Ctrl Pts',(0.419170096048379,-5.82604403403957,
67.5837515794768));
#67336=CARTESIAN_POINT('Ctrl Pts',(5.12198718721476,-2.80779983438927,67.7425123417226));
#67337=CARTESIAN_POINT('Ctrl Pts',(5.13700515150643,2.78022853905663,67.9012731039686));
#67338=CARTESIAN_POINT('Ctrl Pts',(0.45047908927406,5.82370683037148,68.0600338662144));
#67339=CARTESIAN_POINT('Ctrl Pts',(-4.64833919552487,3.53715074308911,68.2187946284603));
#67340=CARTESIAN_POINT('Ctrl Pts',(-5.49285546321007,-1.98671374794472,
68.3775553907063));
#67341=CARTESIAN_POINT('Ctrl Pts',(-1.31014262951052,-5.69227713189796,
68.5363161529521));
#67342=CARTESIAN_POINT('Ctrl Pts',(4.07165275754471,-4.18809461186912,68.6950769151981));
#67343=CARTESIAN_POINT('Ctrl Pts',(5.72694717064212,1.14916002395785,68.8538376774439));
#67344=CARTESIAN_POINT('Ctrl Pts',(2.14076460128891,5.43466830430864,69.0125984396898));
#67345=CARTESIAN_POINT('Ctrl Pts',(-3.40471112167017,4.74620214845141,69.1713592019357));
#67346=CARTESIAN_POINT('Ctrl Pts',(-5.83409122782134,-0.28613318830099,
69.3301199641816));
#67347=CARTESIAN_POINT('Ctrl Pts',(-2.92393283763341,-5.0565906910682,69.4888807264275));
#67348=CARTESIAN_POINT('Ctrl Pts',(2.66229819824794,-5.19910193779603,69.6476414886733));
#67349=CARTESIAN_POINT('Ctrl Pts',(5.81191260213551,-0.583236282416525,
69.8064022509193));
#67350=CARTESIAN_POINT('Ctrl Pts',(3.64228706536681,4.56642503381477,69.9651630131651));
#67351=CARTESIAN_POINT('Ctrl Pts',(-1.86087084873268,5.53675467583008,70.123923775411));
#67352=CARTESIAN_POINT('Ctrl Pts',(-5.66090292103185,1.43967731615189,70.282684537657));
#67353=CARTESIAN_POINT('Ctrl Pts',(-4.27990372547136,-3.97503669878468,
70.4414452999028));
#67354=CARTESIAN_POINT('Ctrl Pts',(1.01819409100193,-5.75167570791655,70.6002060621487));
#67355=CARTESIAN_POINT('Ctrl Pts',(5.38440957424679,-2.26420542194124,70.7589668243946));
#67356=CARTESIAN_POINT('Ctrl Pts',(4.82264894620915,3.29553482724991,70.9177275866405));
#67357=CARTESIAN_POINT('Ctrl Pts',(-0.152947307129394,5.83910093911992,
71.0764883488863));
#67358=CARTESIAN_POINT('Ctrl Pts',(-4.98856151314671,3.03854351384673,71.2352491111322));
#67359=CARTESIAN_POINT('Ctrl Pts',(-5.25849184473667,-2.542981748819,71.3940098733781));
#67360=CARTESIAN_POINT('Ctrl Pts',(-0.71568981729892,-5.79709243857671,
71.5527706356241));
#67361=CARTESIAN_POINT('Ctrl Pts',(4.48213339196102,-3.74552705405491,71.7115313978699));
#67362=CARTESIAN_POINT('Ctrl Pts',(5.57777121235107,1.73405909895161,71.8702921601158));
#67363=CARTESIAN_POINT('Ctrl Pts',(1.56846244395725,5.62658139707268,72.0290529223617));
#67364=CARTESIAN_POINT('Ctrl Pts',(-3.87635106245531,4.36948453442625,72.1878136846075));
#67365=CARTESIAN_POINT('Ctrl Pts',(-5.77340967182392,-0.88669804176993,
72.3465744468535));
#67366=CARTESIAN_POINT('Ctrl Pts',(-2.38646739844469,-5.33134748559404,
72.5053352090994));
#67367=CARTESIAN_POINT('Ctrl Pts',(3.18464273358708,-4.89658486247307,72.6640959713453));
#67368=CARTESIAN_POINT('Ctrl Pts',(5.84107055966092,0.0196817949154431,
72.8228567335911));
#67369=CARTESIAN_POINT('Ctrl Pts',(3.15157219170978,4.91793507240897,72.9816174958371));
#67370=CARTESIAN_POINT('Ctrl Pts',(-2.42234131212014,5.31514395135115,73.1403782580829));
#67371=CARTESIAN_POINT('Ctrl Pts',(-5.77925405571895,0.847770732830903,
73.2991390203289));
#67372=CARTESIAN_POINT('Ctrl Pts',(-3.84681695791018,-4.39550815587048,
73.4578997825747));
#67373=CARTESIAN_POINT('Ctrl Pts',(1.60634452233207,-5.61588371777435,73.6166605448206));
#67374=CARTESIAN_POINT('Ctrl Pts',(5.58933042930359,-1.6964309617693,73.7754213070665));
#67375=CARTESIAN_POINT('Ctrl Pts',(4.45679039905553,3.77564722860532,73.9341820693123));
#67376=CARTESIAN_POINT('Ctrl Pts',(-0.754740338843374,5.79213774671418,
74.0929428315583));
#67377=CARTESIAN_POINT('Ctrl Pts',(-5.2755096647891,2.50748687587913,74.2517035938041));
#67378=CARTESIAN_POINT('Ctrl Pts',(-4.96797140297887,-3.07209257594453,
74.4104643560501));
#67379=CARTESIAN_POINT('Ctrl Pts',(-0.113593964499922,-5.83999906397405,
74.5692251182959));
#67380=CARTESIAN_POINT('Ctrl Pts',(4.84474814006207,-3.26296002356047,74.7279858805419));
#67381=CARTESIAN_POINT('Ctrl Pts',(5.36902876208054,2.30043969882727,74.8867466427877));
#67382=CARTESIAN_POINT('Ctrl Pts',(0.979410261924092,5.75840674100279,75.0455074050336));
#67383=CARTESIAN_POINT('Ctrl Pts',(-4.30659442642138,3.94610404098849,75.2042681672795));
#67384=CARTESIAN_POINT('Ctrl Pts',(-5.65107234906636,-1.477793612656,75.3630289295254));
#67385=CARTESIAN_POINT('Ctrl Pts',(-1.82351624359326,-5.54916941220397,
75.5217896917713));
#67386=CARTESIAN_POINT('Ctrl Pts',(3.6729776280452,-4.54177586411616,75.6805504540171));
#67387=CARTESIAN_POINT('Ctrl Pts',(5.80785018193428,0.622389685160801,75.8393112162631));
#67388=CARTESIAN_POINT('Ctrl Pts',(2.62720084622344,5.21692518343825,75.9980719785088));
#67389=CARTESIAN_POINT('Ctrl Pts',(-2.95794295284595,5.0367714007783,76.1568327407549));
#67390=CARTESIAN_POINT('Ctrl Pts',(-5.83588700992668,0.246810581940319,
76.3155935030007));
#67391=CARTESIAN_POINT('Ctrl Pts',(-3.37264901603277,-4.76903882041673,
76.4743542652466));
#67392=CARTESIAN_POINT('Ctrl Pts',(2.17734037623983,-5.42011822214095,76.6331150274925));
#67393=CARTESIAN_POINT('Ctrl Pts',(5.73456134845009,-1.110539867295,76.7918757897384));
#67394=CARTESIAN_POINT('Ctrl Pts',(4.04333661010157,4.21543849598137,76.9506365519843));
#67395=CARTESIAN_POINT('Ctrl Pts',(-1.34847329913683,5.68331878549001,77.1093973142302));
#67396=CARTESIAN_POINT('Ctrl Pts',(-5.50611925535187,1.94965212328559,77.2681580764761));
#67397=CARTESIAN_POINT('Ctrl Pts',(-4.62439668246642,-3.56839571504929,
77.4269188387219));
#67398=CARTESIAN_POINT('Ctrl Pts',(0.489714988248199,-5.82053879690483,
77.5856796009679));
#67399=CARTESIAN_POINT('Ctrl Pts',(5.15562454317905,-2.74554698116043,77.7444403632137));
#67400=CARTESIAN_POINT('Ctrl Pts',(5.1029490355901,2.8422532955665,77.9032011254596));
#67401=CARTESIAN_POINT('Ctrl Pts',(0.379898699021361,5.82873653843356,78.0619618877055));
#67402=CARTESIAN_POINT('Ctrl Pts',(-4.69084653104859,3.48058206025056,78.2207226499513));
#67403=CARTESIAN_POINT('Ctrl Pts',(-5.46838573213,-2.05310743523703,78.3794834121973));
#67404=CARTESIAN_POINT('Ctrl Pts',(-1.24109127714898,-5.70773029301263,
78.5382441744431));
#67405=CARTESIAN_POINT('Ctrl Pts',(4.12208782430557,-4.13846404173107,78.6970049366891));
#67406=CARTESIAN_POINT('Ctrl Pts',(5.71260623814347,1.21845091157291,78.8557656989349));
#67407=CARTESIAN_POINT('Ctrl Pts',(2.07477292900298,5.46020237253759,79.0145264611808));
#67408=CARTESIAN_POINT('Ctrl Pts',(-3.46195593952531,4.70460983810283,79.1732872234267));
#67409=CARTESIAN_POINT('Ctrl Pts',(-5.83019698537905,-0.356785324342241,
79.3320479856726));
#67410=CARTESIAN_POINT('Ctrl Pts',(-2.86246366452812,-5.09163965979981,
79.4908087479185));
#67411=CARTESIAN_POINT('Ctrl Pts',(2.72508383719022,-5.16646985244982,79.6495695101644));
#67412=CARTESIAN_POINT('Ctrl Pts',(5.81855137234204,-0.512789024261698,
79.8083302724102));
#67413=CARTESIAN_POINT('Ctrl Pts',(3.58670296156134,4.61021198227599,79.9670910346562));
#67414=CARTESIAN_POINT('Ctrl Pts',(-1.92780555690993,5.51380616187509,80.1258517969019));
#67415=CARTESIAN_POINT('Ctrl Pts',(-5.67792754410753,1.37099652072606,80.2846125591481));
#67416=CARTESIAN_POINT('Ctrl Pts',(-4.23143680838723,-4.02659101382961,
80.4433733213938));
#67417=CARTESIAN_POINT('Ctrl Pts',(1.08779414529793,-5.73891945869655,80.6021340836398));
#67418=CARTESIAN_POINT('Ctrl Pts',(5.41144267008512,-2.19881351740198,80.7608948458856));
#67419=CARTESIAN_POINT('Ctrl Pts',(4.7823735685733,3.3537137186807,80.9196556081314));
#67420=CARTESIAN_POINT('Ctrl Pts',(-0.223669902459649,5.83681971885304,
81.0784163703775));
#67421=CARTESIAN_POINT('Ctrl Pts',(-5.02500384656033,2.97789002445559,81.2371771326232));
#67422=CARTESIAN_POINT('Ctrl Pts',(-5.22730077976831,-2.60649558135874,
81.3959378948693));
#67423=CARTESIAN_POINT('Ctrl Pts',(-0.645412368928784,-5.8053368142863,
81.5546986571149));
#67424=CARTESIAN_POINT('Ctrl Pts',(4.52717715552302,-3.69095646919078,81.713459419361));
#67425=CARTESIAN_POINT('Ctrl Pts',(5.5563558643626,1.80149997964642,81.8722201816067));
#67426=CARTESIAN_POINT('Ctrl Pts',(1.5001879620707,5.64516861688714,82.0309809438528));
#67427=CARTESIAN_POINT('Ctrl Pts',(-3.92899778126385,4.3222065071854,82.1897417060986));
#67428=CARTESIAN_POINT('Ctrl Pts',(-5.76224475326896,-0.956571031279116,
82.3485024683446));
#67429=CARTESIAN_POINT('Ctrl Pts',(-2.32170929618077,-5.35986552417092,
82.5072632305903));
#67430=CARTESIAN_POINT('Ctrl Pts',(3.24372538638481,-4.8576474063222,82.6660239928364));
#67431=CARTESIAN_POINT('Ctrl Pts',(5.8404035909078,0.0904380659057711,82.8247847550821));
#67432=CARTESIAN_POINT('Ctrl Pts',(3.09176588514392,4.95575172494502,82.9835455173283));
#67433=CARTESIAN_POINT('Ctrl Pts',(-2.48655011745873,5.28541028426119,83.1423062795738));
#67434=CARTESIAN_POINT('Ctrl Pts',(-5.78910003705706,0.777699419312094,
83.30106704182));
#67435=CARTESIAN_POINT('Ctrl Pts',(-3.79328774359228,-4.44178477631751,
83.4598278040656));
#67436=CARTESIAN_POINT('Ctrl Pts',(1.67425538991496,-5.59601365552512,83.6185885663117));
#67437=CARTESIAN_POINT('Ctrl Pts',(5.60947262352764,-1.6285964822938,83.7773493285575));
#67438=CARTESIAN_POINT('Ctrl Pts',(4.41072194085603,3.82935538285094,83.9361100908034));
#67439=CARTESIAN_POINT('Ctrl Pts',(-0.8248423466062,5.78257678649102,84.0948708530494));
#67440=CARTESIAN_POINT('Ctrl Pts',(-5.30551223554587,2.44338323992171,84.253631615295));
#67441=CARTESIAN_POINT('Ctrl Pts',(-4.9303644901222,-3.13202323158636,84.4123923775413));
#67442=CARTESIAN_POINT('Ctrl Pts',(-0.0428938145929691,-5.84099457038411,
84.5711531397868));
#67443=CARTESIAN_POINT('Ctrl Pts',(4.88402085037918,-3.20394034224944,84.729913902033));
#67444=CARTESIAN_POINT('Ctrl Pts',(5.3405737125575,2.36513442508082,84.8886746642787));
#67445=CARTESIAN_POINT('Ctrl Pts',(0.90995364228369,5.77018558745976,85.0474354265247));
#67446=CARTESIAN_POINT('Ctrl Pts',(-4.35479260506382,3.89299956501012,85.2061961887705));
#67447=CARTESIAN_POINT('Ctrl Pts',(-5.63139114508318,-1.54490255601334,
85.3649569510165));
#67448=CARTESIAN_POINT('Ctrl Pts',(-1.75878919991609,-5.5732440393258,85.5237177132622));
#67449=CARTESIAN_POINT('Ctrl Pts',(3.73289035077776,-4.49219002151886,85.6824784755083));
#67450=CARTESIAN_POINT('Ctrl Pts',(5.44619302579455,-0.180386406182261,
85.814779110713));
#67451=CARTESIAN_POINT('Ctrl Pts',(4.18934532924144,2.98339184141738,85.9206196188771));
#67452=CARTESIAN_POINT('Ctrl Pts',(2.90742207776985,4.07986902565238,85.973539872959));
#67453=CARTESIAN_POINT('Ctrl Pts',(2.16917135428672,4.4405021828327,86.));
#67454=CARTESIAN_POINT('Ctrl Pts',(2.75898463274055,-3.86904481704483,25.7806068977079));
#67455=CARTESIAN_POINT('Ctrl Pts',(3.40222835107826,-3.41035291299081,25.8070670247489));
#67456=CARTESIAN_POINT('Ctrl Pts',(4.44488144388779,-2.1678284260566,25.8599872788309));
#67457=CARTESIAN_POINT('Ctrl Pts',(5.13713708894935,1.03153993625474,25.9658277869948));
#67458=CARTESIAN_POINT('Ctrl Pts',(2.83087052930385,4.85053885500829,26.0981284221998));
#67459=CARTESIAN_POINT('Ctrl Pts',(-2.54870530784567,5.00827073567408,26.2568891844456));
#67460=CARTESIAN_POINT('Ctrl Pts',(-5.58537388969466,0.575612517731738,
26.4156499466916));
#67461=CARTESIAN_POINT('Ctrl Pts',(-3.51540226351445,-4.38046981539479,
26.5744107089373));
#67462=CARTESIAN_POINT('Ctrl Pts',(1.77471175523205,-5.32917482126994,26.7331714711833));
#67463=CARTESIAN_POINT('Ctrl Pts',(5.43912643226927,-1.39953709723575,26.8919322334291));
#67464=CARTESIAN_POINT('Ctrl Pts',(4.12623242092013,3.81051993270251,27.0506929956751));
#67465=CARTESIAN_POINT('Ctrl Pts',(-0.963505012884285,5.53332322688231,
27.2094537579209));
#67466=CARTESIAN_POINT('Ctrl Pts',(-5.17120987535828,2.19172929477075,27.3682145201668));
#67467=CARTESIAN_POINT('Ctrl Pts',(-4.64617167900849,-3.15573394561846,
27.5269752824127));
#67468=CARTESIAN_POINT('Ctrl Pts',(0.131240194292791,-5.61500874158838,
27.6857360446586));
#67469=CARTESIAN_POINT('Ctrl Pts',(4.78850808778552,-2.93523740776727,27.8444968069045));
#67470=CARTESIAN_POINT('Ctrl Pts',(5.06320222551221,2.43094313930505,28.0032575691504));
#67471=CARTESIAN_POINT('Ctrl Pts',(0.703891137995956,5.57225534640277,28.1620183313963));
#67472=CARTESIAN_POINT('Ctrl Pts',(-4.29963849958627,3.61366660379846,28.3207790936422));
#67473=CARTESIAN_POINT('Ctrl Pts',(-5.36800979937294,-1.65225881189325,
28.4795398558881));
#67474=CARTESIAN_POINT('Ctrl Pts',(-1.52341343958394,-5.40598721644804,
28.638300618134));
#67475=CARTESIAN_POINT('Ctrl Pts',(3.7154568469317,-4.21199061529042,28.7970613803798));
#67476=CARTESIAN_POINT('Ctrl Pts',(5.55382784322941,0.836948256968893,28.9558221426258));
#67477=CARTESIAN_POINT('Ctrl Pts',(2.30916579364752,5.11988662236081,29.1145829048716));
#67478=CARTESIAN_POINT('Ctrl Pts',(-3.04891524119282,4.71694830830577,29.2733436671175));
#67479=CARTESIAN_POINT('Ctrl Pts',(-5.61653596054952,-0.00308515054028371,
29.4321044293634));
#67480=CARTESIAN_POINT('Ctrl Pts',(-3.04373138672984,-4.72029500001125,
29.5908651916093));
#67481=CARTESIAN_POINT('Ctrl Pts',(2.31478911232886,-5.11734667454166,29.7496259538552));
#67482=CARTESIAN_POINT('Ctrl Pts',(5.55474391583396,-0.830846365132238,
29.908386716101));
#67483=CARTESIAN_POINT('Ctrl Pts',(3.71082741246647,4.21606991826224,30.067147478347));
#67484=CARTESIAN_POINT('Ctrl Pts',(-1.52935168579825,5.40431022984286,30.2259082405928));
#67485=CARTESIAN_POINT('Ctrl Pts',(-5.36982140744797,1.64636074283387,30.3846690028388));
#67486=CARTESIAN_POINT('Ctrl Pts',(-4.29566655320965,-3.61838838505691,
30.5434297650846));
#67487=CARTESIAN_POINT('Ctrl Pts',(0.710013543128747,-5.57147793767643,
30.7021905273306));
#67488=CARTESIAN_POINT('Ctrl Pts',(5.06586755727536,-2.42538069880583,30.8609512895764));
#67489=CARTESIAN_POINT('Ctrl Pts',(4.78528484399858,2.94049903987215,31.0197120518223));
#67490=CARTESIAN_POINT('Ctrl Pts',(0.125063273099813,5.61514423852442,31.1784728140682));
#67491=CARTESIAN_POINT('Ctrl Pts',(-4.64962002546522,3.15063791327663,31.3372335763141));
#67492=CARTESIAN_POINT('Ctrl Pts',(-5.16882905222222,-2.19742846769609,
31.49599433856));
#67493=CARTESIAN_POINT('Ctrl Pts',(-0.957367846451143,-5.5343411937037,
31.6547551008058));
#67494=CARTESIAN_POINT('Ctrl Pts',(4.13030565557618,-3.80605581058243,31.8135158630518));
#67495=CARTESIAN_POINT('Ctrl Pts',(5.4377972597899,1.40564810787321,31.9722766252976));
#67496=CARTESIAN_POINT('Ctrl Pts',(1.76845071216457,5.33085994192234,32.1310373875435));
#67497=CARTESIAN_POINT('Ctrl Pts',(-3.51943594526451,4.37710592388724,32.2897981497894));
#67498=CARTESIAN_POINT('Ctrl Pts',(-5.58622732301659,-0.582709136130893,
32.4485589120353));
#67499=CARTESIAN_POINT('Ctrl Pts',(-2.54033282120867,-5.00921099567965,
32.6073196742812));
#67500=CARTESIAN_POINT('Ctrl Pts',(2.83055187404587,-4.8511299436403,32.7660804365271));
#67501=CARTESIAN_POINT('Ctrl Pts',(5.61082903384082,-0.253146587487778,
32.9248411987729));
#67502=CARTESIAN_POINT('Ctrl Pts',(3.25590407686029,4.57652425799672,33.0836019610189));
#67503=CARTESIAN_POINT('Ctrl Pts',(-2.07892374414776,5.217620310809,33.2423627232647));
#67504=CARTESIAN_POINT('Ctrl Pts',(-5.51105705295918,1.08339088088132,33.4011234855107));
#67505=CARTESIAN_POINT('Ctrl Pts',(-3.8993026094728,-4.0423909758343,33.5598842477566));
#67506=CARTESIAN_POINT('Ctrl Pts',(1.28121268795212,-5.46845313502624,33.7186450100024));
#67507=CARTESIAN_POINT('Ctrl Pts',(5.28912299821215,-1.88961994896626,33.8774057722484));
#67508=CARTESIAN_POINT('Ctrl Pts',(4.45626638214284,3.41865113358054,34.0361665344941));
#67509=CARTESIAN_POINT('Ctrl Pts',(-0.455101345292619,5.59806827461589,
34.1949272967401));
#67510=CARTESIAN_POINT('Ctrl Pts',(-4.94994642026466,2.65396233550082,34.353688058986));
#67511=CARTESIAN_POINT('Ctrl Pts',(-4.91444933332838,-2.71913099939964,
34.5124488212319));
#67512=CARTESIAN_POINT('Ctrl Pts',(-0.381098102720512,-5.60359258671175,
34.6712095834778));
#67513=CARTESIAN_POINT('Ctrl Pts',(4.50104575229031,-3.35947507470101,34.8299703457236));
#67514=CARTESIAN_POINT('Ctrl Pts',(5.26369504857235,1.95933664217838,34.9887311079696));
#67515=CARTESIAN_POINT('Ctrl Pts',(1.20884985474224,5.48490361541909,35.1474918702154));
#67516=CARTESIAN_POINT('Ctrl Pts',(-3.95237165094757,3.99051926126589,35.3062526324614));
#67517=CARTESIAN_POINT('Ctrl Pts',(-5.49626189492614,-1.15611021279586,
35.4650133947072));
#67518=CARTESIAN_POINT('Ctrl Pts',(-2.00980536716273,-5.24463230626054,
35.6237741569531));
#67519=CARTESIAN_POINT('Ctrl Pts',(3.31608642293227,-4.53310671365589,35.782534919199));
#67520=CARTESIAN_POINT('Ctrl Pts',(5.60699462758102,0.327256608834102,35.9412956814449));
#67521=CARTESIAN_POINT('Ctrl Pts',(2.76621008118667,4.88810468673588,36.1000564436907));
#67522=CARTESIAN_POINT('Ctrl Pts',(-2.60629442649681,4.97521004623518,36.2588172059367));
#67523=CARTESIAN_POINT('Ctrl Pts',(-5.59343866475058,0.508851201650464,
36.4175779681825));
#67524=CARTESIAN_POINT('Ctrl Pts',(-3.46129698321598,-4.42322380574711,
36.5763387304285));
#67525=CARTESIAN_POINT('Ctrl Pts',(1.83872942405087,-5.30702927699456,36.7350994926743));
#67526=CARTESIAN_POINT('Ctrl Pts',(5.4558944977048,-1.33367944861663,36.8938602549202));
#67527=CARTESIAN_POINT('Ctrl Pts',(4.07965827459196,3.86029454890444,37.0526210171661));
#67528=CARTESIAN_POINT('Ctrl Pts',(-1.03040581621204,5.52120906103586,37.211381779412));
#67529=CARTESIAN_POINT('Ctrl Pts',(-5.1974110298633,2.12894439298054,37.3701425416579));
#67530=CARTESIAN_POINT('Ctrl Pts',(-4.60758691199661,-3.21179521298375,
37.5289033039038));
#67531=CARTESIAN_POINT('Ctrl Pts',(0.199241488304119,-5.61300173446314,
37.6876640661497));
#67532=CARTESIAN_POINT('Ctrl Pts',(4.82371799259843,-2.87701761719148,37.8464248283956));
#67533=CARTESIAN_POINT('Ctrl Pts',(5.03338044768208,2.49210090298119,38.0051855906414));
#67534=CARTESIAN_POINT('Ctrl Pts',(0.636339370439441,5.58037255453223,38.1639463528873));
#67535=CARTESIAN_POINT('Ctrl Pts',(-4.34309893586852,3.56131678947628,38.3227071151332));
#67536=CARTESIAN_POINT('Ctrl Pts',(-5.34760043438529,-1.71716488314614,
38.4814678773791));
#67537=CARTESIAN_POINT('Ctrl Pts',(-1.45781467077047,-5.4240448032289,38.640228639625));
#67538=CARTESIAN_POINT('Ctrl Pts',(3.76620760906239,-4.16667323979076,38.7989894018709));
#67539=CARTESIAN_POINT('Ctrl Pts',(5.54328164477202,0.904164945395139,38.9577501641167));
#67540=CARTESIAN_POINT('Ctrl Pts',(2.2469749974438,5.14748375447756,39.1165109263627));
#67541=CARTESIAN_POINT('Ctrl Pts',(-3.10583180228996,4.67966819952357,39.2752716886085));
#67542=CARTESIAN_POINT('Ctrl Pts',(-5.61608646770029,-0.0711226339607316,
39.4340324508545));
#67543=CARTESIAN_POINT('Ctrl Pts',(-2.98632725227654,-4.75681986037505,
39.5927932131003));
#67544=CARTESIAN_POINT('Ctrl Pts',(2.37660988298438,-5.08893025161958,39.7515539753462));
#67545=CARTESIAN_POINT('Ctrl Pts',(5.56440105884388,-0.763496233183334,
39.9103147375921));
#67546=CARTESIAN_POINT('Ctrl Pts',(3.65948241880601,4.26071285915838,40.069075499838));
#67547=CARTESIAN_POINT('Ctrl Pts',(-1.59470631126904,5.3853873976295,40.2278362620839));
#67548=CARTESIAN_POINT('Ctrl Pts',(-5.38937111433215,1.58119089099016,40.3865970243298));
#67549=CARTESIAN_POINT('Ctrl Pts',(-4.25151885307432,-3.67015981718801,
40.5453577865757));
#67550=CARTESIAN_POINT('Ctrl Pts',(0.777453326851397,-5.56246815418439,
40.7041185488216));
#67551=CARTESIAN_POINT('Ctrl Pts',(5.09487647442165,-2.36383572866916,40.8628793110675));
#67552=CARTESIAN_POINT('Ctrl Pts',(4.74931304757294,2.9982513600266,41.0216400733133));
#67553=CARTESIAN_POINT('Ctrl Pts',(0.0570332499295138,5.61624722124574,
41.1804008355593));
#67554=CARTESIAN_POINT('Ctrl Pts',(-4.6874451201527,3.09408207507567,41.3391615978051));
#67555=CARTESIAN_POINT('Ctrl Pts',(-5.14183053639566,-2.25988149617119,
41.497922360051));
#67556=CARTESIAN_POINT('Ctrl Pts',(-0.89025558647059,-5.5455324931431,41.6566831222969));
#67557=CARTESIAN_POINT('Ctrl Pts',(4.17610846940334,-3.75574276189485,41.8154438845428));
#67558=CARTESIAN_POINT('Ctrl Pts',(5.4203704931852,1.47141746569594,41.9742046467887));
#67559=CARTESIAN_POINT('Ctrl Pts',(1.70374387423147,5.35189148365012,42.1329654090346));
#67560=CARTESIAN_POINT('Ctrl Pts',(-3.57220117995318,4.33415094011377,42.2917261712804));
#67561=CARTESIAN_POINT('Ctrl Pts',(-5.57875859993888,-0.65033693217899,
42.4504869335264));
#67562=CARTESIAN_POINT('Ctrl Pts',(-2.47946574386026,-5.03961657934126,
42.6092476957722));
#67563=CARTESIAN_POINT('Ctrl Pts',(2.88910989726652,-4.81648519599765,42.7680084580182));
#67564=CARTESIAN_POINT('Ctrl Pts',(5.61348391140414,-0.185159439821055,
42.926769220264));
#67565=CARTESIAN_POINT('Ctrl Pts',(3.200225983726,4.61562989144849,43.0855299825099));
#67566=CARTESIAN_POINT('Ctrl Pts',(-2.14197651643363,5.19205375981362,43.2442907447558));
#67567=CARTESIAN_POINT('Ctrl Pts',(-5.52377668122861,1.01655143385025,43.4030515070017));
#67568=CARTESIAN_POINT('Ctrl Pts',(-3.8500477014075,-4.08932981534074,43.5618122692476));
#67569=CARTESIAN_POINT('Ctrl Pts',(1.34736253598006,-5.45253150732624,43.7205730314935));
#67570=CARTESIAN_POINT('Ctrl Pts',(5.31162542471411,-1.82540981406326,43.8793337937394));
#67571=CARTESIAN_POINT('Ctrl Pts',(4.41452647903867,3.47238269889917,44.0380945559852));
#67572=CARTESIAN_POINT('Ctrl Pts',(-0.522881943720034,5.59214450051854,
44.1968553182311));
#67573=CARTESIAN_POINT('Ctrl Pts',(-4.98173283994925,2.59380484098539,44.355616080477));
#67574=CARTESIAN_POINT('Ctrl Pts',(-4.88114967204592,-2.77846423781803,
44.5143768427229));
#67575=CARTESIAN_POINT('Ctrl Pts',(-0.313189227628139,-5.60779797687521,
44.6731376049688));
#67576=CARTESIAN_POINT('Ctrl Pts',(4.54141156440446,-3.30470371507665,44.8318983672147));
#67577=CARTESIAN_POINT('Ctrl Pts',(5.23957377347164,2.02295633024942,44.9906591294605));
#67578=CARTESIAN_POINT('Ctrl Pts',(1.14231802019273,5.49914495012552,45.1494198917065));
#67579=CARTESIAN_POINT('Ctrl Pts',(-4.00042207772478,3.94234813807709,45.3081806539523));
#67580=CARTESIAN_POINT('Ctrl Pts',(-5.48185369562519,-1.22260611053129,
45.4669414161983));
#67581=CARTESIAN_POINT('Ctrl Pts',(-1.94612536588803,-5.26859390179156,
45.6257021784441));
#67582=CARTESIAN_POINT('Ctrl Pts',(3.37075634388315,-4.492603622836,45.7844629406901));
#67583=CARTESIAN_POINT('Ctrl Pts',(5.60261888663935,0.395154720103479,45.9432237029359));
#67584=CARTESIAN_POINT('Ctrl Pts',(2.70679349012103,4.92125539304622,46.1019844651818));
#67585=CARTESIAN_POINT('Ctrl Pts',(-2.66637198863979,4.94327280856975,46.2607452274277));
#67586=CARTESIAN_POINT('Ctrl Pts',(-5.59919237800458,0.441055955456253,
46.4195059896736));
#67587=CARTESIAN_POINT('Ctrl Pts',(-3.40746087346144,-4.46482878032041,
46.5782667519195));
#67588=CARTESIAN_POINT('Ctrl Pts',(1.90288290472123,-5.28436583637694,46.7370275141654));
#67589=CARTESIAN_POINT('Ctrl Pts',(5.47165012418784,-1.26748986592512,46.8957882764113));
#67590=CARTESIAN_POINT('Ctrl Pts',(4.03259601626857,3.90943154580342,47.0545490386571));
#67591=CARTESIAN_POINT('Ctrl Pts',(-1.09721314298891,5.50832179167125,47.2133098009031));
#67592=CARTESIAN_POINT('Ctrl Pts',(-5.22281931897105,2.06582767992164,47.3720705631488));
#67593=CARTESIAN_POINT('Ctrl Pts',(-4.56834172113761,-3.26737502602034,
47.5308313253949));
#67594=CARTESIAN_POINT('Ctrl Pts',(0.267221761695801,-5.61017630487886,
47.6895920876407));
#67595=CARTESIAN_POINT('Ctrl Pts',(4.85821572583019,-2.81837286444571,47.8483528498866));
#67596=CARTESIAN_POINT('Ctrl Pts',(5.00282226155327,2.5528915098482,48.0071136121325));
#67597=CARTESIAN_POINT('Ctrl Pts',(0.568693050307066,5.58767159524255,48.1658743743783));
#67598=CARTESIAN_POINT('Ctrl Pts',(-4.38592141153559,3.50844395901968,48.3246351366243));
#67599=CARTESIAN_POINT('Ctrl Pts',(-5.32640662782695,-1.78181875531413,
48.4833958988701));
#67600=CARTESIAN_POINT('Ctrl Pts',(-1.39200180112221,-5.44130651842186,
48.6421566611161));
#67601=CARTESIAN_POINT('Ctrl Pts',(3.81640559321821,-4.12074434899823,48.8009174233619));
#67602=CARTESIAN_POINT('Ctrl Pts',(5.53192201501862,0.971248918403669,48.9596781856079));
#67603=CARTESIAN_POINT('Ctrl Pts',(2.18445443391585,5.17432550849803,49.1184389478537));
#67604=CARTESIAN_POINT('Ctrl Pts',(-3.16229257013621,4.64170134138436,49.2771997100997));
#67605=CARTESIAN_POINT('Ctrl Pts',(-5.61481282051529,-0.139149675977844,
49.4359604723455));
#67606=CARTESIAN_POINT('Ctrl Pts',(-2.92848487086811,-4.79264665950293,
49.5947212345914));
#67607=CARTESIAN_POINT('Ctrl Pts',(2.43808188433272,-5.05976702695259,49.7534819968373));
#67608=CARTESIAN_POINT('Ctrl Pts',(5.57324162681136,-0.696034058739029,
49.9122427590832));
#67609=CARTESIAN_POINT('Ctrl Pts',(3.60760039555022,4.30473054066965,50.0710035213291));
#67610=CARTESIAN_POINT('Ctrl Pts',(-1.65982691330743,5.36567425955101,50.229764283575));
#67611=CARTESIAN_POINT('Ctrl Pts',(-5.40812993103286,1.515788999437,50.3885250458208));
#67612=CARTESIAN_POINT('Ctrl Pts',(-4.20674724239739,-3.7213926533396,50.5472858080668));
#67613=CARTESIAN_POINT('Ctrl Pts',(0.844779019247828,-5.55264207836113,
50.7060465703126));
#67614=CARTESIAN_POINT('Ctrl Pts',(5.12313771836632,-2.30194386560584,50.8648073325585));
#67615=CARTESIAN_POINT('Ctrl Pts',(4.71264428935673,3.05556368674283,51.0235680948044));
#67616=CARTESIAN_POINT('Ctrl Pts',(-0.0110051428662697,5.61652601957635,
51.1823288570503));
#67617=CARTESIAN_POINT('Ctrl Pts',(-4.7245823321816,3.03707218027256,51.3410896192961));
#67618=CARTESIAN_POINT('Ctrl Pts',(-5.11407745683792,-2.32200288699436,
51.4998503815421));
#67619=CARTESIAN_POINT('Ctrl Pts',(-0.82301268146625,-5.55590998558236,
51.6586111437879));
#67620=CARTESIAN_POINT('Ctrl Pts',(4.22129843923301,-3.70487855788512,51.8173719060339));
#67621=CARTESIAN_POINT('Ctrl Pts',(5.40214828710646,1.53697089297761,51.9761326682797));
#67622=CARTESIAN_POINT('Ctrl Pts',(1.63878701185215,5.37213763520004,52.1348934305256));
#67623=CARTESIAN_POINT('Ctrl Pts',(-3.62444219405034,4.29055991960671,52.2936541927716));
#67624=CARTESIAN_POINT('Ctrl Pts',(-5.57047119392959,-0.717869291269865,
52.4524149550173));
#67625=CARTESIAN_POINT('Ctrl Pts',(-2.41823480486641,-5.06928259917325,
52.6111757172634));
#67626=CARTESIAN_POINT('Ctrl Pts',(2.94724394355444,-4.78113362906013,52.7699364795091));
#67627=CARTESIAN_POINT('Ctrl Pts',(5.6153150100958,-0.117145120002924,52.9286972417552));
#67628=CARTESIAN_POINT('Ctrl Pts',(3.14407825736721,4.65405818112524,53.0874580040009));
#67629=CARTESIAN_POINT('Ctrl Pts',(-2.20471495362471,5.16572527482943,53.2462187662469));
#67630=CARTESIAN_POINT('Ctrl Pts',(-5.53568569516419,0.949562807876645,
53.4049795284926));
#67631=CARTESIAN_POINT('Ctrl Pts',(-3.80022779876814,-4.13566854561846,
53.5637402907387));
#67632=CARTESIAN_POINT('Ctrl Pts',(1.41331465853004,-5.43580972052295,53.7225010529844));
#67633=CARTESIAN_POINT('Ctrl Pts',(5.33334837008319,-1.76093180023503,53.8812618152305));
#67634=CARTESIAN_POINT('Ctrl Pts',(4.37213874408905,3.52560469199021,54.0400225774763));
#67635=CARTESIAN_POINT('Ctrl Pts',(-0.590585809212258,5.58540007910849,
54.1987833397222));
#67636=CARTESIAN_POINT('Ctrl Pts',(-5.01278819024406,2.53326670555979,54.3575441019681));
#67637=CARTESIAN_POINT('Ctrl Pts',(-4.8471337019555,-2.83738973655626,54.516304864214));
#67638=CARTESIAN_POINT('Ctrl Pts',(-0.245234392010581,-5.61118042257805,
54.6750656264598));
#67639=CARTESIAN_POINT('Ctrl Pts',(4.58111092428449,-3.2494473901187,54.8338263887058));
#67640=CARTESIAN_POINT('Ctrl Pts',(5.21468359081919,2.08627914944017,54.9925871509516));
#67641=CARTESIAN_POINT('Ctrl Pts',(1.07561855045193,5.51257928520504,55.1513479131975));
#67642=CARTESIAN_POINT('Ctrl Pts',(-4.04788544248539,3.89359847522351,55.3101086754434));
#67643=CARTESIAN_POINT('Ctrl Pts',(-5.46664103418928,-1.28892259079655,
55.4688694376893));
#67644=CARTESIAN_POINT('Ctrl Pts',(-1.88215977067859,-5.29178233106645,
55.6276301999352));
#67645=CARTESIAN_POINT('Ctrl Pts',(3.42493160627594,-4.45144124234838,55.7863909621811));
#67646=CARTESIAN_POINT('Ctrl Pts',(5.59742096126865,0.46299484241015,55.9451517244269));
#67647=CARTESIAN_POINT('Ctrl Pts',(2.64697967705877,4.95368390503328,56.1039124866729));
#67648=CARTESIAN_POINT('Ctrl Pts',(-2.72605826064226,4.91061014552488,56.2626732489187));
#67649=CARTESIAN_POINT('Ctrl Pts',(-5.60412440966974,0.373195984292183,
56.4214340111647));
#67650=CARTESIAN_POINT('Ctrl Pts',(-3.35312471875849,-4.5057785411845,56.5801947734105));
#67651=CARTESIAN_POINT('Ctrl Pts',(1.96675713728871,-5.26092691497154,56.7389555356564));
#67652=CARTESIAN_POINT('Ctrl Pts',(5.48660278591027,-1.20111427907158,56.8977162979024));
#67653=CARTESIAN_POINT('Ctrl Pts',(3.9849419744025,3.95799483354801,57.0564770601482));
#67654=CARTESIAN_POINT('Ctrl Pts',(-1.1638594537159,5.49462617597814,57.2152378223941));
#67655=CARTESIAN_POINT('Ctrl Pts',(-5.24746115924365,2.00240780661117,57.37399858464));
#67656=CARTESIAN_POINT('Ctrl Pts',(-4.52842612604344,-3.32247535170916,
57.5327593468859));
#67657=CARTESIAN_POINT('Ctrl Pts',(0.335162820288752,-5.60652758181426,
57.6915201091317));
#67658=CARTESIAN_POINT('Ctrl Pts',(4.89200051581106,-2.75931451542811,57.8502808713777));
#67659=CARTESIAN_POINT('Ctrl Pts',(4.97152991116165,2.61330747983713,58.0090416336235));
#67660=CARTESIAN_POINT('Ctrl Pts',(0.500963274458718,5.59415064503912,58.1678023958695));
#67661=CARTESIAN_POINT('Ctrl Pts',(-4.42810025315133,3.45505626434493,58.3265631581152));
#67662=CARTESIAN_POINT('Ctrl Pts',(-5.30443117099388,-1.84621114554552,
58.4853239203613));
#67663=CARTESIAN_POINT('Ctrl Pts',(-1.325984655183,-5.45776972177896,58.644084682607));
#67664=CARTESIAN_POINT('Ctrl Pts',(3.86604351978,-4.07421073889346,58.802845444853));
#67665=CARTESIAN_POINT('Ctrl Pts',(5.51975057560345,1.03819036061473,58.9616062070988));
#67666=CARTESIAN_POINT('Ctrl Pts',(2.12161330165796,5.20040793015086,59.1203669693448));
#67667=CARTESIAN_POINT('Ctrl Pts',(-3.21828927148705,4.60305331348437,59.2791277315906));
#67668=CARTESIAN_POINT('Ctrl Pts',(-5.61271519944128,-0.207156297777243,
59.4378884938366));
#67669=CARTESIAN_POINT('Ctrl Pts',(-2.8702127342488,-4.82777013764157,59.5966492560824));
#67670=CARTESIAN_POINT('Ctrl Pts',(2.49919609711769,-5.02986128137743,59.7554100183283));
#67671=CARTESIAN_POINT('Ctrl Pts',(5.58126432146331,-0.6284697412833,59.9141707805742));
#67672=CARTESIAN_POINT('Ctrl Pts',(3.55518895686721,4.34811650289146,60.0729315428202));
#67673=CARTESIAN_POINT('Ctrl Pts',(-1.72470393571439,5.34517370867209,60.2316923050659));
#67674=CARTESIAN_POINT('Ctrl Pts',(-5.42609510456254,1.45016466581917,60.3904530673119));
#67675=CARTESIAN_POINT('Ctrl Pts',(-4.161358291482,-3.7720793750479,60.5492138295578));
#67676=CARTESIAN_POINT('Ctrl Pts',(0.911980740306919,-5.54200115220642,
60.7079745918037));
#67677=CARTESIAN_POINT('Ctrl Pts',(5.15064714175253,-2.23971419223624,60.8667353540495));
#67678=CARTESIAN_POINT('Ctrl Pts',(4.67528395050075,3.11242760942936,61.0254961162954));
#67679=CARTESIAN_POINT('Ctrl Pts',(-0.0790419206570804,5.61598059260596,
61.1842568785413));
#67680=CARTESIAN_POINT('Ctrl Pts',(-4.76102621166261,2.97961659506878,61.3430176407873));
#67681=CARTESIAN_POINT('Ctrl Pts',(-5.08557388631535,-2.38378352384928,
61.5017784030331));
#67682=CARTESIAN_POINT('Ctrl Pts',(-0.75564899933528,-5.56547214812468,
61.660539165279));
#67683=CARTESIAN_POINT('Ctrl Pts',(4.26586893343571,-3.65347066287608,61.8192999275249));
#67684=CARTESIAN_POINT('Ctrl Pts',(5.38313331566308,1.60229876975119,61.9780606897708));
#67685=CARTESIAN_POINT('Ctrl Pts',(1.5735896574475,5.39159542544895,62.1368214520167));
#67686=CARTESIAN_POINT('Ctrl Pts',(-3.67615132118597,4.24633925934925,62.2955822142625));
#67687=CARTESIAN_POINT('Ctrl Pts',(-5.56136632116585,-0.785296303028447,
62.4543429765086));
#67688=CARTESIAN_POINT('Ctrl Pts',(-2.3566489898686,-5.09820470168657,62.6131037387542));
#67689=CARTESIAN_POINT('Ctrl Pts',(3.00494548173707,-4.7450804306709,62.7718645010003));
#67690=CARTESIAN_POINT('Ctrl Pts',(5.61632206120212,-0.0491136091362308,
62.930625263246));
#67691=CARTESIAN_POINT('Ctrl Pts',(3.08746913746389,4.69180348767462,63.0893860254921));
#67692=CARTESIAN_POINT('Ctrl Pts',(-2.26712984885402,5.13863871956213,63.2481467877378));
#67693=CARTESIAN_POINT('Ctrl Pts',(-5.54678234711784,0.882434833542929,
63.4069075499838));
#67694=CARTESIAN_POINT('Ctrl Pts',(-3.74985021262651,-4.18140036645774,
63.5656683122296));
#67695=CARTESIAN_POINT('Ctrl Pts',(1.47905937712676,-5.41829022853902,63.7244290744757));
#67696=CARTESIAN_POINT('Ctrl Pts',(5.35428864647665,-1.69619536963139,63.8831898367214));
#67697=CARTESIAN_POINT('Ctrl Pts',(4.32910939769494,3.57830930252506,64.0419505989674));
#67698=CARTESIAN_POINT('Ctrl Pts',(-0.658203006225538,5.57783600012977,
64.2007113612132));
#67699=CARTESIAN_POINT('Ctrl Pts',(-5.04310791377582,2.47235681319663,64.3594721234592));
#67700=CARTESIAN_POINT('Ctrl Pts',(-4.81240641490144,-2.89589884829624,
64.518232885705));
#67701=CARTESIAN_POINT('Ctrl Pts',(-0.177243568241342,-5.61373942744627,
64.676993647951));
#67702=CARTESIAN_POINT('Ctrl Pts',(4.62013800604848,-3.19371420869404,64.8357544101967));
#67703=CARTESIAN_POINT('Ctrl Pts',(5.18902815324987,2.14929580712564,64.9945151724427));
#67704=CARTESIAN_POINT('Ctrl Pts',(1.00876123366836,5.52520464916871,65.1532759346885));
#67705=CARTESIAN_POINT('Ctrl Pts',(-4.09475477997962,3.84427742671915,65.3120366969346));
#67706=CARTESIAN_POINT('Ctrl Pts',(-5.45062614307688,-1.35504992164687,
65.4707974591803));
#67707=CARTESIAN_POINT('Ctrl Pts',(-1.81791796848671,-5.31419419118279,
65.6295582214263));
#67708=CARTESIAN_POINT('Ctrl Pts',(3.47860425988976,-4.40962561277309,65.7883189836721));
#67709=CARTESIAN_POINT('Ctrl Pts',(5.59140161426455,0.530767020214592,65.947079745918));
#67710=CARTESIAN_POINT('Ctrl Pts',(2.58677741967834,4.98538546381227,66.1058405081639));
#67711=CARTESIAN_POINT('Ctrl Pts',(-2.78534448354271,4.87722685034708,66.2646012704098));
#67712=CARTESIAN_POINT('Ctrl Pts',(-5.6082340359703,0.305281246610254,66.4233620326558));
#67713=CARTESIAN_POINT('Ctrl Pts',(-3.29829649293878,-4.54606707896127,
66.5821227949015));
#67714=CARTESIAN_POINT('Ctrl Pts',(2.03034274820855,-5.23671595244054,66.7408835571475));
#67715=CARTESIAN_POINT('Ctrl Pts',(5.50075028856868,-1.13456242867458,66.8996443193933));
#67716=CARTESIAN_POINT('Ctrl Pts',(3.93670314222528,4.00597728547496,67.0584050816393));
#67717=CARTESIAN_POINT('Ctrl Pts',(-1.23033496804577,5.48012422378831,67.2171658438851));
#67718=CARTESIAN_POINT('Ctrl Pts',(-5.27133293449043,1.93869407991674,67.375926606131));
#67719=CARTESIAN_POINT('Ctrl Pts',(-4.48784598432852,-3.37708810407645,
67.534687368377));
#67720=CARTESIAN_POINT('Ctrl Pts',(0.403054693731489,-5.60205610071956,
67.6934481306228));
#67721=CARTESIAN_POINT('Ctrl Pts',(4.92506740462245,-2.69985123695237,67.8522088928687));
#67722=CARTESIAN_POINT('Ctrl Pts',(4.93950798866025,2.67333994690335,68.0109696551146));
#67723=CARTESIAN_POINT('Ctrl Pts',(0.433159982240225,5.59980875312125,68.1697304173605));
#67724=CARTESIAN_POINT('Ctrl Pts',(-4.46962927096998,3.40116154009715,68.3284911796064));
#67725=CARTESIAN_POINT('Ctrl Pts',(-5.28167728878481,-1.91033260425587,
68.4872519418522));
#67726=CARTESIAN_POINT('Ctrl Pts',(-1.25977292097022,-5.47343199732475,
68.6460127040982));
#67727=CARTESIAN_POINT('Ctrl Pts',(3.9151141043812,-4.02707923828464,68.804773466344));
#67728=CARTESIAN_POINT('Ctrl Pts',(5.50676911268545,1.10497944837047,68.96353422859));
#67729=CARTESIAN_POINT('Ctrl Pts',(2.05846082260739,5.22572719184021,69.1222949908358));
#67730=CARTESIAN_POINT('Ctrl Pts',(-3.27381368882556,4.56372978742243,69.2810557530818));
#67731=CARTESIAN_POINT('Ctrl Pts',(-5.60979391230414,-0.27513251938597,
69.4398165153275));
#67732=CARTESIAN_POINT('Ctrl Pts',(-2.81151939385567,-4.86218514042,69.5985772775736));
#67733=CARTESIAN_POINT('Ctrl Pts',(2.55994355282749,-4.99921740356275,69.7573380398193));
#67734=CARTESIAN_POINT('Ctrl Pts',(5.58846796546901,-0.560813195881055,
69.9160988020653));
#67735=CARTESIAN_POINT('Ctrl Pts',(3.50225579413674,4.39086437893307,70.074859564311));
#67736=CARTESIAN_POINT('Ctrl Pts',(-1.78932785778569,5.32388875344897,70.2336203265571));
#67737=CARTESIAN_POINT('Ctrl Pts',(-5.4432639985316,1.38432752050883,70.3923810888029));
#67738=CARTESIAN_POINT('Ctrl Pts',(-4.11535866115752,-3.82221254403565,
70.5511418510488));
#67739=CARTESIAN_POINT('Ctrl Pts',(0.979048628174891,-5.53054693727633,
70.7099026132948));
#67740=CARTESIAN_POINT('Ctrl Pts',(5.17740070757192,-2.17715584076599,70.8686633755405));
#67741=CARTESIAN_POINT('Ctrl Pts',(4.63723751363544,3.16883478330451,71.0274241377865));
#67742=CARTESIAN_POINT('Ctrl Pts',(-0.14706709904452,5.61461102037593,71.1861849000324));
#67743=CARTESIAN_POINT('Ctrl Pts',(-4.79677141045583,2.92172375107252,71.3449456622783));
#67744=CARTESIAN_POINT('Ctrl Pts',(-5.05632400772744,-2.44521434042637,
71.5037064245242));
#67745=CARTESIAN_POINT('Ctrl Pts',(-0.688174425699173,-5.57421757752254,
71.6624671867701));
#67746=CARTESIAN_POINT('Ctrl Pts',(4.30981341129062,-3.60152662097726,71.8212279490159));
#67747=CARTESIAN_POINT('Ctrl Pts',(5.36332836930242,1.66739150914959,71.9799887112618));
#67748=CARTESIAN_POINT('Ctrl Pts',(1.50816137873041,5.41026199896583,72.1387494735078));
#67749=CARTESIAN_POINT('Ctrl Pts',(-3.72732097304471,4.20149544872403,72.2975102357535));
#67750=CARTESIAN_POINT('Ctrl Pts',(-5.55144531778782,-0.85260807253943,
72.4562709979996));
#67751=CARTESIAN_POINT('Ctrl Pts',(-2.29471733658639,-5.12637864256223,
72.6150317602453));
#67752=CARTESIAN_POINT('Ctrl Pts',(3.06220604411272,-4.70833089163749,72.7737925224914));
#67753=CARTESIAN_POINT('Ctrl Pts',(5.61650491693822,0.0189251091536447,
72.9325532847371));
#67754=CARTESIAN_POINT('Ctrl Pts',(3.03040693140542,4.72886027197227,73.0913140469831));
#67755=CARTESIAN_POINT('Ctrl Pts',(-2.32921204273454,5.11079806896419,73.2500748092289));
#67756=CARTESIAN_POINT('Ctrl Pts',(-5.55706500865567,0.815177361880478,
73.4088355714748));
#67757=CARTESIAN_POINT('Ctrl Pts',(-3.69892233589434,-4.22651856671307,
73.5675963337208));
#67758=CARTESIAN_POINT('Ctrl Pts',(1.54458704373152,-5.39997560236016,73.7263570959665));
#67759=CARTESIAN_POINT('Ctrl Pts',(5.37444318090863,-1.63121002232468,73.8851178582126));
#67760=CARTESIAN_POINT('Ctrl Pts',(4.28544475441368,3.63048879610115,74.0438786204583));
#67761=CARTESIAN_POINT('Ctrl Pts',(-0.725723611935015,5.56945337361106,
74.2026393827042));
#67762=CARTESIAN_POINT('Ctrl Pts',(-5.07268756112454,2.41108410242379,74.3614001449502));
#67763=CARTESIAN_POINT('Ctrl Pts',(-4.77697290711372,-2.9539829868247,74.5201609071961));
#67764=CARTESIAN_POINT('Ctrl Pts',(-0.109226733975009,-5.61547461594591,
74.6789216694419));
#67765=CARTESIAN_POINT('Ctrl Pts',(4.65848708247156,-3.13751234964793,74.8376824316879));
#67766=CARTESIAN_POINT('Ctrl Pts',(5.16261122569953,2.21199705561036,74.9964431939337));
#67767=CARTESIAN_POINT('Ctrl Pts',(0.94175588115421,5.53701918924425,75.1552039561797));
#67768=CARTESIAN_POINT('Ctrl Pts',(-4.14102321213148,3.79439223042856,75.3139647184255));
#67769=CARTESIAN_POINT('Ctrl Pts',(-5.43381137247341,-1.42097839889528,
75.4727254806715));
#67770=CARTESIAN_POINT('Ctrl Pts',(-1.75340938679805,-5.33582619319972,
75.6314862429172));
#67771=CARTESIAN_POINT('Ctrl Pts',(3.53176642826186,-4.36716287055454,75.7902470051633));
#67772=CARTESIAN_POINT('Ctrl Pts',(5.58456172896637,0.598461307948863,75.949007767409));
#67773=CARTESIAN_POINT('Ctrl Pts',(2.52619555266178,5.0163554171789,76.107768529655));
#67774=CARTESIAN_POINT('Ctrl Pts',(-2.84422195708685,4.8431278220354,76.2665292919008));
#67775=CARTESIAN_POINT('Ctrl Pts',(-5.61152065381861,0.23732170889948,76.4252900541468));
#67776=CARTESIAN_POINT('Ctrl Pts',(-3.24298424204541,-4.58568848130712,
76.5840508163926));
#67777=CARTESIAN_POINT('Ctrl Pts',(2.09363040629115,-5.21173650174305,76.7428115786384));
#67778=CARTESIAN_POINT('Ctrl Pts',(5.51409055601673,-1.06784408121947,76.9015723408844));
#67779=CARTESIAN_POINT('Ctrl Pts',(3.88788659878658,4.05337186015841,77.0603331031303));
#67780=CARTESIAN_POINT('Ctrl Pts',(-1.29662993069554,5.46481806326361,77.2190938653762));
#67781=CARTESIAN_POINT('Ctrl Pts',(-5.29443114152808,1.8746958498288,77.377854627622));
#67782=CARTESIAN_POINT('Ctrl Pts',(-4.44660725112929,-3.43120526869962,
77.5366153898679));
#67783=CARTESIAN_POINT('Ctrl Pts',(0.470887418890042,-5.59676251778467,
77.6953761521139));
#67784=CARTESIAN_POINT('Ctrl Pts',(4.95741153969778,-2.63999175525599,77.8541369143597));
#67785=CARTESIAN_POINT('Ctrl Pts',(4.90676119326682,2.73298010128111,78.0128976766056));
#67786=CARTESIAN_POINT('Ctrl Pts',(0.365293123785983,5.60464508916152,78.1716584388516));
#67787=CARTESIAN_POINT('Ctrl Pts',(-4.51050237060752,3.34676769532807,78.3304192010974));
#67788=CARTESIAN_POINT('Ctrl Pts',(-5.25814832033228,-1.9741737216199,78.4891799633432));
#67789=CARTESIAN_POINT('Ctrl Pts',(-1.19337631505721,-5.48829104661996,
78.6479407255893));
#67790=CARTESIAN_POINT('Ctrl Pts',(3.96361014591247,-3.97935676372049,78.806701487835));
#67791=CARTESIAN_POINT('Ctrl Pts',(5.49297953129461,1.17160638037103,78.9654622500811));
#67792=CARTESIAN_POINT('Ctrl Pts',(1.99500626439154,5.25027957796405,79.1242230123267));
#67793=CARTESIAN_POINT('Ctrl Pts',(-3.32885767394246,4.52373653392658,79.2829837745728));
#67794=CARTESIAN_POINT('Ctrl Pts',(-5.60604938780277,-0.34306836529208,
79.4417445368186));
#67795=CARTESIAN_POINT('Ctrl Pts',(-2.75241346293775,-4.89588661743591,
79.6005052990645));
#67796=CARTESIAN_POINT('Ctrl Pts',(2.62031533677199,-4.96783989049817,79.7592660613105));
#67797=CARTESIAN_POINT('Ctrl Pts',(5.59485150169351,-0.493074351131619,
79.9180268235562));
#67798=CARTESIAN_POINT('Ctrl Pts',(3.44880867530152,4.43296789554331,80.0767875858023));
#67799=CARTESIAN_POINT('Ctrl Pts',(-1.85368919596017,5.30182251744854,80.235548348048));
#67800=CARTESIAN_POINT('Ctrl Pts',(-5.45963409340325,1.31828722510949,80.3943091102941));
#67801=CARTESIAN_POINT('Ctrl Pts',(-4.06875510187306,-3.87178480326137,
80.5530698725397));
#67802=CARTESIAN_POINT('Ctrl Pts',(1.04597284064243,-5.51828111447312,80.7118306347859));
#67803=CARTESIAN_POINT('Ctrl Pts',(5.20339448972971,-2.11427799164205,80.8705913970315));
#67804=CARTESIAN_POINT('Ctrl Pts',(4.59851056209243,3.2247769306293,81.0293521592777));
#67805=CARTESIAN_POINT('Ctrl Pts',(-0.215070695363695,5.6124175038425,81.1881129215234));
#67806=CARTESIAN_POINT('Ctrl Pts',(-4.8318126828924,2.86340214411448,81.3468736837694));
#67807=CARTESIAN_POINT('Ctrl Pts',(-5.02633211360974,-2.50628632185673,
81.5056344460153));
#67808=CARTESIAN_POINT('Ctrl Pts',(-0.62059886223198,-5.58214499018382,
81.664395208261));
#67809=CARTESIAN_POINT('Ctrl Pts',(4.35312542352183,-3.54905405536124,81.823155970507));
#67810=CARTESIAN_POINT('Ctrl Pts',(5.34273635521072,1.73223955954653,81.9819167327528));
#67811=CARTESIAN_POINT('Ctrl Pts',(1.44251177575087,5.42813461502377,82.1406774949988));
#67812=CARTESIAN_POINT('Ctrl Pts',(-3.77794363750813,4.15603507125568,82.2994382572446));
#67813=CARTESIAN_POINT('Ctrl Pts',(-5.54070964539341,-0.919794726960242,
82.4581990194906));
#67814=CARTESIAN_POINT('Ctrl Pts',(-2.23244892259243,-5.15380027738969,
82.6169597817364));
#67815=CARTESIAN_POINT('Ctrl Pts',(3.11901720681907,-4.6708904238858,82.7757205439823));
#67816=CARTESIAN_POINT('Ctrl Pts',(5.61586359044797,0.0869610864393738,
82.9344813062282));
#67817=CARTESIAN_POINT('Ctrl Pts',(2.97289993650437,4.765223026495,83.0932420684742));
#67818=CARTESIAN_POINT('Ctrl Pts',(-2.39095227805809,5.08220754164499,83.2520028307198));
#67819=CARTESIAN_POINT('Ctrl Pts',(-5.56653245165825,0.747800008209614,
83.4107635929661));
#67820=CARTESIAN_POINT('Ctrl Pts',(-3.64745110432035,-4.27101603744643,
83.5695243552116));
#67821=CARTESIAN_POINT('Ctrl Pts',(1.60988701191321,-5.38086946399345,83.7282851174578));
#67822=CARTESIAN_POINT('Ctrl Pts',(5.39381098887153,-1.56598350543525,83.8870458797035));
#67823=CARTESIAN_POINT('Ctrl Pts',(4.24114744292764,3.68213208808317,84.0458066419495));
#67824=CARTESIAN_POINT('Ctrl Pts',(-0.793130479779808,5.56025999380927,
84.2045674041954));
#67825=CARTESIAN_POINT('Ctrl Pts',(-5.10153665384735,2.3494449931422,84.3633281664411));
#67826=CARTESIAN_POINT('Ctrl Pts',(-4.74081182862427,-3.01160955008047,
84.5220889286872));
#67827=CARTESIAN_POINT('Ctrl Pts',(-0.0412447201429887,-5.61643184914312,
84.680849690933));
#67828=CARTESIAN_POINT('Ctrl Pts',(4.6962499152168,-3.08076173742818,84.8396104531789));
#67829=CARTESIAN_POINT('Ctrl Pts',(5.13525015825041,2.27420453014635,84.9983712154247));
#67830=CARTESIAN_POINT('Ctrl Pts',(0.874969588857335,5.54834518648496,85.1571319776707));
#67831=CARTESIAN_POINT('Ctrl Pts',(-4.1873683648852,3.74332940771524,85.3158927399165));
#67832=CARTESIAN_POINT('Ctrl Pts',(-5.41488683153288,-1.48550727360877,
85.4746535021625));
#67833=CARTESIAN_POINT('Ctrl Pts',(-1.69117083731324,-5.35897524785026,
85.6334142644083));
#67834=CARTESIAN_POINT('Ctrl Pts',(3.58937574805651,-4.3194834039373,85.7921750266543));
#67835=CARTESIAN_POINT('Ctrl Pts',(5.23680883419176,-0.173451275228434,
85.9244756618591));
#67836=CARTESIAN_POINT('Ctrl Pts',(4.02828187061023,2.86869243836803,86.0303161700231));
#67837=CARTESIAN_POINT('Ctrl Pts',(2.79564340622479,3.92301449006468,86.083236424105));
#67838=CARTESIAN_POINT('Ctrl Pts',(2.08577545033815,4.26978275451652,86.109696551146));
#67839=CARTESIAN_POINT('Ctrl Pts',(2.64867169498355,-3.71434815979776,25.890303448854));
#67840=CARTESIAN_POINT('Ctrl Pts',(3.26619649360659,-3.27399620981999,25.916763575895));
#67841=CARTESIAN_POINT('Ctrl Pts',(4.26716101578614,-2.08115178444252,25.9696838299769));
#67842=CARTESIAN_POINT('Ctrl Pts',(4.93173808918078,0.990295704796579,26.0755243381408));
#67843=CARTESIAN_POINT('Ctrl Pts',(2.71768336588486,4.65659895971115,26.2078249733458));
#67844=CARTESIAN_POINT('Ctrl Pts',(-2.44680000302844,4.80802422056935,26.3665857355916));
#67845=CARTESIAN_POINT('Ctrl Pts',(-5.36205296397033,0.552597707469077,
26.5253464978375));
#67846=CARTESIAN_POINT('Ctrl Pts',(-3.3748453548303,-4.20532476806197,26.6841072600834));
#67847=CARTESIAN_POINT('Ctrl Pts',(1.70375316232487,-5.11609754516703,26.8428680223293));
#67848=CARTESIAN_POINT('Ctrl Pts',(5.22165294276351,-1.34357917457709,27.0016287845752));
#67849=CARTESIAN_POINT('Ctrl Pts',(3.96125258927572,3.65816328556149,27.1603895468211));
#67850=CARTESIAN_POINT('Ctrl Pts',(-0.924981032991848,5.31208345139673,
27.319150309067));
#67851=CARTESIAN_POINT('Ctrl Pts',(-4.96444853774918,2.10409702077966,27.4779110713129));
#67852=CARTESIAN_POINT('Ctrl Pts',(-4.46040303022669,-3.02955771462767,
27.6366718335588));
#67853=CARTESIAN_POINT('Ctrl Pts',(0.125992795951784,-5.39050292069155,
27.7954325958046));
#67854=CARTESIAN_POINT('Ctrl Pts',(4.59704837888827,-2.8178773262279,27.9541933580506));
#67855=CARTESIAN_POINT('Ctrl Pts',(4.86075937558651,2.33374633870135,28.1129541202964));
#67856=CARTESIAN_POINT('Ctrl Pts',(0.67574734249545,5.34945894155921,28.2717148825423));
#67857=CARTESIAN_POINT('Ctrl Pts',(-4.12772534408922,3.46918077578477,28.4304756447882));
#67858=CARTESIAN_POINT('Ctrl Pts',(-5.15337977793343,-1.58619627522226,
28.5892364070341));
#67859=CARTESIAN_POINT('Ctrl Pts',(-1.46250254869165,-5.18983873767588,
28.74799716928));
#67860=CARTESIAN_POINT('Ctrl Pts',(3.56690112283287,-4.04358189961183,28.9067579315259));
#67861=CARTESIAN_POINT('Ctrl Pts',(5.3317682282855,0.803484416727951,29.0655186937718));
#67862=CARTESIAN_POINT('Ctrl Pts',(2.2168380367468,4.91517735084379,29.2242794560177));
#67863=CARTESIAN_POINT('Ctrl Pts',(-2.92700996008437,4.52834978587781,29.3830402182635));
#67864=CARTESIAN_POINT('Ctrl Pts',(-5.39196907660498,-0.00296179645705061,
29.5418009805095));
#67865=CARTESIAN_POINT('Ctrl Pts',(-2.92203337252994,-4.5315626662565,29.7005617427553));
#67866=CARTESIAN_POINT('Ctrl Pts',(2.22223651734922,-4.91273895817748,29.8593225050013));
#67867=CARTESIAN_POINT('Ctrl Pts',(5.33264767340791,-0.797626497839672,
30.0180832672471));
#67868=CARTESIAN_POINT('Ctrl Pts',(3.56245678780991,4.04749809913968,30.176844029493));
#67869=CARTESIAN_POINT('Ctrl Pts',(-1.46820336502753,5.18822880230289,30.3356047917389));
#67870=CARTESIAN_POINT('Ctrl Pts',(-5.15511895218379,1.58053402963151,30.4943655539848));
#67871=CARTESIAN_POINT('Ctrl Pts',(-4.12391220870013,-3.47371376528387,
30.6531263162307));
#67872=CARTESIAN_POINT('Ctrl Pts',(0.681624954493375,-5.34871261609428,
30.8118870784765));
#67873=CARTESIAN_POINT('Ctrl Pts',(4.86331813894988,-2.32840630217865,30.9706478407225));
#67874=CARTESIAN_POINT('Ctrl Pts',(4.59395401058964,2.82292858162795,31.1294086029683));
#67875=CARTESIAN_POINT('Ctrl Pts',(0.120062847618306,5.39063300003123,31.2881693652142));
#67876=CARTESIAN_POINT('Ctrl Pts',(-4.46371350087791,3.02466543778803,31.4469301274601));
#67877=CARTESIAN_POINT('Ctrl Pts',(-4.96216290745751,-2.10956832273333,
31.605690889706));
#67878=CARTESIAN_POINT('Ctrl Pts',(-0.919089249897086,-5.31306071668268,
31.7644516519519));
#67879=CARTESIAN_POINT('Ctrl Pts',(3.96516296311825,-3.65387765317291,31.9232124141978));
#67880=CARTESIAN_POINT('Ctrl Pts',(5.22037691480677,1.34944584766767,32.0819731764437));
#67881=CARTESIAN_POINT('Ctrl Pts',(1.69774245557567,5.11771528936226,32.2407339386896));
#67882=CARTESIAN_POINT('Ctrl Pts',(-3.37871775721717,4.20209537558378,32.3994947009355));
#67883=CARTESIAN_POINT('Ctrl Pts',(-5.36287227432698,-0.559410580603594,
32.5582554631813));
#67884=CARTESIAN_POINT('Ctrl Pts',(-2.43876227490629,-4.80892688600382,
32.7170162254272));
#67885=CARTESIAN_POINT('Ctrl Pts',(2.71737745147233,-4.65716641474905,32.8757769876731));
#67886=CARTESIAN_POINT('Ctrl Pts',(5.38649033088843,-0.24302498571551,33.034537749919));
#67887=CARTESIAN_POINT('Ctrl Pts',(3.12572272698597,4.39354033353968,33.1932985121649));
#67888=CARTESIAN_POINT('Ctrl Pts',(-1.99580179309791,5.00900333710248,33.3520592744107));
#67889=CARTESIAN_POINT('Ctrl Pts',(-5.29070754957905,1.04007348454996,33.5108200366567));
#67890=CARTESIAN_POINT('Ctrl Pts',(-3.74339614991909,-3.88076339052093,
33.6695807989025));
#67891=CARTESIAN_POINT('Ctrl Pts',(1.22998574967103,-5.24980707112582,33.8283415611485));
#67892=CARTESIAN_POINT('Ctrl Pts',(5.07764712075832,-1.81406696279143,33.9871023233943));
#67893=CARTESIAN_POINT('Ctrl Pts',(4.2780907481768,3.28196264128657,34.1458630856403));
#67894=CARTESIAN_POINT('Ctrl Pts',(-0.436904953119544,5.37423978720491,
34.3046238478861));
#67895=CARTESIAN_POINT('Ctrl Pts',(-4.75203189588531,2.54784852158155,34.463384610132));
#67896=CARTESIAN_POINT('Ctrl Pts',(-4.71795409483259,-2.61041153603965,
34.6221453723779));
#67897=CARTESIAN_POINT('Ctrl Pts',(-0.36586059440485,-5.3795432198188,34.7809061346238));
#67898=CARTESIAN_POINT('Ctrl Pts',(4.32107969737961,-3.22515262853255,34.9396668968697));
#67899=CARTESIAN_POINT('Ctrl Pts',(5.05323586102427,1.88099616195643,35.0984276591155));
#67900=CARTESIAN_POINT('Ctrl Pts',(1.16051621156039,5.265599809247,35.2571884213615));
#67901=CARTESIAN_POINT('Ctrl Pts',(-3.79434332315281,3.83096567127432,35.4159491836074));
#67902=CARTESIAN_POINT('Ctrl Pts',(-5.27650394879067,-1.10988526741874,
35.5747099458532));
#67903=CARTESIAN_POINT('Ctrl Pts',(-1.92944698758358,-5.03493530748322,
35.7334707080991));
#67904=CARTESIAN_POINT('Ctrl Pts',(3.18349879238559,-4.3518587600376,35.892231470345));
#67905=CARTESIAN_POINT('Ctrl Pts',(5.38280923632674,0.314171853851074,36.0509922325909));
#67906=CARTESIAN_POINT('Ctrl Pts',(2.65560824713265,4.69266279059105,36.2097529948368));
#67907=CARTESIAN_POINT('Ctrl Pts',(-2.50208652644733,4.77628540213074,36.3685137570827));
#67908=CARTESIAN_POINT('Ctrl Pts',(-5.36979528379463,0.488505720103176,
36.5272745193286));
#67909=CARTESIAN_POINT('Ctrl Pts',(-3.32290337488047,-4.24636931856435,
36.6860352815745));
#67910=CARTESIAN_POINT('Ctrl Pts',(1.76521120212947,-5.09483744984206,36.8447960438204));
#67911=CARTESIAN_POINT('Ctrl Pts',(5.23775056787229,-1.28035472318811,37.0035568060662));
#67912=CARTESIAN_POINT('Ctrl Pts',(3.91654062472413,3.70594775507185,37.1623175683121));
#67913=CARTESIAN_POINT('Ctrl Pts',(-0.98920693046264,5.30045364824194,37.321078330558));
#67914=CARTESIAN_POINT('Ctrl Pts',(-4.98960208717089,2.04382245807619,37.4798390928039));
#67915=CARTESIAN_POINT('Ctrl Pts',(-4.42336100432008,-3.08337747509074,
37.6385998550498));
#67916=CARTESIAN_POINT('Ctrl Pts',(0.191275183005581,-5.38857616006331,
37.7973606172957));
#67917=CARTESIAN_POINT('Ctrl Pts',(4.63085048026802,-2.761985347144,37.9561213795416));
#67918=CARTESIAN_POINT('Ctrl Pts',(4.83212996681944,2.39245882142244,38.1148821417875));
#67919=CARTESIAN_POINT('Ctrl Pts',(0.610896508406062,5.35725159801683,38.2736429040334));
#67920=CARTESIAN_POINT('Ctrl Pts',(-4.16944809457737,3.41892407272547,38.4324036662793));
#67921=CARTESIAN_POINT('Ctrl Pts',(-5.13378644395327,-1.64850719631984,
38.5911644285251));
#67922=CARTESIAN_POINT('Ctrl Pts',(-1.39952662627435,-5.20717432498527,
38.7499251907711));
#67923=CARTESIAN_POINT('Ctrl Pts',(3.61562270886826,-4.00007645621339,38.9086859530169));
#67924=CARTESIAN_POINT('Ctrl Pts',(5.32164370022099,0.868013569211233,39.0674467152629));
#67925=CARTESIAN_POINT('Ctrl Pts',(2.15713382540813,4.94167106227405,39.2262074775087));
#67926=CARTESIAN_POINT('Ctrl Pts',(-2.98165081692889,4.49256025383564,39.3849682397546));
#67927=CARTESIAN_POINT('Ctrl Pts',(-5.39153755590251,-0.0682789259528612,
39.5437290020005));
#67928=CARTESIAN_POINT('Ctrl Pts',(-2.8669244370552,-4.56662714710238,39.7024897642464));
#67929=CARTESIAN_POINT('Ctrl Pts',(2.28158549793223,-4.88545871378134,39.8612505264922));
#67930=CARTESIAN_POINT('Ctrl Pts',(5.3419186932756,-0.732969237328121,40.0200112887382));
#67931=CARTESIAN_POINT('Ctrl Pts',(3.51316472950203,4.09035607396464,40.1787720509841));
#67932=CARTESIAN_POINT('Ctrl Pts',(-1.53094490572569,5.17006256481187,40.3375328132299));
#67933=CARTESIAN_POINT('Ctrl Pts',(-5.17388699991225,1.517969874726,40.4962935754758));
#67934=CARTESIAN_POINT('Ctrl Pts',(-4.08152967334293,-3.52341521170266,
40.6550543377217));
#67935=CARTESIAN_POINT('Ctrl Pts',(0.746368282217007,-5.34006307226206,
40.8138150999676));
#67936=CARTESIAN_POINT('Ctrl Pts',(4.89116718777592,-2.26932209473684,40.9725758622135));
#67937=CARTESIAN_POINT('Ctrl Pts',(4.55942048043523,2.87837178123751,41.1313366244594));
#67938=CARTESIAN_POINT('Ctrl Pts',(0.054752880088232,5.39169188201243,41.2900973867052));
#67939=CARTESIAN_POINT('Ctrl Pts',(-4.50002622856399,2.97037088099662,41.4488581489512));
#67940=CARTESIAN_POINT('Ctrl Pts',(-4.93624387774355,-2.16952428146721,
41.607618911197));
#67941=CARTESIAN_POINT('Ctrl Pts',(-0.854660350479725,-5.32380455255023,
41.766379673443));
#67942=CARTESIAN_POINT('Ctrl Pts',(4.00913443548347,-3.60557627941182,41.9251404356888));
#67943=CARTESIAN_POINT('Ctrl Pts',(5.20364692548634,1.41258553840574,42.0839011979347));
#67944=CARTESIAN_POINT('Ctrl Pts',(1.63562280181919,5.13790592348729,42.2426619601806));
#67945=CARTESIAN_POINT('Ctrl Pts',(-3.42937327082192,4.16085786801338,42.4014227224264));
#67946=CARTESIAN_POINT('Ctrl Pts',(-5.3557021744363,-0.62433440332485,42.5601834846724));
#67947=CARTESIAN_POINT('Ctrl Pts',(-2.38032885595355,-4.83811675819748,
42.7189442469182));
#67948=CARTESIAN_POINT('Ctrl Pts',(2.77359413958947,-4.62390687376719,42.8777050091642));
#67949=CARTESIAN_POINT('Ctrl Pts',(5.38903905804413,-0.177756179390683,
43.03646577141));
#67950=CARTESIAN_POINT('Ctrl Pts',(3.07227082023542,4.43108239999738,43.195226533656));
#67951=CARTESIAN_POINT('Ctrl Pts',(-2.05633351598682,4.9844590177336,43.3539872959018));
#67952=CARTESIAN_POINT('Ctrl Pts',(-5.30291860685286,0.975906490156919,
43.5127480581477));
#67953=CARTESIAN_POINT('Ctrl Pts',(-3.6961106089692,-3.92582546666328,43.6715088203936));
#67954=CARTESIAN_POINT('Ctrl Pts',(1.29349071741166,-5.23452204049296,43.8302695826395));
#67955=CARTESIAN_POINT('Ctrl Pts',(5.09924982902894,-1.75242415230585,43.9890303448854));
#67956=CARTESIAN_POINT('Ctrl Pts',(4.23801973850483,3.33354584856425,44.1477911071313));
#67957=CARTESIAN_POINT('Ctrl Pts',(-0.501975468697378,5.36855286434462,
44.3065518693772));
#67958=CARTESIAN_POINT('Ctrl Pts',(-4.78254739390742,2.4900963140943,44.4653126316231));
#67959=CARTESIAN_POINT('Ctrl Pts',(-4.68598585940108,-2.66737244379737,
44.624073393869));
#67960=CARTESIAN_POINT('Ctrl Pts',(-0.300666931069113,-5.38358046517354,
44.7828341561148));
#67961=CARTESIAN_POINT('Ctrl Pts',(4.35983155656832,-3.1725712012164,44.9415949183607));
#67962=CARTESIAN_POINT('Ctrl Pts',(5.03007903084552,1.94207213354316,45.1003556806066));
#67963=CARTESIAN_POINT('Ctrl Pts',(1.0966445303283,5.27927173031827,45.2591164428526));
#67964=CARTESIAN_POINT('Ctrl Pts',(-3.84047254178868,3.78472058205141,45.4178772050983));
#67965=CARTESIAN_POINT('Ctrl Pts',(-5.26267183489948,-1.17372244870432,
45.5766379673443));
#67966=CARTESIAN_POINT('Ctrl Pts',(-1.86831311430597,-5.05793884258687,
45.7353987295902));
#67967=CARTESIAN_POINT('Ctrl Pts',(3.23598283686748,-4.3129751109803,45.8941594918361));
#67968=CARTESIAN_POINT('Ctrl Pts',(5.37860845135706,0.379355183735526,46.052920254082));
#67969=CARTESIAN_POINT('Ctrl Pts',(2.59856731943033,4.72448802674167,46.2116810163278));
#67970=CARTESIAN_POINT('Ctrl Pts',(-2.55976199751136,4.745625116308,46.3704417785738));
#67971=CARTESIAN_POINT('Ctrl Pts',(-5.37531894538233,0.423421142422616,
46.5292025408196));
#67972=CARTESIAN_POINT('Ctrl Pts',(-3.27121980318429,-4.28631079457517,
46.6879633030656));
#67973=CARTESIAN_POINT('Ctrl Pts',(1.82679962359794,-5.07308016530974,46.8467240653114));
#67974=CARTESIAN_POINT('Ctrl Pts',(5.25287623454225,-1.21681160950152,47.0054848275573));
#67975=CARTESIAN_POINT('Ctrl Pts',(3.87136006443976,3.75312009931705,47.1642455898032));
#67976=CARTESIAN_POINT('Ctrl Pts',(-1.05334308887091,5.28808165269453,47.3230063520491));
#67977=CARTESIAN_POINT('Ctrl Pts',(-5.01399447246331,1.98322935096872,47.4817671142949));
#67978=CARTESIAN_POINT('Ctrl Pts',(-4.38568496040199,-3.13673503129295,
47.6405278765409));
#67979=CARTESIAN_POINT('Ctrl Pts',(0.256537389910642,-5.38586370009625,
47.7992886387868));
#67980=CARTESIAN_POINT('Ctrl Pts',(4.66396888494043,-2.70568539722266,47.9580494010326));
#67981=CARTESIAN_POINT('Ctrl Pts',(4.80279359368822,2.45081882742566,48.1168101632785));
#67982=CARTESIAN_POINT('Ctrl Pts',(0.545954902252042,5.3642587999782,48.2755709255244));
#67983=CARTESIAN_POINT('Ctrl Pts',(-4.21055839213486,3.36816526537215,48.4343316877703));
#67984=CARTESIAN_POINT('Ctrl Pts',(-5.11344003285917,-1.71057600205014,
48.5930924500163));
#67985=CARTESIAN_POINT('Ctrl Pts',(-1.33634516345125,-5.22374586217178,
48.751853212262));
#67986=CARTESIAN_POINT('Ctrl Pts',(3.66381361874176,-3.9559839478389,48.910613974508));
#67987=CARTESIAN_POINT('Ctrl Pts',(5.31073826441816,0.932415312659234,49.0693747367539));
#67988=CARTESIAN_POINT('Ctrl Pts',(2.09711303188655,4.96743959801509,49.2281354989997));
#67989=CARTESIAN_POINT('Ctrl Pts',(-3.03585410457926,4.45611143084931,49.3868962612457));
#67990=CARTESIAN_POINT('Ctrl Pts',(-5.39031483316305,-0.133586031525688,
49.5456570234915));
#67991=CARTESIAN_POINT('Ctrl Pts',(-2.81139477712564,-4.60102147740992,
49.7044177857375));
#67992=CARTESIAN_POINT('Ctrl Pts',(2.34059965410881,-4.85746152713764,49.8631785479833));
#67993=CARTESIAN_POINT('Ctrl Pts',(5.35040578735549,-0.668204414134744,
50.0219393102293));
#67994=CARTESIAN_POINT('Ctrl Pts',(3.46335711374174,4.13261378925387,50.180700072475));
#67995=CARTESIAN_POINT('Ctrl Pts',(-1.59346177998899,5.15113762038552,50.339460834721));
#67996=CARTESIAN_POINT('Ctrl Pts',(-5.19189577974993,1.45518295779302,50.4982215969668));
#67997=CARTESIAN_POINT('Ctrl Pts',(-4.03854817336226,-3.57259959691384,
50.6569823592128));
#67998=CARTESIAN_POINT('Ctrl Pts',(0.811002080346741,-5.33062987404959,
50.8157431214586));
#67999=CARTESIAN_POINT('Ctrl Pts',(4.91829845774134,-2.2099048642455,50.9745038837045));
#68000=CARTESIAN_POINT('Ctrl Pts',(4.5242178552285,2.93339257973907,51.1332646459504));
#68001=CARTESIAN_POINT('Ctrl Pts',(-0.0105651224232033,5.3919595331034,
51.2920254081963));
#68002=CARTESIAN_POINT('Ctrl Pts',(-4.53567857731733,2.91564042222309,51.4507861704422));
#68003=CARTESIAN_POINT('Ctrl Pts',(-4.90960045414457,-2.22916186247211,
51.6095469326881));
#68004=CARTESIAN_POINT('Ctrl Pts',(-0.790106029640123,-5.33376711999718,
51.7683076949339));
#68005=CARTESIAN_POINT('Ctrl Pts',(4.05251756729386,-3.55674578726275,51.92706845718));
#68006=CARTESIAN_POINT('Ctrl Pts',(5.18615330087962,1.47551793218919,52.0858292194257));
#68007=CARTESIAN_POINT('Ctrl Pts',(1.57326312038517,5.15734256981952,52.2445899816717));
#68008=CARTESIAN_POINT('Ctrl Pts',(-3.47952552383355,4.11900975447104,52.4033507439175));
#68009=CARTESIAN_POINT('Ctrl Pts',(-5.34774612514876,-0.689166604960497,
52.5621115061635));
#68010=CARTESIAN_POINT('Ctrl Pts',(-2.32154612369557,-4.86659663666414,
52.7208722684093));
#68011=CARTESIAN_POINT('Ctrl Pts',(2.82940380271352,-4.58996877436295,52.8796330306552));
#68012=CARTESIAN_POINT('Ctrl Pts',(5.39079694361469,-0.112461287343052,
53.0383937929012));
#68013=CARTESIAN_POINT('Ctrl Pts',(3.01836805768307,4.46797420502795,53.1971545551469));
#68014=CARTESIAN_POINT('Ctrl Pts',(-2.11656347189292,4.95918322890829,53.355915317393));
#68015=CARTESIAN_POINT('Ctrl Pts',(-5.31435146071946,0.911596281467614,
53.5146760796387));
#68016=CARTESIAN_POINT('Ctrl Pts',(-3.64828266371651,-3.97031142784319,
53.6734368418848));
#68017=CARTESIAN_POINT('Ctrl Pts',(1.35680586536473,-5.21846884365023,53.8321976041305));
#68018=CARTESIAN_POINT('Ctrl Pts',(5.1201042222894,-1.69052417354231,53.9909583663765));
#68019=CARTESIAN_POINT('Ctrl Pts',(4.19732679935496,3.38463985792481,54.1497191286223));
#68020=CARTESIAN_POINT('Ctrl Pts',(-0.56697231936563,5.36207810624853,54.3084798908682));
#68021=CARTESIAN_POINT('Ctrl Pts',(-4.81236105300778,2.43197868492519,54.4672406531142));
#68022=CARTESIAN_POINT('Ctrl Pts',(-4.65332995545485,-2.72394191459784,
54.6260014153599));
#68023=CARTESIAN_POINT('Ctrl Pts',(-0.235429144855458,-5.3868276699918,
54.784762177606));
#68024=CARTESIAN_POINT('Ctrl Pts',(4.39794361039255,-3.11952419901562,54.9435229398517));
#68025=CARTESIAN_POINT('Ctrl Pts',(5.00618403647253,2.002863106007,55.1022837020977));
#68026=CARTESIAN_POINT('Ctrl Pts',(1.03261191649043,5.29216891816187,55.2610444643436));
#68027=CARTESIAN_POINT('Ctrl Pts',(-3.88603817100542,3.73792008501059,55.4198052265894));
#68028=CARTESIAN_POINT('Ctrl Pts',(-5.24806742381559,-1.23738738619803,
55.5785659888354));
#68029=CARTESIAN_POINT('Ctrl Pts',(-1.80690506604304,-5.08020012506836,
55.7373267510812));
#68030=CARTESIAN_POINT('Ctrl Pts',(3.287992000806,-4.27345853274282,55.8960875133271));
#68031=CARTESIAN_POINT('Ctrl Pts',(5.37361835549403,0.444482843239534,56.054848275573));
#68032=CARTESIAN_POINT('Ctrl Pts',(2.54114505192401,4.7556199441838,56.2136090378189));
#68033=CARTESIAN_POINT('Ctrl Pts',(-2.61706182345312,4.71426840990844,56.3723698000648));
#68034=CARTESIAN_POINT('Ctrl Pts',(-5.38005377881171,0.358274427681354,
56.5311305623107));
#68035=CARTESIAN_POINT('Ctrl Pts',(-3.21905617991939,-4.32562325439461,
56.6898913245565));
#68036=CARTESIAN_POINT('Ctrl Pts',(1.88811996218651,-5.05057840616592,56.8486520868024));
#68037=CARTESIAN_POINT('Ctrl Pts',(5.26723104152409,-1.15308992868801,57.0074128490484));
#68038=CARTESIAN_POINT('Ctrl Pts',(3.82561138199176,3.79974167311562,57.1661736112942));
#68039=CARTESIAN_POINT('Ctrl Pts',(-1.11732466916059,5.27493363106322,57.3249343735401));
#68040=CARTESIAN_POINT('Ctrl Pts',(-5.03765105397079,1.92234520491603,57.4836951357861));
#68041=CARTESIAN_POINT('Ctrl Pts',(-4.34736531713187,-3.18963227156913,
57.6424558980318));
#68042=CARTESIAN_POINT('Ctrl Pts',(0.321761949948743,-5.38236086452793,
57.8012166602778));
#68043=CARTESIAN_POINT('Ctrl Pts',(4.69640285208957,-2.64898838791747,57.9599774225237));
#68044=CARTESIAN_POINT('Ctrl Pts',(4.77275241050502,2.50881917571891,58.1187381847696));
#68045=CARTESIAN_POINT('Ctrl Pts',(0.480933177205712,5.37047879685782,58.2774989470154));
#68046=CARTESIAN_POINT('Ctrl Pts',(-4.25105079016747,3.31691217970165,58.4362597092614));
#68047=CARTESIAN_POINT('Ctrl Pts',(-5.09234322434225,-1.77239378071924,
58.5950204715072));
#68048=CARTESIAN_POINT('Ctrl Pts',(-1.27296759194985,-5.23955081455291,
58.7537812337532));
#68049=CARTESIAN_POINT('Ctrl Pts',(3.71146686389641,-3.91131089874422,58.912541995999));
#68050=CARTESIAN_POINT('Ctrl Pts',(5.29905347767321,0.996680224142156,59.071302758245));
#68051=CARTESIAN_POINT('Ctrl Pts',(2.03678448698746,4.99247916189982,59.2300635204907));
#68052=CARTESIAN_POINT('Ctrl Pts',(-3.08961188058148,4.41900867342512,59.3888242827367));
#68053=CARTESIAN_POINT('Ctrl Pts',(-5.38830108161851,-0.198873533345728,
59.5475850449826));
#68054=CARTESIAN_POINT('Ctrl Pts',(-2.7554525449587,-4.63474060772737,59.7063458072284));
#68055=CARTESIAN_POINT('Ctrl Pts',(2.39927032724118,-4.82875150792175,59.8651065694744));
#68056=CARTESIAN_POINT('Ctrl Pts',(5.35810770928357,-0.603341531930828,
60.0238673317202));
#68057=CARTESIAN_POINT('Ctrl Pts',(3.4130412502586,4.17426504339022,60.1826280939662));
#68058=CARTESIAN_POINT('Ctrl Pts',(-1.65574481370544,5.13145674641463,60.341388856212));
#68059=CARTESIAN_POINT('Ctrl Pts',(-5.20914264878242,1.39218249273314,60.500149618458));
#68060=CARTESIAN_POINT('Ctrl Pts',(-3.99497401635973,-3.62125970306563,
60.6589103807038));
#68061=CARTESIAN_POINT('Ctrl Pts',(0.875516863905577,-5.32041440580089,
60.8176711429497));
#68062=CARTESIAN_POINT('Ctrl Pts',(4.94470796731371,-2.15016333017309,60.9764319051956));
#68063=CARTESIAN_POINT('Ctrl Pts',(4.48835130096483,2.98798290282324,61.1351926674415));
#68064=CARTESIAN_POINT('Ctrl Pts',(-0.0758815745026817,5.39143591402955,
61.2939534296874));
#68065=CARTESIAN_POINT('Ctrl Pts',(-4.57066531515243,2.86048209316173,61.4527141919332));
#68066=CARTESIAN_POINT('Ctrl Pts',(-4.88223654658481,-2.2884723139309,61.6114749541792));
#68067=CARTESIAN_POINT('Ctrl Pts',(-0.725435760725668,-5.34294695701698,
61.770235716425));
#68068=CARTESIAN_POINT('Ctrl Pts',(4.09530599207347,-3.50739334260129,61.9289964786709));
#68069=CARTESIAN_POINT('Ctrl Pts',(5.16789860817661,1.53823379368774,62.0877572409168));
#68070=CARTESIAN_POINT('Ctrl Pts',(1.51067256255815,5.17602237603069,62.2465180031627));
#68071=CARTESIAN_POINT('Ctrl Pts',(-3.52916715640777,4.07655717616831,62.4052787654086));
#68072=CARTESIAN_POINT('Ctrl Pts',(-5.33900529401489,-0.75389767138361,
62.5640395276545));
#68073=CARTESIAN_POINT('Ctrl Pts',(-2.26242270449944,-4.89436234198102,
62.7228002899004));
#68074=CARTESIAN_POINT('Ctrl Pts',(2.88479825077521,-4.5553570969531,62.8815610521463));
#68075=CARTESIAN_POINT('Ctrl Pts',(5.39176372963048,-0.0471498915993996,
63.0403218143921));
#68076=CARTESIAN_POINT('Ctrl Pts',(2.96402234956039,4.50421033475823,63.1990825766381));
#68077=CARTESIAN_POINT('Ctrl Pts',(-2.17648282206887,4.93317967984907,63.3578433388838));
#68078=CARTESIAN_POINT('Ctrl Pts',(-5.32500443340729,0.847152296006667,
63.5166041011299));
#68079=CARTESIAN_POINT('Ctrl Pts',(-3.59991933291304,-4.01421474574488,
63.6753648633757));
#68080=CARTESIAN_POINT('Ctrl Pts',(1.41992190203103,-5.20164983640472,63.8341256256216));
#68081=CARTESIAN_POINT('Ctrl Pts',(5.14020724015703,-1.62837611032391,63.9928863878675));
#68082=CARTESIAN_POINT('Ctrl Pts',(4.15601790241685,3.43523717132127,64.1516471501133));
#68083=CARTESIAN_POINT('Ctrl Pts',(-0.631885966835028,5.35481646308756,
64.3104079123593));
#68084=CARTESIAN_POINT('Ctrl Pts',(-4.84146849803133,2.3735041628375,64.4691686746051));
#68085=CARTESIAN_POINT('Ctrl Pts',(-4.61999117524849,-2.7801116468701,64.6279294368511));
#68086=CARTESIAN_POINT('Ctrl Pts',(-0.170156809410319,-5.38928435774618,
64.7866901990969));
#68087=CARTESIAN_POINT('Ctrl Pts',(4.43541026590754,-3.06601940657889,64.9454509613428));
#68088=CARTESIAN_POINT('Ctrl Pts',(4.98155438449627,2.06336015827155,65.1042117235887));
#68089=CARTESIAN_POINT('Ctrl Pts',(0.968427766834154,5.30428948011521,65.2629724858346));
#68090=CARTESIAN_POINT('Ctrl Pts',(-3.93103352404596,3.69057104812572,65.4217332480805));
#68091=CARTESIAN_POINT('Ctrl Pts',(-5.23269285873673,-1.30087073706907,
65.5804940103263));
#68092=CARTESIAN_POINT('Ctrl Pts',(-1.74523185442701,-5.10171588808409,
65.7392547725724));
#68093=CARTESIAN_POINT('Ctrl Pts',(3.33951865185531,-4.23331482438371,65.8980155348181));
#68094=CARTESIAN_POINT('Ctrl Pts',(5.36783968103429,0.50954527487755,66.0567762970641));
#68095=CARTESIAN_POINT('Ctrl Pts',(2.48334987133277,4.78605397430791,66.2155370593099));
#68096=CARTESIAN_POINT('Ctrl Pts',(-2.67397759552212,4.68221988452942,66.3742978215559));
#68097=CARTESIAN_POINT('Ctrl Pts',(-5.38399908924589,0.29307513616095,66.5330585838017));
#68098=CARTESIAN_POINT('Ctrl Pts',(-3.16642016009836,-4.36430092891852,
66.6918193460477));
#68099=CARTESIAN_POINT('Ctrl Pts',(1.94916321913439,-5.0273354745442,66.8505801082934));
#68100=CARTESIAN_POINT('Ctrl Pts',(5.2808128822496,-1.08919903190536,67.0093408705395));
#68101=CARTESIAN_POINT('Ctrl Pts',(3.77930129100008,3.84580563475087,67.1681016327852));
#68102=CARTESIAN_POINT('Ctrl Pts',(-1.18114228203367,5.26101151282039,67.3268623950312));
#68103=CARTESIAN_POINT('Ctrl Pts',(-5.06056836008944,1.86117895466771,67.485623157277));
#68104=CARTESIAN_POINT('Ctrl Pts',(-4.30840769791819,-3.24206143324834,
67.644383919523));
#68105=CARTESIAN_POINT('Ctrl Pts',(0.386939291414611,-5.37806816739956,
67.8031446817688));
#68106=CARTESIAN_POINT('Ctrl Pts',(4.72814762203013,-2.59190263951545,67.9619054440148));
#68107=CARTESIAN_POINT('Ctrl Pts',(4.74201082581408,2.56645135475007,68.1206662062606));
#68108=CARTESIAN_POINT('Ctrl Pts',(0.415840875206383,5.37591067587102,68.2794269685066));
#68109=CARTESIAN_POINT('Ctrl Pts',(-4.29091934641509,3.26517233710519,68.4381877307524));
#68110=CARTESIAN_POINT('Ctrl Pts',(-5.07049911435956,-1.83395146056701,
68.5969484929983));
#68111=CARTESIAN_POINT('Ctrl Pts',(-1.20940321242992,-5.25458686275155,
68.7557092552442));
#68112=CARTESIAN_POINT('Ctrl Pts',(3.75857545121767,-3.86606386470014,68.9144700174901));
#68113=CARTESIAN_POINT('Ctrl Pts',(5.28659105472879,1.06079887278309,69.073230779736));
#68114=CARTESIAN_POINT('Ctrl Pts',(1.97615704392586,5.01678607937179,69.2319915419818));
#68115=CARTESIAN_POINT('Ctrl Pts',(-3.14291625598096,4.38125742639343,69.3907523042277));
#68116=CARTESIAN_POINT('Ctrl Pts',(-5.38549659678694,-0.264131850470941,
69.5495130664737));
#68117=CARTESIAN_POINT('Ctrl Pts',(-2.69910595007792,-4.66777958977181,
69.7082738287194));
#68118=CARTESIAN_POINT('Ctrl Pts',(2.45758890740704,-4.79933286932947,69.8670345909655));
#68119=CARTESIAN_POINT('Ctrl Pts',(5.36502332880251,-0.538390109345589,
70.0257953532112));
#68120=CARTESIAN_POINT('Ctrl Pts',(3.36222452290666,4.21530372405138,70.1845561154571));
#68121=CARTESIAN_POINT('Ctrl Pts',(-1.7177848668387,5.11102283106786,70.3433168777031));
#68122=CARTESIAN_POINT('Ctrl Pts',(-5.22562507603134,1.32897772486576,70.5020776399489));
#68123=CARTESIAN_POINT('Ctrl Pts',(-3.95081359684368,-3.66938838928662,
70.6608384021949));
#68124=CARTESIAN_POINT('Ctrl Pts',(0.939903165347853,-5.3094181666361,70.8195991644408));
#68125=CARTESIAN_POINT('Ctrl Pts',(4.97039184089704,-2.09010625959075,70.9783599266866));
#68126=CARTESIAN_POINT('Ctrl Pts',(4.45182608106173,3.0421347393591,71.1371206889325));
#68127=CARTESIAN_POINT('Ctrl Pts',(-0.141186890959645,5.39012110163196,
71.2958814511784));
#68128=CARTESIAN_POINT('Ctrl Pts',(-4.60498130776496,2.80490398829831,71.4546422134243));
#68129=CARTESIAN_POINT('Ctrl Pts',(-4.85415617071822,-2.34744693203373,
71.6134029756702));
#68130=CARTESIAN_POINT('Ctrl Pts',(-0.660659034099426,-5.35134271646838,
71.7721637379161));
#68131=CARTESIAN_POINT('Ctrl Pts',(4.13749343062021,-3.4575261878996,71.9309245001619));
#68132=CARTESIAN_POINT('Ctrl Pts',(5.14888552625377,1.60072391934755,72.0896852624079));
#68133=CARTESIAN_POINT('Ctrl Pts',(1.44786031350356,5.19394260085899,72.2484460246537));
#68134=CARTESIAN_POINT('Ctrl Pts',(-3.57829088363412,4.03350636302179,72.4072067868997));
#68135=CARTESIAN_POINT('Ctrl Pts',(-5.32948096375172,-0.818518103308924,
72.5659675491455));
#68136=CARTESIAN_POINT('Ctrl Pts',(-2.20296727472809,-4.92140979953042,
72.7247283113914));
#68137=CARTESIAN_POINT('Ctrl Pts',(2.93976935463837,-4.52007692080191,72.8834890736374));
#68138=CARTESIAN_POINT('Ctrl Pts',(5.39193927421552,0.0181684233918482,
73.0422498358832));
#68139=CARTESIAN_POINT('Ctrl Pts',(2.90924167110106,4.53978547153557,73.201010598129));
#68140=CARTESIAN_POINT('Ctrl Pts',(-2.23608277334895,4.90645218657722,73.359771360375));
#68141=CARTESIAN_POINT('Ctrl Pts',(-5.33487596159239,0.782583990930051,
73.5185321226207));
#68142=CARTESIAN_POINT('Ctrl Pts',(-3.5510277138785,-4.05752897755565,73.6772928848669));
#68143=CARTESIAN_POINT('Ctrl Pts',(1.48282956513097,-5.18406748694598,73.8360536471125));
#68144=CARTESIAN_POINT('Ctrl Pts',(5.15955593251365,-1.56598908288006,73.9948144093587));
#68145=CARTESIAN_POINT('Ctrl Pts',(4.11409910977184,3.48533036359696,74.1535751716043));
#68146=CARTESIAN_POINT('Ctrl Pts',(-0.696706885026663,5.34676900050795,
74.3123359338504));
#68147=CARTESIAN_POINT('Ctrl Pts',(-4.86986545745996,2.31468132896846,74.4710966960961));
#68148=CARTESIAN_POINT('Ctrl Pts',(-4.58597441124858,-2.83587339770487,
74.6298574583422));
#68149=CARTESIAN_POINT('Ctrl Pts',(-0.104859503450096,-5.39095016791776,
74.7886182205879));
#68150=CARTESIAN_POINT('Ctrl Pts',(4.47222602488106,-3.01206467573539,74.9473789828339));
#68151=CARTESIAN_POINT('Ctrl Pts',(4.95619368931852,2.12355441239345,75.1061397450797));
#68152=CARTESIAN_POINT('Ctrl Pts',(0.904101500384337,5.31563163748572,75.2649005073256));
#68153=CARTESIAN_POINT('Ctrl Pts',(-3.97545199784159,3.64268041986863,75.4236612695716));
#68154=CARTESIAN_POINT('Ctrl Pts',(-5.21655039588045,-1.36416318513457,
75.5824220318174));
#68155=CARTESIAN_POINT('Ctrl Pts',(-1.68330253000285,-5.12248297419546,
75.7411827940633));
#68156=CARTESIAN_POINT('Ctrl Pts',(3.39055522847852,-4.19254987699292,75.8999435563093));
#68157=CARTESIAN_POINT('Ctrl Pts',(5.36127327599845,0.574532930736923,76.058704318555));
#68158=CARTESIAN_POINT('Ctrl Pts',(2.42519025910013,4.81578565091957,76.217465080801));
#68159=CARTESIAN_POINT('Ctrl Pts',(-2.73050096132775,4.64948424329249,76.3762258430469));
#68160=CARTESIAN_POINT('Ctrl Pts',(-5.38715429771053,0.227832835858649,
76.5349866052928));
#68161=CARTESIAN_POINT('Ctrl Pts',(-3.11331946805805,-4.40233814219751,
76.6937473675387));
#68162=CARTESIAN_POINT('Ctrl Pts',(2.00992043634247,-5.00335478134514,76.8525081297845));
#68163=CARTESIAN_POINT('Ctrl Pts',(5.29361976358337,-1.02514829514396,77.0112688920305));
#68164=CARTESIAN_POINT('Ctrl Pts',(3.73243658747159,3.89130522433545,77.1700296542762));
#68165=CARTESIAN_POINT('Ctrl Pts',(-1.24478656225425,5.2463173410372,77.3287904165223));
#68166=CARTESIAN_POINT('Ctrl Pts',(-5.0827430277043,1.79973957637201,77.4875511787681));
#68167=CARTESIAN_POINT('Ctrl Pts',(-4.26881781979216,-3.29401482234996,
77.646311941014));
#68168=CARTESIAN_POINT('Ctrl Pts',(0.452059849531884,-5.3729862386645,77.8050727032599));
#68169=CARTESIAN_POINT('Ctrl Pts',(4.75919853621651,-2.53443652935156,77.9638334655057));
#68170=CARTESIAN_POINT('Ctrl Pts',(4.71057335094352,2.62370690699572,78.1225942277518));
#68171=CARTESIAN_POINT('Ctrl Pts',(0.350687548550617,5.38055363988948,78.2813549899974));
#68172=CARTESIAN_POINT('Ctrl Pts',(-4.33015821016646,3.21295333040559,78.4401157522436));
#68173=CARTESIAN_POINT('Ctrl Pts',(-5.04791090853454,-1.89524000800277,
78.5988765144892));
#68174=CARTESIAN_POINT('Ctrl Pts',(-1.14566135296546,-5.26885180022729,
78.7576372767353));
#68175=CARTESIAN_POINT('Ctrl Pts',(3.80513246751939,-3.82024948570991,78.916398038981));
#68176=CARTESIAN_POINT('Ctrl Pts',(5.27335282444574,1.12476184916915,79.0751588012271));
#68177=CARTESIAN_POINT('Ctrl Pts',(1.91523959978009,5.0403567833905,79.2339195634728));
#68178=CARTESIAN_POINT('Ctrl Pts',(-3.19575940835959,4.34286322975033,79.3926803257188));
#68179=CARTESIAN_POINT('Ctrl Pts',(-5.3819017902265,-0.329351406241924,
79.5514410879647));
#68180=CARTESIAN_POINT('Ctrl Pts',(-2.64236326134738,-4.70013357507201,
79.7102018502106));
#68181=CARTESIAN_POINT('Ctrl Pts',(2.51554683635375,-4.76920992854652,79.8689626124565));
#68182=CARTESIAN_POINT('Ctrl Pts',(5.37115163104497,-0.473359678001532,
80.0277233747023));
#68183=CARTESIAN_POINT('Ctrl Pts',(3.31091438904171,4.25572380881061,80.1864841369483));
#68184=CARTESIAN_POINT('Ctrl Pts',(-1.77957283501041,5.089838873022,80.3452448991941));
#68185=CARTESIAN_POINT('Ctrl Pts',(-5.24134064269895,1.26557792949291,80.50400566144));
#68186=CARTESIAN_POINT('Ctrl Pts',(-3.9060733953589,-3.71697859269313,80.6627664236859));
#68187=CARTESIAN_POINT('Ctrl Pts',(1.00415153598694,-5.29764277024969,80.8215271859318));
#68188=CARTESIAN_POINT('Ctrl Pts',(4.99534630937428,-2.02974246588212,80.9802879481777));
#68189=CARTESIAN_POINT('Ctrl Pts',(4.41464755561157,3.0958401425779,81.1390487104235));
#68190=CARTESIAN_POINT('Ctrl Pts',(-0.206471488267744,5.38801528883197,
81.2978094726694));
#68191=CARTESIAN_POINT('Ctrl Pts',(-4.63862151922447,2.74891426377335,81.4565702349153));
#68192=CARTESIAN_POINT('Ctrl Pts',(-4.82536344745119,-2.40607706235473,
81.6153309971613));
#68193=CARTESIAN_POINT('Ctrl Pts',(-0.595785355535171,-5.35895316608133,
81.7740917594071));
#68194=CARTESIAN_POINT('Ctrl Pts',(4.17907369152063,-3.4071516415317,81.932852521653));
#68195=CARTESIAN_POINT('Ctrl Pts',(5.12911684605883,1.66297913944664,82.0916132838989));
#68196=CARTESIAN_POINT('Ctrl Pts',(1.38483558943104,5.2111006131604,82.2503740461447));
#68197=CARTESIAN_POINT('Ctrl Pts',(-3.62688949375241,3.98986363532597,82.4091348083908));
#68198=CARTESIAN_POINT('Ctrl Pts',(-5.31917453751786,-0.883018422641366,
82.5678955706364));
#68199=CARTESIAN_POINT('Ctrl Pts',(-2.1431885490041,-4.94773503060847,82.7266563328826));
#68200=CARTESIAN_POINT('Ctrl Pts',(2.99430902725335,-4.48413344144938,82.8854170951283));
#68201=CARTESIAN_POINT('Ctrl Pts',(5.39132358998814,0.0834841069729651,
83.0441778573743));
#68202=CARTESIAN_POINT('Ctrl Pts',(2.85403398786483,4.57469432804498,83.20293861962));
#68203=CARTESIAN_POINT('Ctrl Pts',(-2.29535443865746,4.87900479902879,83.3616993818661));
#68204=CARTESIAN_POINT('Ctrl Pts',(-5.34396486625942,0.717900597107141,
83.5204601441119));
#68205=CARTESIAN_POINT('Ctrl Pts',(-3.50161446504842,-4.10024729857536,
83.6792209063577));
#68206=CARTESIAN_POINT('Ctrl Pts',(1.54551863391146,-5.16572527246177,83.8379816686037));
#68207=CARTESIAN_POINT('Ctrl Pts',(5.17814935421542,-1.50337052857669,83.9967424308496));
#68208=CARTESIAN_POINT('Ctrl Pts',(4.07157294499926,3.5349087933154,84.1555031930955));
#68209=CARTESIAN_POINT('Ctrl Pts',(-0.761418612953421,5.33794320112753,
84.3142639553413));
#68210=CARTESIAN_POINT('Ctrl Pts',(-4.89756107214883,2.25550674636269,84.4730247175872));
#68211=CARTESIAN_POINT('Ctrl Pts',(-4.55125916712634,-2.89119586857457,
84.6317854798332));
#68212=CARTESIAN_POINT('Ctrl Pts',(-0.0395956256930076,-5.39186912790212,
84.7905462420789));
#68213=CARTESIAN_POINT('Ctrl Pts',(4.50847898005441,-2.95758313260692,84.949307004325));
#68214=CARTESIAN_POINT('Ctrl Pts',(4.92992660394334,2.18327463521188,85.1080677665708));
#68215=CARTESIAN_POINT('Ctrl Pts',(0.83998553543098,5.32650478551015,85.2668285288166));
#68216=CARTESIAN_POINT('Ctrl Pts',(-4.0199441247066,3.59365925042037,85.4255892910627));
#68217=CARTESIAN_POINT('Ctrl Pts',(-5.19838251798258,-1.4261119912042,85.5843500533084));
#68218=CARTESIAN_POINT('Ctrl Pts',(-1.62355247471041,-5.1447064563747,85.7431108155544));
#68219=CARTESIAN_POINT('Ctrl Pts',(3.44586114533526,-4.14677678635576,85.9018715778002));
#68220=CARTESIAN_POINT('Ctrl Pts',(5.02742464258896,-0.1665161442746,86.0341722130051));
#68221=CARTESIAN_POINT('Ctrl Pts',(3.86721841197903,2.75399303531867,86.1400127211691));
#68222=CARTESIAN_POINT('Ctrl Pts',(2.68386473467973,3.76615995447699,86.192932975251));
#68223=CARTESIAN_POINT('Ctrl Pts',(2.00237954638958,4.09906332620035,86.219393102292));
#68224=CARTESIAN_POINT('Ctrl Pts',(2.53835875722654,-3.55965150255068,26.));
#68225=CARTESIAN_POINT('Ctrl Pts',(3.13016463613492,-3.13763950664917,26.026460127041));
#68226=CARTESIAN_POINT('Ctrl Pts',(4.08944058768451,-1.99447514282845,26.079380381123));
#68227=CARTESIAN_POINT('Ctrl Pts',(4.72633908941221,0.949051473338421,26.1852208892869));
#68228=CARTESIAN_POINT('Ctrl Pts',(2.60449620246589,4.46265906441401,26.3175215244918));
#68229=CARTESIAN_POINT('Ctrl Pts',(-2.34489469821123,4.60777770546463,26.4762822867377));
#68230=CARTESIAN_POINT('Ctrl Pts',(-5.13873203824598,0.529582897206408,
26.6350430489835));
#68231=CARTESIAN_POINT('Ctrl Pts',(-3.23428844614615,-4.03017972072915,
26.7938038112295));
#68232=CARTESIAN_POINT('Ctrl Pts',(1.63279456941769,-4.90302026906412,26.9525645734753));
#68233=CARTESIAN_POINT('Ctrl Pts',(5.00417945325775,-1.28762125191842,27.1113253357213));
#68234=CARTESIAN_POINT('Ctrl Pts',(3.79627275763131,3.50580663842047,27.2700860979671));
#68235=CARTESIAN_POINT('Ctrl Pts',(-0.886457053099411,5.09084367591115,
27.428846860213));
#68236=CARTESIAN_POINT('Ctrl Pts',(-4.75768720014009,2.01646474678857,27.5876076224589));
#68237=CARTESIAN_POINT('Ctrl Pts',(-4.27463438144488,-2.90338148363688,
27.7463683847048));
#68238=CARTESIAN_POINT('Ctrl Pts',(0.12074539761077,-5.16599709979471,27.9051291469506));
#68239=CARTESIAN_POINT('Ctrl Pts',(4.40558866999103,-2.70051724468854,28.0638899091966));
#68240=CARTESIAN_POINT('Ctrl Pts',(4.65831652566081,2.23654953809766,28.2226506714425));
#68241=CARTESIAN_POINT('Ctrl Pts',(0.647603546994949,5.12666253671564,28.3814114336883));
#68242=CARTESIAN_POINT('Ctrl Pts',(-3.95581218859218,3.32469494777108,28.5401721959342));
#68243=CARTESIAN_POINT('Ctrl Pts',(-4.93874975649391,-1.52013373855127,
28.6989329581801));
#68244=CARTESIAN_POINT('Ctrl Pts',(-1.40159165779937,-4.9736902589037,28.857693720426));
#68245=CARTESIAN_POINT('Ctrl Pts',(3.41834539873403,-3.87517318393326,29.0164544826719));
#68246=CARTESIAN_POINT('Ctrl Pts',(5.10970861334159,0.770020576487015,29.1752152449178));
#68247=CARTESIAN_POINT('Ctrl Pts',(2.12451027984608,4.71046807932676,29.3339760071637));
#68248=CARTESIAN_POINT('Ctrl Pts',(-2.80510467897592,4.33975126344986,29.4927367694096));
#68249=CARTESIAN_POINT('Ctrl Pts',(-5.16740219266045,-0.00283844237382118,
29.6514975316555));
#68250=CARTESIAN_POINT('Ctrl Pts',(-2.80033535833003,-4.34283033250174,
29.8102582939013));
#68251=CARTESIAN_POINT('Ctrl Pts',(2.12968392236957,-4.70813124181331,29.9690190561473));
#68252=CARTESIAN_POINT('Ctrl Pts',(5.11055143098187,-0.764406630547101,
30.1277798183931));
#68253=CARTESIAN_POINT('Ctrl Pts',(3.41408616315334,3.87892628001712,30.286540580639));
#68254=CARTESIAN_POINT('Ctrl Pts',(-1.4070550442568,4.97214737476293,30.4453013428849));
#68255=CARTESIAN_POINT('Ctrl Pts',(-4.94041649691963,1.51470731642915,30.6040621051308));
#68256=CARTESIAN_POINT('Ctrl Pts',(-3.95215786419059,-3.32903914551084,
30.7628228673767));
#68257=CARTESIAN_POINT('Ctrl Pts',(0.653236365857992,-5.12594729451212,
30.9215836296226));
#68258=CARTESIAN_POINT('Ctrl Pts',(4.6607687206244,-2.23143190555148,31.0803443918685));
#68259=CARTESIAN_POINT('Ctrl Pts',(4.4026231771807,2.70535812338375,31.2391051541143));
#68260=CARTESIAN_POINT('Ctrl Pts',(0.115062422136807,5.16612176153803,31.3978659163603));
#68261=CARTESIAN_POINT('Ctrl Pts',(-4.27780697629061,2.89869296229943,31.5566266786061));
#68262=CARTESIAN_POINT('Ctrl Pts',(-4.7554967626928,-2.02170817777057,31.715387440852));
#68263=CARTESIAN_POINT('Ctrl Pts',(-0.880810653343035,-5.09178023966167,
31.8741482030979));
#68264=CARTESIAN_POINT('Ctrl Pts',(3.80002027066033,-3.5016994957634,32.0329089653438));
#68265=CARTESIAN_POINT('Ctrl Pts',(5.00295656982363,1.29324358746212,32.1916697275897));
#68266=CARTESIAN_POINT('Ctrl Pts',(1.62703419898677,4.90457063680218,32.3504304898356));
#68267=CARTESIAN_POINT('Ctrl Pts',(-3.23799956916984,4.02708482728032,32.5091912520815));
#68268=CARTESIAN_POINT('Ctrl Pts',(-5.13951722563736,-0.536112025076297,
32.6679520143274));
#68269=CARTESIAN_POINT('Ctrl Pts',(-2.33719172860392,-4.60864277632799,
32.8267127765732));
#68270=CARTESIAN_POINT('Ctrl Pts',(2.60420302889879,-4.4632028858578,32.9854735388192));
#68271=CARTESIAN_POINT('Ctrl Pts',(5.16215162793603,-0.232903383943239,
33.144234301065));
#68272=CARTESIAN_POINT('Ctrl Pts',(2.99554137711165,4.21055640908263,33.302995063311));
#68273=CARTESIAN_POINT('Ctrl Pts',(-1.91267984204806,4.80038636339596,33.4617558255568));
#68274=CARTESIAN_POINT('Ctrl Pts',(-5.07035804619892,0.996756088218607,
33.6205165878027));
#68275=CARTESIAN_POINT('Ctrl Pts',(-3.58748969036538,-3.71913580520757,
33.7792773500486));
#68276=CARTESIAN_POINT('Ctrl Pts',(1.17875881138994,-5.0311610072254,33.9380381122944));
#68277=CARTESIAN_POINT('Ctrl Pts',(4.86617124330449,-1.73851397661661,34.0967988745404));
#68278=CARTESIAN_POINT('Ctrl Pts',(4.09991511421076,3.14527414899259,34.2555596367862));
#68279=CARTESIAN_POINT('Ctrl Pts',(-0.418708560946466,5.15041129979394,
34.4143203990322));
#68280=CARTESIAN_POINT('Ctrl Pts',(-4.55411737150595,2.44173470766227,34.5730811612781));
#68281=CARTESIAN_POINT('Ctrl Pts',(-4.5214588563368,-2.50169207267966,34.7318419235239));
#68282=CARTESIAN_POINT('Ctrl Pts',(-0.350623086089188,-5.15549385292585,
34.8906026857698));
#68283=CARTESIAN_POINT('Ctrl Pts',(4.14111364246891,-3.09083018236409,35.0493634480157));
#68284=CARTESIAN_POINT('Ctrl Pts',(4.84277667347619,1.80265568173448,35.2081242102616));
#68285=CARTESIAN_POINT('Ctrl Pts',(1.11218256837853,5.0462960030749,35.3668849725075));
#68286=CARTESIAN_POINT('Ctrl Pts',(-3.63631499535807,3.67141208128276,35.5256457347534));
#68287=CARTESIAN_POINT('Ctrl Pts',(-5.05674600265519,-1.06366032204162,
35.6844064969993));
#68288=CARTESIAN_POINT('Ctrl Pts',(-1.84908860800444,-4.8252383087059,35.8431672592452));
#68289=CARTESIAN_POINT('Ctrl Pts',(3.05091116183891,-4.17061080641931,36.0019280214911));
#68290=CARTESIAN_POINT('Ctrl Pts',(5.15862384507246,0.301087098868051,36.1606887837369));
#68291=CARTESIAN_POINT('Ctrl Pts',(2.54500641307862,4.49722089444621,36.3194495459828));
#68292=CARTESIAN_POINT('Ctrl Pts',(-2.39787862639785,4.5773607580263,36.4782103082287));
#68293=CARTESIAN_POINT('Ctrl Pts',(-5.14615190283867,0.468160238555881,
36.6369710704746));
#68294=CARTESIAN_POINT('Ctrl Pts',(-3.18450976654496,-4.06951483138158,
36.7957318327205));
#68295=CARTESIAN_POINT('Ctrl Pts',(1.69169298020808,-4.88264562268956,36.9544925949664));
#68296=CARTESIAN_POINT('Ctrl Pts',(5.01960663803976,-1.22702999775959,37.1132533572123));
#68297=CARTESIAN_POINT('Ctrl Pts',(3.75342297485632,3.55160096123927,37.2720141194582));
#68298=CARTESIAN_POINT('Ctrl Pts',(-0.94800804471325,5.07969823544803,37.430774881704));
#68299=CARTESIAN_POINT('Ctrl Pts',(-4.78179314447847,1.95870052317183,37.58953564395));
#68300=CARTESIAN_POINT('Ctrl Pts',(-4.23913509664356,-2.95495973719773,
37.7482964061958));
#68301=CARTESIAN_POINT('Ctrl Pts',(0.183308877707052,-5.16415058566349,
37.9070571684418));
#68302=CARTESIAN_POINT('Ctrl Pts',(4.43798296793759,-2.64695307709652,38.0658179306876));
#68303=CARTESIAN_POINT('Ctrl Pts',(4.63087948595682,2.29281673986369,38.2245786929335));
#68304=CARTESIAN_POINT('Ctrl Pts',(0.585453646372677,5.13413064150142,38.3833394551794));
#68305=CARTESIAN_POINT('Ctrl Pts',(-3.99579725328622,3.27653135597467,38.5421002174253));
#68306=CARTESIAN_POINT('Ctrl Pts',(-4.91997245352125,-1.57984950949354,
38.7008609796712));
#68307=CARTESIAN_POINT('Ctrl Pts',(-1.34123858177823,-4.99030384674165,
38.8596217419171));
#68308=CARTESIAN_POINT('Ctrl Pts',(3.46503780867414,-3.83347967263602,39.0183825041629));
#68309=CARTESIAN_POINT('Ctrl Pts',(5.10000575566994,0.831862193027325,39.1771432664089));
#68310=CARTESIAN_POINT('Ctrl Pts',(2.06729265337245,4.73585837007054,39.3359040286547));
#68311=CARTESIAN_POINT('Ctrl Pts',(-2.85746983156782,4.30545230814772,39.4946647909006));
#68312=CARTESIAN_POINT('Ctrl Pts',(-5.16698864410473,-0.0654352179449955,
39.6534255531465));
#68313=CARTESIAN_POINT('Ctrl Pts',(-2.74752162183386,-4.3764344338297,39.8121863153924));
#68314=CARTESIAN_POINT('Ctrl Pts',(2.18656111288008,-4.68198717594309,39.9709470776383));
#68315=CARTESIAN_POINT('Ctrl Pts',(5.11943632770732,-0.702442241472902,
40.1297078398842));
#68316=CARTESIAN_POINT('Ctrl Pts',(3.36684704019806,3.9199992887709,40.2884686021301));
#68317=CARTESIAN_POINT('Ctrl Pts',(-1.46718350018236,4.95473773199425,40.4472293643759));
#68318=CARTESIAN_POINT('Ctrl Pts',(-4.95840288549236,1.45474885846183,40.6059901266218));
#68319=CARTESIAN_POINT('Ctrl Pts',(-3.91154049361154,-3.37667060621731,
40.7647508888677));
#68320=CARTESIAN_POINT('Ctrl Pts',(0.715283237582617,-5.11765799033974,
40.9235116511136));
#68321=CARTESIAN_POINT('Ctrl Pts',(4.6874579011302,-2.17480846080452,41.0822724133595));
#68322=CARTESIAN_POINT('Ctrl Pts',(4.36952791329752,2.75849220244841,41.2410331756054));
#68323=CARTESIAN_POINT('Ctrl Pts',(0.052472510246957,5.16713654277911,41.3997939378513));
#68324=CARTESIAN_POINT('Ctrl Pts',(-4.3126073369753,2.84665968691757,41.5585547000972));
#68325=CARTESIAN_POINT('Ctrl Pts',(-4.73065721909144,-2.07916706676323,
41.7173154623431));
#68326=CARTESIAN_POINT('Ctrl Pts',(-0.819065114488867,-5.10207661195736,
41.8760762245889));
#68327=CARTESIAN_POINT('Ctrl Pts',(3.8421604015636,-3.45540979692878,42.0348369868349));
#68328=CARTESIAN_POINT('Ctrl Pts',(4.98692335778749,1.35375361111553,42.1935977490807));
#68329=CARTESIAN_POINT('Ctrl Pts',(1.56750172940691,4.92392036332446,42.3523585113267));
#68330=CARTESIAN_POINT('Ctrl Pts',(-3.28654536169065,3.98756479591298,42.5111192735724));
#68331=CARTESIAN_POINT('Ctrl Pts',(-5.13264574893371,-0.59833187447071,
42.6698800358185));
#68332=CARTESIAN_POINT('Ctrl Pts',(-2.28119196804685,-4.63661693705371,
42.8286407980642));
#68333=CARTESIAN_POINT('Ctrl Pts',(2.65807838191241,-4.43132855153674,42.9874015603103));
#68334=CARTESIAN_POINT('Ctrl Pts',(5.1645942046841,-0.170352918960309,43.146162322556));
#68335=CARTESIAN_POINT('Ctrl Pts',(2.94431565674484,4.24653490854626,43.304923084802));
#68336=CARTESIAN_POINT('Ctrl Pts',(-1.97069051554003,4.77686427565358,43.4636838470478));
#68337=CARTESIAN_POINT('Ctrl Pts',(-5.0820605324771,0.935261546463589,43.6224446092938));
#68338=CARTESIAN_POINT('Ctrl Pts',(-3.54217351653091,-3.76232111798581,
43.7812053715396));
#68339=CARTESIAN_POINT('Ctrl Pts',(1.23961889884326,-5.01651257365967,43.9399661337855));
#68340=CARTESIAN_POINT('Ctrl Pts',(4.88687423334376,-1.67943849054845,44.0987268960314));
#68341=CARTESIAN_POINT('Ctrl Pts',(4.06151299797099,3.19470899822934,44.2574876582773));
#68342=CARTESIAN_POINT('Ctrl Pts',(-0.481068993674721,5.1449612281707,44.4162484205232));
#68343=CARTESIAN_POINT('Ctrl Pts',(-4.5833619478656,2.38638778720321,44.5750091827691));
#68344=CARTESIAN_POINT('Ctrl Pts',(-4.49082204675623,-2.55628064977671,
44.733769945015));
#68345=CARTESIAN_POINT('Ctrl Pts',(-0.288144634510089,-5.15936295347187,
44.8925307072609));
#68346=CARTESIAN_POINT('Ctrl Pts',(4.17825154873217,-3.04043868735616,45.0512914695067));
#68347=CARTESIAN_POINT('Ctrl Pts',(4.8205842882194,1.86118793683688,45.2100522317526));
#68348=CARTESIAN_POINT('Ctrl Pts',(1.05097104046387,5.05939851051103,45.3688129939986));
#68349=CARTESIAN_POINT('Ctrl Pts',(-3.68052300585259,3.62709302602572,45.5275737562444));
#68350=CARTESIAN_POINT('Ctrl Pts',(-5.04348997417376,-1.12483878687734,
45.6863345184903));
#68351=CARTESIAN_POINT('Ctrl Pts',(-1.79050086272392,-4.84728378338218,
45.8450952807362));
#68352=CARTESIAN_POINT('Ctrl Pts',(3.1012093298518,-4.13334659912459,46.0038560429821));
#68353=CARTESIAN_POINT('Ctrl Pts',(5.15459801607478,0.363555647367575,46.162616805228));
#68354=CARTESIAN_POINT('Ctrl Pts',(2.49034114873962,4.52772066043712,46.3213775674739));
#68355=CARTESIAN_POINT('Ctrl Pts',(-2.45315200638293,4.54797742404625,46.4801383297198));
#68356=CARTESIAN_POINT('Ctrl Pts',(-5.15144551276008,0.405786329388982,
46.6388990919657));
#68357=CARTESIAN_POINT('Ctrl Pts',(-3.13497873290715,-4.10779280882992,
46.7976598542116));
#68358=CARTESIAN_POINT('Ctrl Pts',(1.75071634247466,-4.86179449424254,46.9564206164574));
#68359=CARTESIAN_POINT('Ctrl Pts',(5.03410234489664,-1.16613335307792,47.1151813787034));
#68360=CARTESIAN_POINT('Ctrl Pts',(3.71012411261097,3.59680865283067,47.2739421409492));
#68361=CARTESIAN_POINT('Ctrl Pts',(-1.00947303475291,5.06784151371782,47.4327029031951));
#68362=CARTESIAN_POINT('Ctrl Pts',(-4.80516962595556,1.90063102201579,47.5914636654409));
#68363=CARTESIAN_POINT('Ctrl Pts',(-4.20302819966638,-3.00609503656556,
47.750224427687));
#68364=CARTESIAN_POINT('Ctrl Pts',(0.245853018125491,-5.16155109531365,
47.9089851899327));
#68365=CARTESIAN_POINT('Ctrl Pts',(4.46972204405066,-2.59299792999961,48.0677459521787));
#68366=CARTESIAN_POINT('Ctrl Pts',(4.60276492582317,2.34874614500311,48.2265067144246));
#68367=CARTESIAN_POINT('Ctrl Pts',(0.523216754197009,5.14084600471386,48.3852674766704));
#68368=CARTESIAN_POINT('Ctrl Pts',(-4.03519537273411,3.22788657172462,48.5440282389163));
#68369=CARTESIAN_POINT('Ctrl Pts',(-4.9004734378914,-1.63933324878614,48.7027890011622));
#68370=CARTESIAN_POINT('Ctrl Pts',(-1.2806885257803,-5.00618520592171,48.8615497634081));
#68371=CARTESIAN_POINT('Ctrl Pts',(3.51122164426531,-3.79122354667958,49.020310525654));
#68372=CARTESIAN_POINT('Ctrl Pts',(5.0895545138177,0.893581706914796,49.1790712878999));
#68373=CARTESIAN_POINT('Ctrl Pts',(2.00977162985725,4.76055368753214,49.3378320501457));
#68374=CARTESIAN_POINT('Ctrl Pts',(-2.90941563902232,4.27052152031426,49.4965928123917));
#68375=CARTESIAN_POINT('Ctrl Pts',(-5.1658168458108,-0.128022387073527,
49.6553535746375));
#68376=CARTESIAN_POINT('Ctrl Pts',(-2.69430468338317,-4.40939629531691,
49.8141143368835));
#68377=CARTESIAN_POINT('Ctrl Pts',(2.2431174238849,-4.6551560273227,49.9728750991294));
#68378=CARTESIAN_POINT('Ctrl Pts',(5.12756994789964,-0.640374769530455,
50.1316358613752));
#68379=CARTESIAN_POINT('Ctrl Pts',(3.31911383193326,3.96049703783808,50.2903966236212));
#68380=CARTESIAN_POINT('Ctrl Pts',(-1.52709664667054,4.93660098122003,50.4491573858669));
#68381=CARTESIAN_POINT('Ctrl Pts',(-4.975661628467,1.39457691614903,50.607918148113));
#68382=CARTESIAN_POINT('Ctrl Pts',(-3.87034910432713,-3.42380654048809,
50.7666789103588));
#68383=CARTESIAN_POINT('Ctrl Pts',(0.777225141445664,-5.10861766973804,
50.9254396726047));
#68384=CARTESIAN_POINT('Ctrl Pts',(4.71345919711634,-2.11786586288516,51.0842004348506));
#68385=CARTESIAN_POINT('Ctrl Pts',(4.33579142110028,2.81122147273531,51.2429611970965));
#68386=CARTESIAN_POINT('Ctrl Pts',(-0.0101251019801382,5.16739304663044,
51.4017219593423));
#68387=CARTESIAN_POINT('Ctrl Pts',(-4.34677482245307,2.79420866417363,51.5604827215882));
#68388=CARTESIAN_POINT('Ctrl Pts',(-4.7051234514512,-2.13632083794987,51.7192434838341));
#68389=CARTESIAN_POINT('Ctrl Pts',(-0.757199377814005,-5.111624254412,51.87800424608));
#68390=CARTESIAN_POINT('Ctrl Pts',(3.88373669535471,-3.40861301664037,52.0367650083259));
#68391=CARTESIAN_POINT('Ctrl Pts',(4.97015831465276,1.41406497140078,52.1955257705718));
#68392=CARTESIAN_POINT('Ctrl Pts',(1.50773922891819,4.94254750443899,52.3542865328176));
#68393=CARTESIAN_POINT('Ctrl Pts',(-3.33460885361675,3.94745958933536,52.5130472950636));
#68394=CARTESIAN_POINT('Ctrl Pts',(-5.12502105636793,-0.660463918651125,
52.6718080573094));
#68395=CARTESIAN_POINT('Ctrl Pts',(-2.22485744252472,-4.66391067415503,
52.8305688195554));
#68396=CARTESIAN_POINT('Ctrl Pts',(2.71156366187259,-4.39880391966578,52.9893295818012));
#68397=CARTESIAN_POINT('Ctrl Pts',(5.16627887713359,-0.107777454683187,
53.1480903440472));
#68398=CARTESIAN_POINT('Ctrl Pts',(2.89265785799892,4.28189022893068,53.306851106293));
#68399=CARTESIAN_POINT('Ctrl Pts',(-2.02841199016113,4.75264118298715,53.4656118685389));
#68400=CARTESIAN_POINT('Ctrl Pts',(-5.09301722627474,0.873629755058583,
53.6243726307848));
#68401=CARTESIAN_POINT('Ctrl Pts',(-3.49633752866489,-3.80495431006791,
53.7831333930307));
#68402=CARTESIAN_POINT('Ctrl Pts',(1.30029707219943,-5.00112796677752,53.9418941552766));
#68403=CARTESIAN_POINT('Ctrl Pts',(4.90686007449561,-1.62011654684958,54.1006549175225));
#68404=CARTESIAN_POINT('Ctrl Pts',(4.02251485462088,3.2436750238594,54.2594156797684));
#68405=CARTESIAN_POINT('Ctrl Pts',(-0.543358829519001,5.13875613338857,
54.4181764420142));
#68406=CARTESIAN_POINT('Ctrl Pts',(-4.61193391577151,2.33069066429059,54.5769372042602));
#68407=CARTESIAN_POINT('Ctrl Pts',(-4.4595262089542,-2.61049409263942,54.735697966506));
#68408=CARTESIAN_POINT('Ctrl Pts',(-0.22562389770033,-5.16247491740555,
54.8944587287519));
#68409=CARTESIAN_POINT('Ctrl Pts',(4.21477629650059,-2.98960100791253,55.0532194909978));
#68410=CARTESIAN_POINT('Ctrl Pts',(4.79768448212587,1.91944706257383,55.2119802532437));
#68411=CARTESIAN_POINT('Ctrl Pts',(0.989605282528937,5.07175855111871,55.3707410154895));
#68412=CARTESIAN_POINT('Ctrl Pts',(-3.72419089952545,3.58224169479765,55.5295017777355));
#68413=CARTESIAN_POINT('Ctrl Pts',(-5.0294938134419,-1.1858521815995,55.6882625399813));
#68414=CARTESIAN_POINT('Ctrl Pts',(-1.7316503614075,-4.86861791907028,55.8470233022273));
#68415=CARTESIAN_POINT('Ctrl Pts',(3.15105239533607,-4.09547582313724,56.0057840644731));
#68416=CARTESIAN_POINT('Ctrl Pts',(5.14981574971942,0.425970844068908,56.1645448267191));
#68417=CARTESIAN_POINT('Ctrl Pts',(2.43531042678924,4.55755598333432,56.3233055889649));
#68418=CARTESIAN_POINT('Ctrl Pts',(-2.50806538626398,4.517926674292,56.4820663512109));
#68419=CARTESIAN_POINT('Ctrl Pts',(-5.1559831479537,0.343352871070528,56.6408271134567));
#68420=CARTESIAN_POINT('Ctrl Pts',(-3.08498764108028,-4.14546796760472,
56.7995878757026));
#68421=CARTESIAN_POINT('Ctrl Pts',(1.8094827870843,-4.8402298973603,56.9583486379485));
#68422=CARTESIAN_POINT('Ctrl Pts',(5.04785929713791,-1.10506557830443,57.1171094001944));
#68423=CARTESIAN_POINT('Ctrl Pts',(3.66628078958101,3.64148851268323,57.2758701624403));
#68424=CARTESIAN_POINT('Ctrl Pts',(-1.07078988460527,5.05524108614831,57.4346309246862));
#68425=CARTESIAN_POINT('Ctrl Pts',(-4.82784094869794,1.84228260322088,57.593391686932));
#68426=CARTESIAN_POINT('Ctrl Pts',(-4.16630450822031,-3.05678919142909,
57.7521524491779));
#68427=CARTESIAN_POINT('Ctrl Pts',(0.308361079608735,-5.1581941472416,57.9109132114238));
#68428=CARTESIAN_POINT('Ctrl Pts',(4.50080518836808,-2.53866226040682,58.0696739736697));
#68429=CARTESIAN_POINT('Ctrl Pts',(4.57397490984839,2.40433087160068,58.2284347359156));
#68430=CARTESIAN_POINT('Ctrl Pts',(0.460903079952699,5.14680694867653,58.3871954981615));
#68431=CARTESIAN_POINT('Ctrl Pts',(-4.07400132718361,3.17876809505837,58.5459562604074));
#68432=CARTESIAN_POINT('Ctrl Pts',(-4.88025527769062,-1.69857641589297,
58.7047170226532));
#68433=CARTESIAN_POINT('Ctrl Pts',(-1.21995052871669,-5.02133190732686,
58.8634777848992));
#68434=CARTESIAN_POINT('Ctrl Pts',(3.55689020801282,-3.74841105859499,59.022238547145));
#68435=CARTESIAN_POINT('Ctrl Pts',(5.07835637974298,0.955170087669591,59.1809993093909));
#68436=CARTESIAN_POINT('Ctrl Pts',(1.95195567231696,4.78455039364876,59.3397600716368));
#68437=CARTESIAN_POINT('Ctrl Pts',(-2.96093448967591,4.23496403336588,59.4985208338827));
#68438=CARTESIAN_POINT('Ctrl Pts',(-5.16388696379574,-0.190590768914221,
59.6572815961286));
#68439=CARTESIAN_POINT('Ctrl Pts',(-2.6406923556686,-4.44171107781315,59.8160423583745));
#68440=CARTESIAN_POINT('Ctrl Pts',(2.29934455736468,-4.62764173446609,59.9748031206204));
#68441=CARTESIAN_POINT('Ctrl Pts',(5.13495109710383,-0.578213322578349,
60.1335638828663));
#68442=CARTESIAN_POINT('Ctrl Pts',(3.27089354364999,4.00041358388897,60.2923246451122));
#68443=CARTESIAN_POINT('Ctrl Pts',(-1.58678569169648,4.91773978415717,60.451085407358));
#68444=CARTESIAN_POINT('Ctrl Pts',(-4.99219019300232,1.33420031964711,60.6098461696039));
#68445=CARTESIAN_POINT('Ctrl Pts',(-3.82858974123746,-3.47044003108337,
60.7686069318499));
#68446=CARTESIAN_POINT('Ctrl Pts',(0.839052987504236,-5.09882765939536,
60.9273676940957));
#68447=CARTESIAN_POINT('Ctrl Pts',(4.73876879287487,-2.06061246810993,61.0861284563416));
#68448=CARTESIAN_POINT('Ctrl Pts',(4.30141865142892,2.86353819621711,61.2448892185875));
#68449=CARTESIAN_POINT('Ctrl Pts',(-0.0727212283482856,5.16689123545314,
61.4036499808334));
#68450=CARTESIAN_POINT('Ctrl Pts',(-4.38030441864225,2.74134759125467,61.5624107430792));
#68451=CARTESIAN_POINT('Ctrl Pts',(-4.67889920685427,-2.19316110401252,
61.7211715053253));
#68452=CARTESIAN_POINT('Ctrl Pts',(-0.695222522116061,-5.12042176590928,
61.879932267571));
#68453=CARTESIAN_POINT('Ctrl Pts',(3.92474305071123,-3.3613160223265,62.038693029817));
#68454=CARTESIAN_POINT('Ctrl Pts',(4.95266390069012,1.47416881762428,62.1974537920629));
#68455=CARTESIAN_POINT('Ctrl Pts',(1.4477554676688,4.96044932661243,62.3562145543087));
#68456=CARTESIAN_POINT('Ctrl Pts',(-3.38218299162958,3.90677509298738,62.5149753165547));
#68457=CARTESIAN_POINT('Ctrl Pts',(-5.11664426686392,-0.722499039738782,
62.6737360788005));
#68458=CARTESIAN_POINT('Ctrl Pts',(-2.16819641913028,-4.69051998227545,
62.8324968410464));
#68459=CARTESIAN_POINT('Ctrl Pts',(2.76465101981334,-4.3656337632353,62.9912576032923));
#68460=CARTESIAN_POINT('Ctrl Pts',(5.16720539805885,-0.0451861740625634,
63.1500183655382));
#68461=CARTESIAN_POINT('Ctrl Pts',(2.8405755616569,4.31661718184185,63.308779127784));
#68462=CARTESIAN_POINT('Ctrl Pts',(-2.08583579528372,4.72772064013601,63.46753989003));
#68463=CARTESIAN_POINT('Ctrl Pts',(-5.10322651969674,0.811869758470405,
63.6263006522758));
#68464=CARTESIAN_POINT('Ctrl Pts',(-3.44998845319957,-3.847029125032,63.7850614145218));
#68465=CARTESIAN_POINT('Ctrl Pts',(1.36078442693529,-4.98500944427043,63.9438221767676));
#68466=CARTESIAN_POINT('Ctrl Pts',(4.92612583383742,-1.56055685101642,64.1025829390136));
#68467=CARTESIAN_POINT('Ctrl Pts',(3.98292640713875,3.29216504011747,64.2613437012594));
#68468=CARTESIAN_POINT('Ctrl Pts',(-0.605568927444514,5.13179692604536,
64.4201044635054));
#68469=CARTESIAN_POINT('Ctrl Pts',(-4.63982908228685,2.27465151247837,64.5788652257511));
#68470=CARTESIAN_POINT('Ctrl Pts',(-4.42757593559553,-2.66432444544396,
64.7376259879972));
#68471=CARTESIAN_POINT('Ctrl Pts',(-0.163070050579303,-5.16482928804609,
64.8963867502428));
#68472=CARTESIAN_POINT('Ctrl Pts',(4.25068252576661,-2.93832460446375,65.0551475124889));
#68473=CARTESIAN_POINT('Ctrl Pts',(4.77408061574266,1.97742450941745,65.2139082747347));
#68474=CARTESIAN_POINT('Ctrl Pts',(0.928094299999949,5.08337431106172,65.3726690369806));
#68475=CARTESIAN_POINT('Ctrl Pts',(-3.76731226811231,3.53686466953228,65.5314297992265));
#68476=CARTESIAN_POINT('Ctrl Pts',(-5.01475957439658,-1.24669155249126,
65.6901905614724));
#68477=CARTESIAN_POINT('Ctrl Pts',(-1.67254574036732,-4.88923758498539,
65.8489513237183));
#68478=CARTESIAN_POINT('Ctrl Pts',(3.20043304382085,-4.05700403599433,66.0077120859643));
#68479=CARTESIAN_POINT('Ctrl Pts',(5.14427774780404,0.488323529540513,66.16647284821));
#68480=CARTESIAN_POINT('Ctrl Pts',(2.3799223229872,4.58672248480354,66.3252336104561));
#68481=CARTESIAN_POINT('Ctrl Pts',(-2.56261070750152,4.48721291871176,66.4839943727018));
#68482=CARTESIAN_POINT('Ctrl Pts',(-5.15976414252148,0.280869025711643,
66.6427551349478));
#68483=CARTESIAN_POINT('Ctrl Pts',(-3.03454382725794,-4.18253477887576,
66.8015158971936));
#68484=CARTESIAN_POINT('Ctrl Pts',(1.86798369006022,-4.81795499664787,66.9602766594396));
#68485=CARTESIAN_POINT('Ctrl Pts',(5.06087547593053,-1.04383563513614,67.1190374216854));
#68486=CARTESIAN_POINT('Ctrl Pts',(3.62189943977487,3.68563398402679,67.2777981839313));
#68487=CARTESIAN_POINT('Ctrl Pts',(-1.13194959602156,5.04189880185246,67.4365589461772));
#68488=CARTESIAN_POINT('Ctrl Pts',(-4.84980378568845,1.78366382941869,67.5953197084231));
#68489=CARTESIAN_POINT('Ctrl Pts',(-4.12896941150786,-3.10703476242022,
67.754080470669));
#68490=CARTESIAN_POINT('Ctrl Pts',(0.370823889097725,-5.15408023407956,
67.9128412329148));
#68491=CARTESIAN_POINT('Ctrl Pts',(4.53122783943781,-2.48395404207855,68.0716019951608));
#68492=CARTESIAN_POINT('Ctrl Pts',(4.5445136629679,2.45956276259679,68.2303627574067));
#68493=CARTESIAN_POINT('Ctrl Pts',(0.398521768172548,5.15201259862078,68.3891235196525));
#68494=CARTESIAN_POINT('Ctrl Pts',(-4.11220942186021,3.12918313411324,68.5478842818985));
#68495=CARTESIAN_POINT('Ctrl Pts',(-4.85932093993431,-1.75757031687816,
68.7066450441443));
#68496=CARTESIAN_POINT('Ctrl Pts',(-1.15903350388962,-5.03574172817834,
68.8654058063903));
#68497=CARTESIAN_POINT('Ctrl Pts',(3.60203679805415,-3.70504849111566,69.0241665686361));
#68498=CARTESIAN_POINT('Ctrl Pts',(5.06641299677213,1.01661829719571,69.182927330882));
#68499=CARTESIAN_POINT('Ctrl Pts',(1.89385326524434,4.80784496690336,69.3416880931279));
#68500=CARTESIAN_POINT('Ctrl Pts',(-3.01201882313635,4.19878506536444,69.5004488553738));
#68501=CARTESIAN_POINT('Ctrl Pts',(-5.16119928126974,-0.25313118155592,
69.6592096176196));
#68502=CARTESIAN_POINT('Ctrl Pts',(-2.58669250630018,-4.47337403912361,
69.8179703798655));
#68503=CARTESIAN_POINT('Ctrl Pts',(2.35523426198658,-4.5994483350962,69.9767311421114));
#68504=CARTESIAN_POINT('Ctrl Pts',(5.14157869213602,-0.51596702281012,70.1354919043573));
#68505=CARTESIAN_POINT('Ctrl Pts',(3.22219325167658,4.03974306916968,70.2942526666032));
#68506=CARTESIAN_POINT('Ctrl Pts',(-1.6462418758917,4.89815690868675,70.4530134288491));
#68507=CARTESIAN_POINT('Ctrl Pts',(-5.00798615353109,1.2736279292227,70.611774191095));
#68508=CARTESIAN_POINT('Ctrl Pts',(-3.78626853252985,-3.51656423453759,
70.7705349533408));
#68509=CARTESIAN_POINT('Ctrl Pts',(0.900757702520816,-5.08828939599587,
70.9292957155868));
#68510=CARTESIAN_POINT('Ctrl Pts',(4.76338297422217,-2.00305667841551,71.0880564778326));
#68511=CARTESIAN_POINT('Ctrl Pts',(4.26641464848803,2.9154346954137,71.2468172400786));
#68512=CARTESIAN_POINT('Ctrl Pts',(-0.135306682874774,5.16563118288797,
71.4055780023244));
#68513=CARTESIAN_POINT('Ctrl Pts',(-4.41319120507407,2.6880842255241,71.5643387645703));
#68514=CARTESIAN_POINT('Ctrl Pts',(-4.65198833370899,-2.24967952364111,
71.7230995268162));
#68515=CARTESIAN_POINT('Ctrl Pts',(-0.63314364249968,-5.12846785541421,
71.8818602890621));
#68516=CARTESIAN_POINT('Ctrl Pts',(3.9651734499498,-3.31352575482195,72.040621051308));
#68517=CARTESIAN_POINT('Ctrl Pts',(4.93444268320512,1.53405632954553,72.1993818135539));
#68518=CARTESIAN_POINT('Ctrl Pts',(1.38755924827672,4.97762320275213,72.3581425757998));
#68519=CARTESIAN_POINT('Ctrl Pts',(-3.42926079422353,3.86551727731956,72.5169033380456));
#68520=CARTESIAN_POINT('Ctrl Pts',(-5.10751660971561,-0.784428134078424,
72.6756641002916));
#68521=CARTESIAN_POINT('Ctrl Pts',(-2.1112172128698,-4.71644095649861,72.8344248625374));
#68522=CARTESIAN_POINT('Ctrl Pts',(2.81733266516402,-4.33182294996633,72.9931856247833));
#68523=CARTESIAN_POINT('Ctrl Pts',(5.16737363149282,0.0174117376300544,
73.1519463870293));
#68524=CARTESIAN_POINT('Ctrl Pts',(2.78807641079671,4.35071067109887,73.3107071492751));
#68525=CARTESIAN_POINT('Ctrl Pts',(-2.14295350396336,4.70210630419026,73.469467911521));
#68526=CARTESIAN_POINT('Ctrl Pts',(-5.11268691452911,0.749990619979619,
73.6282286737669));
#68527=CARTESIAN_POINT('Ctrl Pts',(-3.40313309186266,-3.88853938839824,
73.7869894360128));
#68528=CARTESIAN_POINT('Ctrl Pts',(1.42107208653042,-4.9681593715318,73.9457501982587));
#68529=CARTESIAN_POINT('Ctrl Pts',(4.94466868411869,-1.50076814343543,74.1045109605046));
#68530=CARTESIAN_POINT('Ctrl Pts',(3.94275346512999,3.34017193109278,74.2632717227505));
#68531=CARTESIAN_POINT('Ctrl Pts',(-0.667690158118302,5.12408462740484,
74.4220324849963));
#68532=CARTESIAN_POINT('Ctrl Pts',(-4.6670433537954,2.21827855551313,74.5807932472423));
#68533=CARTESIAN_POINT('Ctrl Pts',(-4.39497591538344,-2.71776380858505,
74.7395540094881));
#68534=CARTESIAN_POINT('Ctrl Pts',(-0.100492272925181,-5.16642571988962,
74.898314771734));
#68535=CARTESIAN_POINT('Ctrl Pts',(4.28596496729055,-2.88661700182285,75.0570755339799));
#68536=CARTESIAN_POINT('Ctrl Pts',(4.74977615293751,2.03511176917654,75.2158362962258));
#68537=CARTESIAN_POINT('Ctrl Pts',(0.866447119614458,5.09424408572719,75.3745970584717));
#68538=CARTESIAN_POINT('Ctrl Pts',(-3.8098807835517,3.4909686093087,75.5333578207175));
#68539=CARTESIAN_POINT('Ctrl Pts',(-4.99928941928749,-1.30734797137385,
75.6921185829635));
#68540=CARTESIAN_POINT('Ctrl Pts',(-1.61319567320764,-4.90913975519121,
75.8508793452094));
#68541=CARTESIAN_POINT('Ctrl Pts',(3.24934402869518,-4.01793688343129,76.0096401074552));
#68542=CARTESIAN_POINT('Ctrl Pts',(5.13798482303055,0.550604553524979,76.1684008697012));
#68543=CARTESIAN_POINT('Ctrl Pts',(2.32418496553848,4.61521588466023,76.3271616319469));
#68544=CARTESIAN_POINT('Ctrl Pts',(-2.61677996556865,4.45584066454958,76.485922394193));
#68545=CARTESIAN_POINT('Ctrl Pts',(-5.16278794160245,0.218343962817818,
76.6446831564387));
#68546=CARTESIAN_POINT('Ctrl Pts',(-2.98365469407069,-4.21898780308791,
76.8034439186847));
#68547=CARTESIAN_POINT('Ctrl Pts',(1.92621046639379,-4.79497306094723,76.9622046809306));
#68548=CARTESIAN_POINT('Ctrl Pts',(5.07314897115,-0.982452509068445,77.1209654431764));
#68549=CARTESIAN_POINT('Ctrl Pts',(3.5769865761566,3.7292385885125,77.2797262054224));
#68550=CARTESIAN_POINT('Ctrl Pts',(-1.19294319381297,5.02781661881079,77.4384869676682));
#68551=CARTESIAN_POINT('Ctrl Pts',(-4.87105491388051,1.72478330291522,77.5972477299142));
#68552=CARTESIAN_POINT('Ctrl Pts',(-4.09102838845504,-3.1568243760003,77.75600849216));
#68553=CARTESIAN_POINT('Ctrl Pts',(0.433232280173729,-5.14920995954434,
77.9147692544059));
#68554=CARTESIAN_POINT('Ctrl Pts',(4.56098553273524,-2.42888130344712,78.0735300166518));
#68555=CARTESIAN_POINT('Ctrl Pts',(4.51438550862023,2.51443371271033,78.2322907788977));
#68556=CARTESIAN_POINT('Ctrl Pts',(0.336081973315249,5.15646219061744,78.3910515411436));
#68557=CARTESIAN_POINT('Ctrl Pts',(-4.1498140497254,3.0791389654831,78.5498123033895));
#68558=CARTESIAN_POINT('Ctrl Pts',(-4.8376734967368,-1.81630629438564,78.7085730656354));
#68559=CARTESIAN_POINT('Ctrl Pts',(-1.0979463908737,-5.04941255383462,78.8673338278812));
#68560=CARTESIAN_POINT('Ctrl Pts',(3.64665478912629,-3.66114220769932,79.0260945901272));
#68561=CARTESIAN_POINT('Ctrl Pts',(5.05372611759689,1.07791731796727,79.184855352373));
#68562=CARTESIAN_POINT('Ctrl Pts',(1.83547293516864,4.83043398881696,79.3436161146189));
#68563=CARTESIAN_POINT('Ctrl Pts',(-3.06266114277673,4.16198992557408,79.5023768768648));
#68564=CARTESIAN_POINT('Ctrl Pts',(-5.15775419265022,-0.315634447191765,
79.6611376391107));
#68565=CARTESIAN_POINT('Ctrl Pts',(-2.53231305975701,-4.50438053270811,
79.8198984013567));
#68566=CARTESIAN_POINT('Ctrl Pts',(2.41077833593552,-4.57057996659486,79.9786591636024));
#68567=CARTESIAN_POINT('Ctrl Pts',(5.14745176039643,-0.453645004871452,
80.1374199258484));
#68568=CARTESIAN_POINT('Ctrl Pts',(3.1730201027819,4.07847972207792,80.2961806880942));
#68569=CARTESIAN_POINT('Ctrl Pts',(-1.70545647406065,4.87785522859546,80.4549414503402));
#68570=CARTESIAN_POINT('Ctrl Pts',(-5.02304719199465,1.21286863387634,80.613702212586));
#68571=CARTESIAN_POINT('Ctrl Pts',(-3.74339168884474,-3.56217238212488,
80.7724629748319));
#68572=CARTESIAN_POINT('Ctrl Pts',(0.962330231331446,-5.07700442602626,
80.9312237370778));
#68573=CARTESIAN_POINT('Ctrl Pts',(4.78729812901886,-1.94520694012218,81.0899844993237));
#68574=CARTESIAN_POINT('Ctrl Pts',(4.2307845491307,2.96690335452649,81.2487452615696));
#68575=CARTESIAN_POINT('Ctrl Pts',(-0.19787228117179,5.16361307382143,81.4075060238155));
#68576=CARTESIAN_POINT('Ctrl Pts',(-4.44543035555655,2.63442638343223,81.5662667860614));
#68577=CARTESIAN_POINT('Ctrl Pts',(-4.62439478129263,-2.30586780285272,
81.7250275483072));
#68578=CARTESIAN_POINT('Ctrl Pts',(-0.57097184883837,-5.13576134197884,
81.8837883105532));
#68579=CARTESIAN_POINT('Ctrl Pts',(4.00502195951943,-3.26524922770216,82.0425490727989));
#68580=CARTESIAN_POINT('Ctrl Pts',(4.91549733690694,1.59371871934676,82.2013098350451));
#68581=CARTESIAN_POINT('Ctrl Pts',(1.32715940311121,4.99406661129702,82.3600705972907));
#68582=CARTESIAN_POINT('Ctrl Pts',(-3.47583534999669,3.82369219939626,82.5188313595369));
#68583=CARTESIAN_POINT('Ctrl Pts',(-5.09763942964231,-0.846242118322492,
82.6775921217824));
#68584=CARTESIAN_POINT('Ctrl Pts',(-2.05392817541576,-4.74166978382725,
82.8363528840287));
#68585=CARTESIAN_POINT('Ctrl Pts',(2.86960084768762,-4.29737645901297,82.9951136462743));
#68586=CARTESIAN_POINT('Ctrl Pts',(5.16678358952832,0.0800071275065655,
83.1538744085204));
#68587=CARTESIAN_POINT('Ctrl Pts',(2.73516803922529,4.38416562959496,83.312635170766));
#68588=CARTESIAN_POINT('Ctrl Pts',(-2.19975659925683,4.67580205641259,83.4713959330121));
#68589=CARTESIAN_POINT('Ctrl Pts',(-5.1213972808606,0.688001186004659,83.6301566952579));
#68590=CARTESIAN_POINT('Ctrl Pts',(-3.35577782577649,-3.92947855970427,
83.7889174575038));
#68591=CARTESIAN_POINT('Ctrl Pts',(1.4811502559097,-4.9505810809301,83.9476782197498));
#68592=CARTESIAN_POINT('Ctrl Pts',(4.96248771955931,-1.44075755171813,84.1064389819956));
#68593=CARTESIAN_POINT('Ctrl Pts',(3.90199844707087,3.38768549854763,84.2651997442416));
#68594=CARTESIAN_POINT('Ctrl Pts',(-0.729706746127024,5.11562640844579,
84.4239605064874));
#68595=CARTESIAN_POINT('Ctrl Pts',(-4.69358549045032,2.16156849958318,84.5827212687333));
#68596=CARTESIAN_POINT('Ctrl Pts',(-4.36170650562841,-2.77078218706868,
84.7414820309791));
#68597=CARTESIAN_POINT('Ctrl Pts',(-0.0379465312430282,-5.16730640666113,
84.9002427932251));
#68598=CARTESIAN_POINT('Ctrl Pts',(4.32070804489202,-2.83440452778566,85.059003555471));
#68599=CARTESIAN_POINT('Ctrl Pts',(4.72460304963626,2.09234474027741,85.2177643177169));
#68600=CARTESIAN_POINT('Ctrl Pts',(0.805001482004623,5.10466438453535,85.3765250799626));
#68601=CARTESIAN_POINT('Ctrl Pts',(-3.85251988452798,3.44398909312549,85.5352858422087));
#68602=CARTESIAN_POINT('Ctrl Pts',(-4.98187820443228,-1.36671670879964,
85.6940466044544));
#68603=CARTESIAN_POINT('Ctrl Pts',(-1.55593411210757,-4.93043766489916,
85.8528073667005));
#68604=CARTESIAN_POINT('Ctrl Pts',(3.302346542614,-3.9740701687742,86.0115681289462));
#68605=CARTESIAN_POINT('Ctrl Pts',(4.81804045098618,-0.159581013320771,
86.1438687641512));
#68606=CARTESIAN_POINT('Ctrl Pts',(3.70615495334781,2.63929363226931,86.2497092723151));
#68607=CARTESIAN_POINT('Ctrl Pts',(2.57208606313468,3.6093054188893,86.3026295263971));
#68608=CARTESIAN_POINT('Ctrl Pts',(1.91898364244101,3.92834389788417,86.329089653438));
#68609=CARTESIAN_POINT('',(2.16917135428672,4.4405021828327,86.));
#68610=CARTESIAN_POINT('Ctrl Pts',(2.54472701347473,-3.56250531650751,85.9999999999999));
#68611=CARTESIAN_POINT('Ctrl Pts',(2.63513329971733,-3.50700228194743,85.9999999999999));
#68612=CARTESIAN_POINT('Ctrl Pts',(2.72315806304114,-3.44815476600379,86.));
#68613=CARTESIAN_POINT('Ctrl Pts',(2.80858471961567,-3.38601400582831,86.));
#68614=CARTESIAN_POINT('Ctrl Pts',(2.91292188753961,-3.31011742753144,86.));
#68615=CARTESIAN_POINT('Ctrl Pts',(3.01338478767473,-3.22930990203852,85.9999999999999));
#68616=CARTESIAN_POINT('Ctrl Pts',(3.1098984160813,-3.14401909712343,85.9999999999999));
#68617=CARTESIAN_POINT('Ctrl Pts',(3.20859981088314,-3.05679492424881,85.9999999999999));
#68618=CARTESIAN_POINT('Ctrl Pts',(3.30317129552995,-2.96488147836652,85.9999999999999));
#68619=CARTESIAN_POINT('Ctrl Pts',(3.39350543356314,-2.86868861821106,85.9999999999999));
#68620=CARTESIAN_POINT('Ctrl Pts',(3.48531110601377,-2.77092878561846,85.9999999999999));
#68621=CARTESIAN_POINT('Ctrl Pts',(3.57274072745551,-2.66874842101355,86.));
#68622=CARTESIAN_POINT('Ctrl Pts',(3.65564683072142,-2.56253686518592,86.));
#68623=CARTESIAN_POINT('Ctrl Pts',(3.68584784338838,-2.52384614862143,86.));
#68624=CARTESIAN_POINT('Ctrl Pts',(3.71544822227817,-2.48462014936941,86.));
#68625=CARTESIAN_POINT('Ctrl Pts',(3.74443952828415,-2.44487660282335,86.));
#68626=CARTESIAN_POINT('Ctrl Pts',(3.75595083040377,-2.42909601082439,86.));
#68627=CARTESIAN_POINT('Ctrl Pts',(3.76736609971463,-2.41323381819194,86.));
#68628=CARTESIAN_POINT('Ctrl Pts',(3.77868477502221,-2.39729111372332,86.));
#68629=CARTESIAN_POINT('Ctrl Pts',(3.78947724093788,-2.38208959146869,86.));
#68630=CARTESIAN_POINT('Ctrl Pts',(3.80017685936615,-2.36682191965604,86.));
#68631=CARTESIAN_POINT('Ctrl Pts',(3.81078105898287,-2.35149266837476,86.));
#68632=CARTESIAN_POINT('Ctrl Pts',(3.88827217096444,-2.23947282995537,86.));
#68633=CARTESIAN_POINT('Ctrl Pts',(3.96071122105411,-2.12411080348259,86.));
#68634=CARTESIAN_POINT('Ctrl Pts',(4.02800505520053,-2.00585829504273,86.));
#68635=CARTESIAN_POINT('Ctrl Pts',(4.09627718657597,-1.88588666771479,86.));
#68636=CARTESIAN_POINT('Ctrl Pts',(4.15925387587574,-1.76293927819734,86.));
#68637=CARTESIAN_POINT('Ctrl Pts',(4.21680206540741,-1.63744665973299,86.));
#68638=CARTESIAN_POINT('Ctrl Pts',(4.27457311504665,-1.5114680607595,86.));
#68639=CARTESIAN_POINT('Ctrl Pts',(4.32687396830893,-1.38292375176368,86.));
#68640=CARTESIAN_POINT('Ctrl Pts',(4.37352758038542,-1.25221847894515,86.));
#68641=CARTESIAN_POINT('Ctrl Pts',(4.41978765417706,-1.1226157473147,86.));
#68642=CARTESIAN_POINT('Ctrl Pts',(4.46049570285582,-0.990887588742712,
86.));
#68643=CARTESIAN_POINT('Ctrl Pts',(4.49543183958698,-0.857409609773572,
86.));
#68644=CARTESIAN_POINT('Ctrl Pts',(4.5001149290464,-0.839517267492425,86.));
#68645=CARTESIAN_POINT('Ctrl Pts',(4.50469423047283,-0.821593465132248,
86.));
#68646=CARTESIAN_POINT('Ctrl Pts',(4.50916914362169,-0.803639092756939,
86.));
#68647=CARTESIAN_POINT('Ctrl Pts',(4.51380380131252,-0.785043788838134,
86.));
#68648=CARTESIAN_POINT('Ctrl Pts',(4.5183245524103,-0.76642335069997,86.));
#68649=CARTESIAN_POINT('Ctrl Pts',(4.52272974339821,-0.747784414927894,
86.));
#68650=CARTESIAN_POINT('Ctrl Pts',(4.55525927718291,-0.610147728443155,
86.));
#68651=CARTESIAN_POINT('Ctrl Pts',(4.58151477805167,-0.471409643850918,
86.));
#68652=CARTESIAN_POINT('Ctrl Pts',(4.60136007125311,-0.332008493005429,
86.));
#68653=CARTESIAN_POINT('Ctrl Pts',(4.6211606972018,-0.19292110252501,86.));
#68654=CARTESIAN_POINT('Ctrl Pts',(4.63458031267456,-0.0531728409362625,
86.));
#68655=CARTESIAN_POINT('Ctrl Pts',(4.64143733545588,0.0868237683291349,
86.));
#68656=CARTESIAN_POINT('Ctrl Pts',(4.64817665416128,0.224417268832664,86.));
#68657=CARTESIAN_POINT('Ctrl Pts',(4.64857698604029,0.362251427033831,86.));
#68658=CARTESIAN_POINT('Ctrl Pts',(4.64241679650986,0.499945184924937,86.));
#68659=CARTESIAN_POINT('Ctrl Pts',(4.64160900570028,0.518001082655194,86.));
#68660=CARTESIAN_POINT('Ctrl Pts',(4.64068833141729,0.536054571915867,86.));
#68661=CARTESIAN_POINT('Ctrl Pts',(4.63965420661563,0.554104796667351,86.));
#68662=CARTESIAN_POINT('Ctrl Pts',(4.63402930249198,0.65228519372856,86.));
#68663=CARTESIAN_POINT('Ctrl Pts',(4.62504894974127,0.750369112179832,86.));
#68664=CARTESIAN_POINT('Ctrl Pts',(4.61279339604946,0.848217515281527,86.));
#68665=CARTESIAN_POINT('Ctrl Pts',(4.6078781705278,0.887460700883271,86.));
#68666=CARTESIAN_POINT('Ctrl Pts',(4.60243597814028,0.926665987486628,86.));
#68667=CARTESIAN_POINT('Ctrl Pts',(4.59647140132863,0.965824309598894,86.));
#68668=CARTESIAN_POINT('Ctrl Pts',(4.59357119157143,0.984864612281179,86.));
#68669=CARTESIAN_POINT('Ctrl Pts',(4.59054712512505,1.00389559177027,86.));
#68670=CARTESIAN_POINT('Ctrl Pts',(4.58740263898465,1.02289935437782,86.));
#68671=CARTESIAN_POINT('Ctrl Pts',(4.56506277525981,1.15791075145704,86.));
#68672=CARTESIAN_POINT('Ctrl Pts',(4.53662319345842,1.29172741325957,86.));
#68673=CARTESIAN_POINT('Ctrl Pts',(4.50239447214487,1.42398414516775,86.));
#68674=CARTESIAN_POINT('Ctrl Pts',(4.46711335178721,1.56030725329147,86.));
#68675=CARTESIAN_POINT('Ctrl Pts',(4.42568158764605,1.6949737254632,86.));
#68676=CARTESIAN_POINT('Ctrl Pts',(4.3783840316949,1.82758749733868,86.));
#68677=CARTESIAN_POINT('Ctrl Pts',(4.33065091250152,1.96142250957807,86.));
#68678=CARTESIAN_POINT('Ctrl Pts',(4.27694321392572,2.09316762674784,86.));
#68679=CARTESIAN_POINT('Ctrl Pts',(4.21750086301315,2.22240829814259,86.));
#68680=CARTESIAN_POINT('Ctrl Pts',(4.17317829962387,2.31877524464499,86.));
#68681=CARTESIAN_POINT('Ctrl Pts',(4.12566627444568,2.41374969077583,86.));
#68682=CARTESIAN_POINT('Ctrl Pts',(4.07504671027994,2.5071531160556,86.));
#68683=CARTESIAN_POINT('Ctrl Pts',(4.04973692819707,2.55385482869548,86.));
#68684=CARTESIAN_POINT('Ctrl Pts',(4.02365003622111,2.60016367547768,86.));
#68685=CARTESIAN_POINT('Ctrl Pts',(3.99679497172134,2.64605655812716,86.));
#68686=CARTESIAN_POINT('Ctrl Pts',(3.98389889010003,2.66809479826952,86.));
#68687=CARTESIAN_POINT('Ctrl Pts',(3.97082565386207,2.69003710756834,86.));
#68688=CARTESIAN_POINT('Ctrl Pts',(3.95757618483902,2.71188087703549,86.));
#68689=CARTESIAN_POINT('Ctrl Pts',(3.94694273066632,2.72941174722991,86.));
#68690=CARTESIAN_POINT('Ctrl Pts',(3.93620106712467,2.74687039690698,86.));
#68691=CARTESIAN_POINT('Ctrl Pts',(3.92535253208302,2.76425480853107,86.));
#68692=CARTESIAN_POINT('Ctrl Pts',(3.92156948774113,2.770317009536,86.));
#68693=CARTESIAN_POINT('Ctrl Pts',(3.91777342701665,2.77637021666335,86.));
#68694=CARTESIAN_POINT('Ctrl Pts',(3.91396438452183,2.78241437972366,86.));
#68695=CARTESIAN_POINT('Ctrl Pts',(3.83729807392157,2.90406796671591,86.));
#68696=CARTESIAN_POINT('Ctrl Pts',(3.7553768005218,3.02205919675202,86.));
#68697=CARTESIAN_POINT('Ctrl Pts',(3.66851542581977,3.13614597147405,86.));
#68698=CARTESIAN_POINT('Ctrl Pts',(3.58104093093735,3.25103803973578,86.));
#68699=CARTESIAN_POINT('Ctrl Pts',(3.48855596305165,3.36197093402805,86.));
#68700=CARTESIAN_POINT('Ctrl Pts',(3.39133507740585,3.46867352459105,86.));
#68701=CARTESIAN_POINT('Ctrl Pts',(3.34733743007933,3.51696215020099,86.));
#68702=CARTESIAN_POINT('Ctrl Pts',(3.30236924503015,3.56438401262811,86.));
#68703=CARTESIAN_POINT('Ctrl Pts',(3.25645316546651,3.61091188198635,86.));
#68704=CARTESIAN_POINT('Ctrl Pts',(3.23459379362241,3.63306250998163,86.));
#68705=CARTESIAN_POINT('Ctrl Pts',(3.21251956234251,3.65501049805194,86.));
#68706=CARTESIAN_POINT('Ctrl Pts',(3.19023278769809,3.67675278772905,86.));
#68707=CARTESIAN_POINT('Ctrl Pts',(3.1754125274436,3.69121097634916,86.));
#68708=CARTESIAN_POINT('Ctrl Pts',(3.16050000228347,3.70557647179484,86.));
#68709=CARTESIAN_POINT('Ctrl Pts',(3.14550229693264,3.71984252397241,86.));
#68710=CARTESIAN_POINT('Ctrl Pts',(3.03965115782958,3.82052978500174,86.));
#68711=CARTESIAN_POINT('Ctrl Pts',(2.92947196960907,3.91635255577481,86.));
#68712=CARTESIAN_POINT('Ctrl Pts',(2.81526020000344,4.00704611824462,86.));
#68713=CARTESIAN_POINT('Ctrl Pts',(2.7017209514917,4.09720564351275,86.));
#68714=CARTESIAN_POINT('Ctrl Pts',(2.58419598194515,4.18229672829323,86.));
#68715=CARTESIAN_POINT('Ctrl Pts',(2.46293629783775,4.26202671871549,86.));
#68716=CARTESIAN_POINT('Ctrl Pts',(2.3673022580591,4.32490747856343,86.));
#68717=CARTESIAN_POINT('Ctrl Pts',(2.26934437440973,4.38445308888104,86.));
#68718=CARTESIAN_POINT('Ctrl Pts',(2.16917135428672,4.4405021828327,86.));
#68719=CARTESIAN_POINT('Ctrl Pts',(2.17574200330365,4.44486699004439,26.));
#68720=CARTESIAN_POINT('Ctrl Pts',(2.28006508424018,4.38720334283182,26.));
#68721=CARTESIAN_POINT('Ctrl Pts',(2.38197081280219,4.32562977310065,26.));
#68722=CARTESIAN_POINT('Ctrl Pts',(2.48120802246663,4.26013719370393,26.));
#68723=CARTESIAN_POINT('Ctrl Pts',(2.60168389996394,4.18062794511602,26.));
#68724=CARTESIAN_POINT('Ctrl Pts',(2.71822805906223,4.09534340135309,26.));
#68725=CARTESIAN_POINT('Ctrl Pts',(2.83065917997165,4.00470474933307,26.));
#68726=CARTESIAN_POINT('Ctrl Pts',(2.90083958424456,3.94812737831637,26.));
#68727=CARTESIAN_POINT('Ctrl Pts',(2.96941670994451,3.88946302886519,26.));
#68728=CARTESIAN_POINT('Ctrl Pts',(3.03633883105725,3.82880744415046,26.));
#68729=CARTESIAN_POINT('Ctrl Pts',(3.07291548330716,3.79565580173034,26.));
#68730=CARTESIAN_POINT('Ctrl Pts',(3.10899764098955,3.76190925146565,26.));
#68731=CARTESIAN_POINT('Ctrl Pts',(3.14457605294962,3.72758291425312,26.));
#68732=CARTESIAN_POINT('Ctrl Pts',(3.16870678245731,3.70430139288574,26.));
#68733=CARTESIAN_POINT('Ctrl Pts',(3.19260993644808,3.68074881011364,26.));
#68734=CARTESIAN_POINT('Ctrl Pts',(3.21625888633569,3.65695400262287,26.));
#68735=CARTESIAN_POINT('Ctrl Pts',(3.31788256697706,3.55470354630845,26.));
#68736=CARTESIAN_POINT('Ctrl Pts',(3.41488652713577,3.44791753206169,26.));
#68737=CARTESIAN_POINT('Ctrl Pts',(3.50709206651038,3.33701451625688,26.));
#68738=CARTESIAN_POINT('Ctrl Pts',(3.59746145912339,3.2283199817939,26.));
#68739=CARTESIAN_POINT('Ctrl Pts',(3.6832218206498,3.11566998580718,26.));
#68740=CARTESIAN_POINT('Ctrl Pts',(3.76416544626806,2.99943221817338,26.));
#68741=CARTESIAN_POINT('Ctrl Pts',(3.79957828247605,2.94857819483358,26.));
#68742=CARTESIAN_POINT('Ctrl Pts',(3.83406863332226,2.89703717531663,26.));
#68743=CARTESIAN_POINT('Ctrl Pts',(3.86761651871398,2.84483889381663,26.));
#68744=CARTESIAN_POINT('Ctrl Pts',(3.89532327236222,2.80172902535561,26.));
#68745=CARTESIAN_POINT('Ctrl Pts',(3.92238715315105,2.75817083249342,26.));
#68746=CARTESIAN_POINT('Ctrl Pts',(3.94879604378199,2.71418084548941,26.));
#68747=CARTESIAN_POINT('Ctrl Pts',(3.95941005243527,2.69650081079038,26.));
#68748=CARTESIAN_POINT('Ctrl Pts',(3.96991386666906,2.6787582983834,26.));
#68749=CARTESIAN_POINT('Ctrl Pts',(3.98030512442337,2.6609577203422,26.));
#68750=CARTESIAN_POINT('Ctrl Pts',(4.05292301831336,2.53656079766556,26.));
#68751=CARTESIAN_POINT('Ctrl Pts',(4.12007774857859,2.40928022608588,26.));
#68752=CARTESIAN_POINT('Ctrl Pts',(4.18159035621228,2.27951928558395,26.));
#68753=CARTESIAN_POINT('Ctrl Pts',(4.24297458767659,2.15002915480893,26.));
#68754=CARTESIAN_POINT('Ctrl Pts',(4.29874053362767,2.01806821927191,26.));
#68755=CARTESIAN_POINT('Ctrl Pts',(4.34866300062458,1.88401668144009,26.));
#68756=CARTESIAN_POINT('Ctrl Pts',(4.39830723531613,1.75071225148679,26.));
#68757=CARTESIAN_POINT('Ctrl Pts',(4.44217322437405,1.61533971306916,26.));
#68758=CARTESIAN_POINT('Ctrl Pts',(4.47998827572883,1.47826395773052,26.));
#68759=CARTESIAN_POINT('Ctrl Pts',(4.50834956424491,1.37545714122654,26.));
#68760=CARTESIAN_POINT('Ctrl Pts',(4.53330618455047,1.27169201598405,26.));
#68761=CARTESIAN_POINT('Ctrl Pts',(4.55472254010161,1.16712293514026,26.));
#68762=CARTESIAN_POINT('Ctrl Pts',(4.5633703360405,1.12489856739035,26.));
#68763=CARTESIAN_POINT('Ctrl Pts',(4.57144068485198,1.0825431363053,26.));
#68764=CARTESIAN_POINT('Ctrl Pts',(4.57892379357549,1.04006693008015,26.));
#68765=CARTESIAN_POINT('Ctrl Pts',(4.58238261217842,1.02043371376567,26.));
#68766=CARTESIAN_POINT('Ctrl Pts',(4.58571635833316,1.00077225530923,26.));
#68767=CARTESIAN_POINT('Ctrl Pts',(4.58892275403614,0.98109144089082,26.));
#68768=CARTESIAN_POINT('Ctrl Pts',(4.6112579051569,0.843998578707096,26.));
#68769=CARTESIAN_POINT('Ctrl Pts',(4.62736483254579,0.706302385469903,26.));
#68770=CARTESIAN_POINT('Ctrl Pts',(4.63704039371253,0.568349643633761,26.));
#68771=CARTESIAN_POINT('Ctrl Pts',(4.64529719664733,0.450625350021645,26.));
#68772=CARTESIAN_POINT('Ctrl Pts',(4.64886975587046,0.332713782967315,26.));
#68773=CARTESIAN_POINT('Ctrl Pts',(4.64760179618238,0.214828774577272,26.));
#68774=CARTESIAN_POINT('Ctrl Pts',(4.64610810169851,0.0759567044171535,
26.));
#68775=CARTESIAN_POINT('Ctrl Pts',(4.63789790766952,-0.0628793196366818,
26.));
#68776=CARTESIAN_POINT('Ctrl Pts',(4.62316922884463,-0.20123695388626,26.));
#68777=CARTESIAN_POINT('Ctrl Pts',(4.60840903270106,-0.339890654178337,
26.));
#68778=CARTESIAN_POINT('Ctrl Pts',(4.58710205140909,-0.478064733297057,
26.));
#68779=CARTESIAN_POINT('Ctrl Pts',(4.55939920087044,-0.615294818730504,
26.));
#68780=CARTESIAN_POINT('Ctrl Pts',(4.54980593455313,-0.66281645389487,26.));
#68781=CARTESIAN_POINT('Ctrl Pts',(4.53944529005038,-0.710224661945217,
26.));
#68782=CARTESIAN_POINT('Ctrl Pts',(4.52832231101321,-0.757499347947085,
26.));
#68783=CARTESIAN_POINT('Ctrl Pts',(4.52204558440698,-0.784176578789409,
26.));
#68784=CARTESIAN_POINT('Ctrl Pts',(4.51552434543633,-0.81081776400017,26.));
#68785=CARTESIAN_POINT('Ctrl Pts',(4.50876854798769,-0.837384466189193,
26.));
#68786=CARTESIAN_POINT('Ctrl Pts',(4.47488762719443,-0.97061882370914,26.));
#68787=CARTESIAN_POINT('Ctrl Pts',(4.43508456291388,-1.10210853291686,26.));
#68788=CARTESIAN_POINT('Ctrl Pts',(4.38958618794437,-1.2314396670372,26.));
#68789=CARTESIAN_POINT('Ctrl Pts',(4.34401166128567,-1.36098726568698,26.));
#68790=CARTESIAN_POINT('Ctrl Pts',(4.29272234355304,-1.48836984485114,26.));
#68791=CARTESIAN_POINT('Ctrl Pts',(4.23589771868779,-1.61315285151403,26.));
#68792=CARTESIAN_POINT('Ctrl Pts',(4.18015009153959,-1.73557084452973,26.));
#68793=CARTESIAN_POINT('Ctrl Pts',(4.11907449353476,-1.85548750502406,26.));
#68794=CARTESIAN_POINT('Ctrl Pts',(4.05280063784894,-1.97246430242313,26.));
#68795=CARTESIAN_POINT('Ctrl Pts',(4.0071971296468,-2.0529568629426,26.));
#68796=CARTESIAN_POINT('Ctrl Pts',(3.95913143391569,-2.13205676654158,26.));
#68797=CARTESIAN_POINT('Ctrl Pts',(3.90866288715487,-2.2096607611529,26.));
#68798=CARTESIAN_POINT('Ctrl Pts',(3.88457170018092,-2.24670506823327,26.));
#68799=CARTESIAN_POINT('Ctrl Pts',(3.85993289144,-2.28340838898037,26.));
#68800=CARTESIAN_POINT('Ctrl Pts',(3.83475240364166,-2.31975877789511,26.));
#68801=CARTESIAN_POINT('Ctrl Pts',(3.81911152043036,-2.34233785548306,26.));
#68802=CARTESIAN_POINT('Ctrl Pts',(3.80326163575805,-2.36478075250477,26.));
#68803=CARTESIAN_POINT('Ctrl Pts',(3.78720411571068,-2.38708450953735,26.));
#68804=CARTESIAN_POINT('Ctrl Pts',(3.77570997324099,-2.40304977442168,26.));
#68805=CARTESIAN_POINT('Ctrl Pts',(3.76411377204687,-2.41893767166227,26.));
#68806=CARTESIAN_POINT('Ctrl Pts',(3.75242084457745,-2.43474120045983,26.));
#68807=CARTESIAN_POINT('Ctrl Pts',(3.66959100122522,-2.54668954001269,26.));
#68808=CARTESIAN_POINT('Ctrl Pts',(3.58184107407233,-2.65450498805187,26.));
#68809=CARTESIAN_POINT('Ctrl Pts',(3.48944434360053,-2.75789800803035,26.));
#68810=CARTESIAN_POINT('Ctrl Pts',(3.40008035358429,-2.85789735603679,26.));
#68811=CARTESIAN_POINT('Ctrl Pts',(3.3063688476751,-2.95376016129811,26.));
#68812=CARTESIAN_POINT('Ctrl Pts',(3.20852006341883,-3.04518760514634,26.));
#68813=CARTESIAN_POINT('Ctrl Pts',(3.11161693078311,-3.13573145589637,26.));
#68814=CARTESIAN_POINT('Ctrl Pts',(3.01065557724222,-3.2219256920299,26.));
#68815=CARTESIAN_POINT('Ctrl Pts',(2.90581240538358,-3.30343749134566,26.));
#68816=CARTESIAN_POINT('Ctrl Pts',(2.80309976478498,-3.38329287915244,26.));
#68817=CARTESIAN_POINT('Ctrl Pts',(2.69666097167601,-3.45865450573126,26.));
#68818=CARTESIAN_POINT('Ctrl Pts',(2.58664264704464,-3.52916309203659,26.));
#68819=CARTESIAN_POINT('Ctrl Pts',(2.57062378681069,-3.53942926535911,26.));
#68820=CARTESIAN_POINT('Ctrl Pts',(2.55452901448013,-3.54959246856517,26.));
#68821=CARTESIAN_POINT('Ctrl Pts',(2.53835875722658,-3.55965150255066,26.));
#68822=CARTESIAN_POINT('Ctrl Pts',(2.16917135428672,4.4405021828327,86.));
#68823=CARTESIAN_POINT('Ctrl Pts',(2.90742207776984,4.07986902565238,85.973539872959));
#68824=CARTESIAN_POINT('Ctrl Pts',(3.54838370350565,3.53163043353487,85.947079745918));
#68825=CARTESIAN_POINT('Ctrl Pts',(4.02597047844268,2.86203885652618,85.9206196188771));
#68826=CARTESIAN_POINT('Ctrl Pts',(4.50355725337971,2.19244727951748,85.894159491836));
#68827=CARTESIAN_POINT('Ctrl Pts',(4.817769177518,1.40150271761755,85.8676993647951));
#68828=CARTESIAN_POINT('Ctrl Pts',(4.91302361527573,0.586752768661848,85.8412392377541));
#68829=CARTESIAN_POINT('Ctrl Pts',(5.10353249079119,-1.04274712924955,85.7883189836721));
#68830=CARTESIAN_POINT('Ctrl Pts',(4.41821142078444,-2.76746857538425,85.7353987295902));
#68831=CARTESIAN_POINT('Ctrl Pts',(3.16027096066549,-3.81000496808603,85.6824784755082));
#68832=CARTESIAN_POINT('Ctrl Pts',(1.90233050054647,-4.85254136078787,85.6295582214263));
#68833=CARTESIAN_POINT('Ctrl Pts',(0.071770650315324,-5.21289270005682,
85.5766379673442));
#68834=CARTESIAN_POINT('Ctrl Pts',(-1.4889429323282,-4.72167812247258,85.5237177132623));
#68835=CARTESIAN_POINT('Ctrl Pts',(-3.04965651497173,-4.23046354488835,
85.4707974591803));
#68836=CARTESIAN_POINT('Ctrl Pts',(-4.34052383002751,-2.88768305045078,
85.4178772050984));
#68837=CARTESIAN_POINT('Ctrl Pts',(-4.77319106421879,-1.30997578306141,
85.3649569510165));
#68838=CARTESIAN_POINT('Ctrl Pts',(-4.88938737554012,-0.886269640491669,
85.3507447855632));
#68839=CARTESIAN_POINT('Ctrl Pts',(-4.94368731125384,-0.445619761719663,
85.33653262011));
#68840=CARTESIAN_POINT('Ctrl Pts',(-4.93983901057914,-0.00407131671605609,
85.3223204546568));
#68841=CARTESIAN_POINT('Origin',(0.,0.,16.));
#68842=CARTESIAN_POINT('Origin',(0.,0.,86.));
#68843=CARTESIAN_POINT('Origin',(0.,0.,26.));
#68844=CARTESIAN_POINT('',(4.61880215351701,-8.,26.));
#68845=CARTESIAN_POINT('',(9.23760430703401,0.,26.));
#68846=CARTESIAN_POINT('',(4.61880215351701,-8.,26.));
#68847=CARTESIAN_POINT('',(4.61880215351701,8.,26.));
#68848=CARTESIAN_POINT('',(9.23760430703401,0.,26.));
#68849=CARTESIAN_POINT('',(-4.61880215351701,8.,26.));
#68850=CARTESIAN_POINT('',(4.61880215351701,8.,26.));
#68851=CARTESIAN_POINT('',(-9.23760430703401,1.11022302462516E-15,26.));
#68852=CARTESIAN_POINT('',(-4.618802153517,8.,26.));
#68853=CARTESIAN_POINT('',(-4.61880215351701,-8.,26.));
#68854=CARTESIAN_POINT('',(-9.23760430703401,1.1312802546399E-15,26.));
#68855=CARTESIAN_POINT('',(-4.61880215351701,-8.,26.));
#68856=CARTESIAN_POINT('Origin',(0.,0.,20.));
#68857=CARTESIAN_POINT('',(4.61880215351701,-8.,20.));
#68858=CARTESIAN_POINT('',(9.23760430703401,0.,20.));
#68859=CARTESIAN_POINT('',(4.61880215351701,-8.,20.));
#68860=CARTESIAN_POINT('',(-4.61880215351701,-8.,20.));
#68861=CARTESIAN_POINT('',(-4.61880215351701,-8.,20.));
#68862=CARTESIAN_POINT('',(-9.23760430703401,1.1312802546399E-15,20.));
#68863=CARTESIAN_POINT('',(-9.23760430703401,1.1312802546399E-15,20.));
#68864=CARTESIAN_POINT('',(-4.618802153517,8.,20.));
#68865=CARTESIAN_POINT('',(-4.618802153517,8.,20.));
#68866=CARTESIAN_POINT('',(4.61880215351701,8.,20.));
#68867=CARTESIAN_POINT('',(4.61880215351701,8.,20.));
#68868=CARTESIAN_POINT('',(9.23760430703401,0.,20.));
#68869=CARTESIAN_POINT('',(-5.,6.12323399573677E-16,20.));
#68870=CARTESIAN_POINT('Origin',(0.,0.,20.));
#68871=CARTESIAN_POINT('Origin',(-4.61880215351701,-8.,20.));
#68872=CARTESIAN_POINT('',(4.61880215351701,-8.,20.));
#68873=CARTESIAN_POINT('',(-4.61880215351701,-8.,20.));
#68874=CARTESIAN_POINT('Origin',(-9.23760430703401,1.1312802546399E-15,
20.));
#68875=CARTESIAN_POINT('',(-9.23760430703401,1.1312802546399E-15,20.));
#68876=CARTESIAN_POINT('Origin',(-4.618802153517,8.,20.));
#68877=CARTESIAN_POINT('',(-4.618802153517,8.,20.));
#68878=CARTESIAN_POINT('Origin',(4.61880215351701,8.,20.));
#68879=CARTESIAN_POINT('',(4.61880215351701,8.,20.));
#68880=CARTESIAN_POINT('Origin',(9.23760430703401,0.,20.));
#68881=CARTESIAN_POINT('',(9.23760430703401,0.,20.));
#68882=CARTESIAN_POINT('Origin',(4.61880215351701,-8.,20.));
#68883=CARTESIAN_POINT('Origin',(0.,0.,16.));
#68884=CARTESIAN_POINT('',(-5.,6.12323399573677E-16,17.3166247903554));
#68885=CARTESIAN_POINT('',(-5.,-6.12323399573677E-16,16.));
#68886=CARTESIAN_POINT('Origin',(0.,0.,17.3166247903554));
#68887=CARTESIAN_POINT('Origin',(0.,0.,86.));
#68888=CARTESIAN_POINT('Origin',(5.55111512312578E-16,0.,14.));
#68889=CARTESIAN_POINT('',(1.87717472568372E-16,-4.49927934798557E-32,8.));
#68890=CARTESIAN_POINT('Origin',(5.55111512312578E-16,0.,14.));
#97444=UNCERTAINTY_MEASURE_WITH_UNIT(LENGTH_MEASURE(0.01),#97476,
'DISTANCE_ACCURACY_VALUE',
'Maximum model space distance between geometric entities at asserted c
onnectivities');
#97452=UNCERTAINTY_MEASURE_WITH_UNIT(LENGTH_MEASURE(0.01),#97476,
'DISTANCE_ACCURACY_VALUE',
'Maximum model space distance between geometric entities at asserted c
onnectivities');
#97467=(
GEOMETRIC_REPRESENTATION_CONTEXT(3)
GLOBAL_UNCERTAINTY_ASSIGNED_CONTEXT((#97444))
GLOBAL_UNIT_ASSIGNED_CONTEXT((#97476,#97478,#97479))
REPRESENTATION_CONTEXT('','3D')
);
#97475=(
GEOMETRIC_REPRESENTATION_CONTEXT(3)
GLOBAL_UNCERTAINTY_ASSIGNED_CONTEXT((#97452))
GLOBAL_UNIT_ASSIGNED_CONTEXT((#97476,#97478,#97479))
REPRESENTATION_CONTEXT('','3D')
);
#97476=(
LENGTH_UNIT()
NAMED_UNIT(*)
SI_UNIT(.MILLI.,.METRE.)
);
#97478=(
NAMED_UNIT(*)
PLANE_ANGLE_UNIT()
SI_UNIT($,.RADIAN.)
);
#97479=(
NAMED_UNIT(*)
SI_UNIT($,.STERADIAN.)
SOLID_ANGLE_UNIT()
);
#97494=SHAPE_DEFINITION_REPRESENTATION(#97556,#97617);
#97556=PRODUCT_DEFINITION_SHAPE('',$,#97640);
#97617=SHAPE_REPRESENTATION('',(#22809),#97467);
#97625=PRODUCT_DEFINITION_CONTEXT('part definition',#97693,'design');
#97640=PRODUCT_DEFINITION('Adjusting spindle','Adjusting spindle',#97662,
#97625);
#97662=PRODUCT_DEFINITION_FORMATION('',$,#97709);
#97693=APPLICATION_CONTEXT(
'Core Data for Automotive Mechanical Design Process');
#97694=PRODUCT_CONTEXT('part definition',#97693,'mechanical');
#97709=PRODUCT('Adjusting spindle','Adjusting spindle',$,(#97694));
#97723=PRESENTATION_STYLE_ASSIGNMENT((#97730));
#97730=SURFACE_STYLE_USAGE(.BOTH.,#97737);
#97737=SURFACE_SIDE_STYLE('',(#97744));
#97744=SURFACE_STYLE_FILL_AREA(#97751);
#97751=FILL_AREA_STYLE('Light blue',(#97758));
#97758=FILL_AREA_STYLE_COLOUR('Light blue',#97765);
#97765=COLOUR_RGB('Light blue',0.662745098039216,0.831372549019608,0.949019607843137);
ENDSEC;
END-ISO-10303-21;
